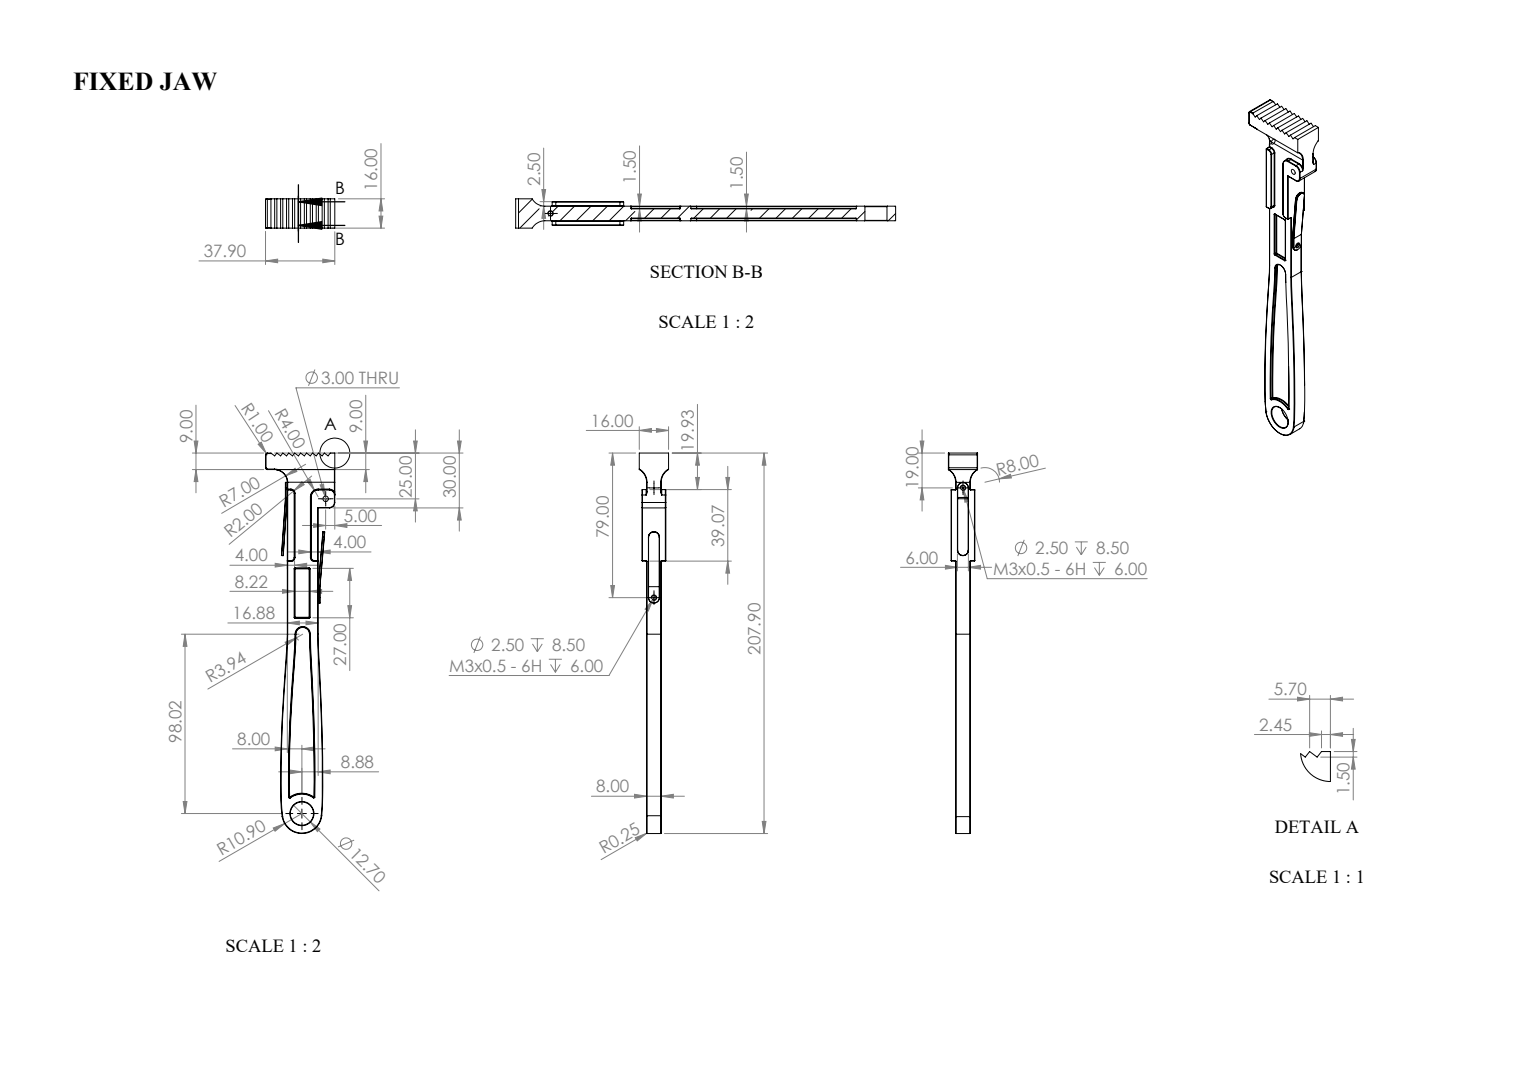
ISO-10303-21;
HEADER;
FILE_DESCRIPTION (('STEP AP214'),
    '1' );
FILE_NAME ('1.0 Fixed Jaw.step',
    '2026-10-07T05:30:18',
    ( '' ),
    ( '' ),
    'SwSTEP 2.0',
    'SolidWorks 2021',
    '' );
FILE_SCHEMA (( 'AUTOMOTIVE_DESIGN' ));
ENDSEC;

DATA;
#30=AXIS2_PLACEMENT_3D ( 'NONE', #64343, #43811, #52312 ) ;
#52=LINE ( 'NONE', #39009, #8257 ) ;
#64=EDGE_CURVE ( 'NONE', #6847, #38896, #39743, .T. ) ;
#74=SURFACE_SIDE_STYLE ('',( #68542 ) ) ;
#87=CARTESIAN_POINT ( 'NONE',  ( -6.000000000000014211, 80.32179676972448590, -4.250000000000000000 ) ) ;
#88=( GEOMETRIC_REPRESENTATION_CONTEXT ( 3 ) GLOBAL_UNCERTAINTY_ASSIGNED_CONTEXT ( ( #83266 ) ) GLOBAL_UNIT_ASSIGNED_CONTEXT ( ( #85236, #77227, #46251 ) ) REPRESENTATION_CONTEXT ( 'NONE', 'WORKASPACE' ) );
#90=EDGE_LOOP ( 'NONE', ( #14273, #19404, #8393, #55652 ) ) ;
#99=DIRECTION ( 'NONE',  ( -0.000000000000000000, -0.000000000000000000, -1.000000000000000000 ) ) ;
#104=CARTESIAN_POINT ( 'NONE',  ( 11.15633734009358058, -69.21829398631774666, 4.000000000000000888 ) ) ;
#105=VERTEX_POINT ( 'NONE', #92727 ) ;
#109=FILL_AREA_STYLE_COLOUR ( '', #46180 ) ;
#111=DIRECTION ( 'NONE',  ( 1.000000000000000000, -0.000000000000000000, -0.000000000000000000 ) ) ;
#123=FILL_AREA_STYLE ('',( #74603 ) ) ;
#124=STYLED_ITEM ( 'NONE', ( #39195 ), #78361 ) ;
#133=CARTESIAN_POINT ( 'NONE',  ( -5.812563760649267941, -35.09659463721938977, -3.750000000000000000 ) ) ;
#148=CIRCLE ( 'NONE', #91104, 1.249999999999987121 ) ;
#175=CARTESIAN_POINT ( 'NONE',  ( -11.62817260212919024, -77.84151128241038009, 3.750000000000000000 ) ) ;
#185=ORIENTED_EDGE ( 'NONE', *, *, #34928, .T. ) ;
#195=DIRECTION ( 'NONE',  ( -1.483861936729427615E-16, 1.000000000000000000, -0.000000000000000000 ) ) ;
#196=DIRECTION ( 'NONE',  ( 0.000000000000000000, 0.000000000000000000, 1.000000000000000000 ) ) ;
#199=ORIENTED_EDGE ( 'NONE', *, *, #97123, .F. ) ;
#201=ORIENTED_EDGE ( 'NONE', *, *, #76299, .T. ) ;
#210=CARTESIAN_POINT ( 'NONE',  ( -6.874984555098656358, -78.81798443069058635, 2.499999999999998224 ) ) ;
#225=STYLED_ITEM ( 'NONE', ( #36779 ), #46100 ) ;
#228=ORIENTED_EDGE ( 'NONE', *, *, #21710, .F. ) ;
#250=SURFACE_STYLE_USAGE ( .BOTH. , #76223 ) ;
#258=FACE_OUTER_BOUND ( 'NONE', #51924, .T. ) ;
#268=AXIS2_PLACEMENT_3D ( 'NONE', #55440, #85944, #96401 ) ;
#274=DIRECTION ( 'NONE',  ( -1.000000000000000000, -0.000000000000000000, -0.000000000000000000 ) ) ;
#281=CARTESIAN_POINT ( 'NONE',  ( 11.13643110622481203, -94.02619357113461263, -3.750000000000000000 ) ) ;
#286=LINE ( 'NONE', #30732, #94331 ) ;
#293=UNCERTAINTY_MEASURE_WITH_UNIT (LENGTH_MEASURE( 1.000000000000000082E-05 ), #85346, 'distance_accuracy_value', 'NONE');
#298=DIRECTION ( 'NONE',  ( 0.000000000000000000, 0.000000000000000000, -1.000000000000000000 ) ) ;
#308=VECTOR ( 'NONE', #84981, 1000.000000000000000 ) ;
#309=( NAMED_UNIT ( * ) SI_UNIT ( $, .STERADIAN. ) SOLID_ANGLE_UNIT ( ) );
#313=ORIENTED_EDGE ( 'NONE', *, *, #41696, .F. ) ;
#328=ORIENTED_EDGE ( 'NONE', *, *, #58687, .T. ) ;
#329=DIRECTION ( 'NONE',  ( 0.000000000000000000, 0.000000000000000000, 1.000000000000000000 ) ) ;
#340=VECTOR ( 'NONE', #77735, 1000.000000000000000 ) ;
#351=CARTESIAN_POINT ( 'NONE',  ( 6.574926501674518420, -50.89417846498341902, -3.750000000000001332 ) ) ;
#365=CARTESIAN_POINT ( 'NONE',  ( 4.864310448982641866, -17.52237222630224878, -2.499999999999999112 ) ) ;
#369=CIRCLE ( 'NONE', #57769, 0.2500000000000002220 ) ;
#384=CARTESIAN_POINT ( 'NONE',  ( -8.330963135173325540, -7.272696214946840598, -3.750000000000000000 ) ) ;
#391=CARTESIAN_POINT ( 'NONE',  ( 9.050000000000002487, 99.99999999999998579, 8.000000000000000000 ) ) ;
#398=EDGE_LOOP ( 'NONE', ( #49399, #35064, #25132, #40932 ) ) ;
#400=CARTESIAN_POINT ( 'NONE',  ( -8.081452932468565109, -7.288464344191233124, -3.999999999999999112 ) ) ;
#406=CARTESIAN_POINT ( 'NONE',  ( -18.89999999999999147, 99.74999999999998579, 7.750000000000000000 ) ) ;
#427=EDGE_CURVE ( 'NONE', #16059, #54251, #3743, .T. ) ;
#445=ORIENTED_EDGE ( 'NONE', *, *, #14494, .F. ) ;
#451=CARTESIAN_POINT ( 'NONE',  ( -6.000000000000014211, 79.82179676972448590, 6.500000000000000888 ) ) ;
#464=ORIENTED_EDGE ( 'NONE', *, *, #87707, .F. ) ;
#475=CARTESIAN_POINT ( 'NONE',  ( -0.6999999999999975131, 99.99999999999998579, -8.000000000000000000 ) ) ;
#477=EDGE_LOOP ( 'NONE', ( #2774, #88083, #69231, #10665 ) ) ;
#493=CARTESIAN_POINT ( 'NONE',  ( 6.033511671501928575, -36.04540650299031768, 2.750000000000000444 ) ) ;
#528=ORIENTED_EDGE ( 'NONE', *, *, #21195, .F. ) ;
#538=VERTEX_POINT ( 'NONE', #32791 ) ;
#539=LINE ( 'NONE', #73152, #10187 ) ;
#540=LINE ( 'NONE', #46011, #12696 ) ;
#548=PLANE ( 'NONE',  #17195 ) ;
#554=CARTESIAN_POINT ( 'NONE',  ( -5.580560104534955101, -28.67655754327235584, -4.000000000000000000 ) ) ;
#556=ORIENTED_EDGE ( 'NONE', *, *, #48860, .F. ) ;
#581=AXIS2_PLACEMENT_3D ( 'NONE', #82369, #74368, #90856 ) ;
#595=( GEOMETRIC_REPRESENTATION_CONTEXT ( 3 ) GLOBAL_UNCERTAINTY_ASSIGNED_CONTEXT ( ( #30226 ) ) GLOBAL_UNIT_ASSIGNED_CONTEXT ( ( #63751, #69807, #85295 ) ) REPRESENTATION_CONTEXT ( 'NONE', 'WORKASPACE' ) );
#598=LINE ( 'NONE', #86029, #77826 ) ;
#599=EDGE_CURVE ( 'NONE', #79717, #54884, #31804, .T. ) ;
#601=CARTESIAN_POINT ( 'NONE',  ( 11.08989791451569396, -87.81815274841501662, 4.000000000000000888 ) ) ;
#620=EDGE_CURVE ( 'NONE', #27580, #78252, #34744, .T. ) ;
#654=CYLINDRICAL_SURFACE ( 'NONE', #4662, 2.999999999999999112 ) ;
#655=EDGE_CURVE ( 'NONE', #6373, #42611, #90428, .T. ) ;
#661=FACE_OUTER_BOUND ( 'NONE', #43555, .T. ) ;
#664=ORIENTED_EDGE ( 'NONE', *, *, #80208, .F. ) ;
#669=CARTESIAN_POINT ( 'NONE',  ( -11.60563658634833040, -81.99692803277896758, 4.000000000000001776 ) ) ;
#679=ORIENTED_EDGE ( 'NONE', *, *, #13478, .F. ) ;
#688=CARTESIAN_POINT ( 'NONE',  ( -3.999999999999994671, 43.00000000000000711, 6.500000000000000888 ) ) ;
#692=ORIENTED_EDGE ( 'NONE', *, *, #60606, .T. ) ;
#694=ORIENTED_EDGE ( 'NONE', *, *, #84783, .T. ) ;
#707=AXIS2_PLACEMENT_3D ( 'NONE', #2561, #55539, #79512 ) ;
#710=DIRECTION ( 'NONE',  ( 0.000000000000000000, -0.000000000000000000, -1.000000000000000000 ) ) ;
#715=DIRECTION ( 'NONE',  ( -0.000000000000000000, -0.000000000000000000, 1.000000000000000000 ) ) ;
#717=VERTEX_POINT ( 'NONE', #42770 ) ;
#730=CARTESIAN_POINT ( 'NONE',  ( 6.034042420210333546, -36.05779855178114701, -2.750000000000001332 ) ) ;
#734=EDGE_CURVE ( 'NONE', #717, #9323, #56198, .T. ) ;
#739=DIRECTION ( 'NONE',  ( 0.000000000000000000, 0.000000000000000000, -1.000000000000000000 ) ) ;
#750=CIRCLE ( 'NONE', #66369, 0.1000000000000001166 ) ;
#761=DIRECTION ( 'NONE',  ( 0.000000000000000000, 0.000000000000000000, -1.000000000000000000 ) ) ;
#767=CARTESIAN_POINT ( 'NONE',  ( 10.68823582872827060, -97.11172657260387098, -4.000000000000000000 ) ) ;
#774=PRESENTATION_STYLE_ASSIGNMENT (( #85725 ) ) ;
#776=ADVANCED_FACE ( 'NONE', ( #13253 ), #4285, .T. ) ;
#780=ORIENTED_EDGE ( 'NONE', *, *, #20104, .T. ) ;
#782=DIRECTION ( 'NONE',  ( -0.000000000000000000, 1.000000000000000000, 0.000000000000000000 ) ) ;
#794=CARTESIAN_POINT ( 'NONE',  ( -3.772059543480554389, -0.8421633283343330501, 3.999999999999999112 ) ) ;
#809=ORIENTED_EDGE ( 'NONE', *, *, #74543, .T. ) ;
#814=( LENGTH_UNIT ( ) NAMED_UNIT ( * ) SI_UNIT ( .MILLI., .METRE. ) );
#818=ADVANCED_FACE ( 'NONE', ( #258 ), #67246, .F. ) ;
#823=CARTESIAN_POINT ( 'NONE',  ( -8.000000000000000000, 80.99999999999994316, -1.249999999999987121 ) ) ;
#826=DIRECTION ( 'NONE',  ( 0.6246950475544238435, 0.7808688094430307203, 0.000000000000000000 ) ) ;
#832=CARTESIAN_POINT ( 'NONE',  ( -7.116236337400218659, -80.68324593764592123, -2.750000000000000000 ) ) ;
#835=( NAMED_UNIT ( * ) SI_UNIT ( $, .STERADIAN. ) SOLID_ANGLE_UNIT ( ) );
#843=CARTESIAN_POINT ( 'NONE',  ( 6.685134130357478277, -80.57704203013921074, -2.500000000000000888 ) ) ;
#846=COLOUR_RGB ( '', 0.40784314, 0.44705882, 0.49803922) ;
#847=CARTESIAN_POINT ( 'NONE',  ( 4.471352795670365587, -3.620003340340034015, 2.750000000000000000 ) ) ;
#861=FILL_AREA_STYLE ('',( #14877 ) ) ;
#868=CYLINDRICAL_SURFACE ( 'NONE', #65920, 0.2500000000000002220 ) ;
#869=DIRECTION ( 'NONE',  ( 0.000000000000000000, 0.000000000000000000, -1.000000000000000000 ) ) ;
#875=VERTEX_POINT ( 'NONE', #9203 ) ;
#876=SURFACE_STYLE_FILL_AREA ( #39838 ) ;
#894=AXIS2_PLACEMENT_3D ( 'NONE', #5161, #50153, #35647 ) ;
#896=CARTESIAN_POINT ( 'NONE',  ( -3.750000000000000000, 37.00000000000000000, 2.500000000000000000 ) ) ;
#905=ORIENTED_EDGE ( 'NONE', *, *, #91110, .F. ) ;
#910=VECTOR ( 'NONE', #54975, 1000.000000000000000 ) ;
#913=CARTESIAN_POINT ( 'NONE',  ( 7.155633850256548634, -69.45312897839663435, 4.000000000000000000 ) ) ;
#917=DIRECTION ( 'NONE',  ( -1.000000000000000000, 0.000000000000000000, 0.000000000000000000 ) ) ;
#918=CARTESIAN_POINT ( 'NONE',  ( -6.060849023604187202, -36.09672517615241816, -3.999999999999998224 ) ) ;
#942=EDGE_CURVE ( 'NONE', #49230, #87437, #86679, .T. ) ;
#944=SURFACE_STYLE_USAGE ( .BOTH. , #70415 ) ;
#946=AXIS2_PLACEMENT_3D ( 'NONE', #32170, #55169, #47682 ) ;
#947=DIRECTION ( 'NONE',  ( 0.000000000000000000, 0.000000000000000000, -1.000000000000000000 ) ) ;
#950=CARTESIAN_POINT ( 'NONE',  ( 4.691427381388422191, -2.693150427207434028, -4.000000000000000000 ) ) ;
#955=AXIS2_PLACEMENT_3D ( 'NONE', #88798, #94817, #26320 ) ;
#965=CARTESIAN_POINT ( 'NONE',  ( -13.22845221182699404, 91.00000000000001421, -8.000000000000001776 ) ) ;
#967=CARTESIAN_POINT ( 'NONE',  ( 4.572805492043258369, -6.390838093377243290, 2.750000000000000000 ) ) ;
#970=DIRECTION ( 'NONE',  ( 0.000000000000000000, 0.000000000000000000, -1.000000000000000000 ) ) ;
#976=AXIS2_PLACEMENT_3D ( 'NONE', #83405, #29399, #14927 ) ;
#981=VERTEX_POINT ( 'NONE', #79166 ) ;
#989=CARTESIAN_POINT ( 'NONE',  ( 18.00000000000000711, 77.36170532436575797, 4.193342410628620343 ) ) ;
#991=SURFACE_STYLE_FILL_AREA ( #92941 ) ;
#1003=EDGE_CURVE ( 'NONE', #3599, #65307, #65631, .T. ) ;
#1019=DIRECTION ( 'NONE',  ( 0.000000000000000000, 0.000000000000000000, 1.000000000000000000 ) ) ;
#1028=ORIENTED_EDGE ( 'NONE', *, *, #35765, .F. ) ;
#1050=STYLED_ITEM ( 'NONE', ( #3795 ), #35208 ) ;
#1051=EDGE_CURVE ( 'NONE', #67870, #46091, #81134, .T. ) ;
#1054=AXIS2_PLACEMENT_3D ( 'NONE', #1684, #85651, #92650 ) ;
#1056=EDGE_CURVE ( 'NONE', #28374, #28519, #71675, .T. ) ;
#1060=ORIENTED_EDGE ( 'NONE', *, *, #71039, .T. ) ;
#1066=CARTESIAN_POINT ( 'NONE',  ( 8.629999999999995453, 40.74999999999999289, -3.750000000000000000 ) ) ;
#1069=CARTESIAN_POINT ( 'NONE',  ( 4.879999999999991900, 76.07179676972444327, 6.250000000000000000 ) ) ;
#1080=DIRECTION ( 'NONE',  ( 1.000000000000000000, 0.000000000000000000, 0.000000000000000000 ) ) ;
#1088=( NAMED_UNIT ( * ) PLANE_ANGLE_UNIT ( ) SI_UNIT ( $, .RADIAN. ) );
#1096=DIRECTION ( 'NONE',  ( 0.000000000000000000, 0.000000000000000000, 1.000000000000000000 ) ) ;
#1107=CARTESIAN_POINT ( 'NONE',  ( -0.000000000000000000, 99.99999999999998579, -8.000000000000000000 ) ) ;
#1113=( BOUNDED_SURFACE ( )  B_SPLINE_SURFACE ( 3, 2, ( 
 ( #32802, #48792, #77812 ),
 ( #94787, #11290, #63297 ),
 ( #64765, #79787, #93807 ),
 ( #79300, #24835, #25337 ),
 ( #95277, #55821, #86315 ),
 ( #87283, #17819, #26287 ),
 ( #39830, #48301, #56788 ),
 ( #26780, #57278, #41327 ),
 ( #70336, #1852, #32310 ),
 ( #62815, #93313, #49774 ),
 ( #35263, #97782, #89746 ),
 ( #50260, #96285, #20276 ),
 ( #5774, #66252, #73265 ),
 ( #87772, #58247, #13760 ),
 ( #27764, #20772, #43262 ),
 ( #35763, #67258, #80281 ),
 ( #28755, #65760, #88766 ),
 ( #44247, #58757, #50773 ) ),
 .UNSPECIFIED., .F., .F., .T. ) 
 B_SPLINE_SURFACE_WITH_KNOTS ( ( 4, 2, 2, 2, 2, 2, 2, 2, 4 ),
 ( 3, 3 ),
 ( 0.000000000000000000, 0.001371970262341175176, 0.002743940524682350352, 0.004115910787023525745, 0.005487881049364700704, 0.006859851311705876531, 0.008231821574047051490, 0.009603791836388226449, 0.01097576209872940141 ),
 ( 0.000000000000000000, 1.000000000000000000 ),
 .UNSPECIFIED. ) 
 GEOMETRIC_REPRESENTATION_ITEM ( )  RATIONAL_B_SPLINE_SURFACE ( (
 ( 1.000000000000000000, 0.7071067811865475727, 1.000000000000000000),
 ( 1.000000000000000000, 0.7072982590433614103, 1.000000000000000000),
 ( 1.000000000000000000, 0.7113498972295660971, 1.000000000000000000),
 ( 1.000000000000000000, 0.7257703676791772418, 1.000000000000000000),
 ( 1.000000000000000000, 0.7362840324263598690, 1.000000000000000000),
 ( 1.000000000000000000, 0.7606319170830569965, 1.000000000000000000),
 ( 1.000000000000000000, 0.7745485803766045674, 1.000000000000000000),
 ( 1.000000000000000000, 0.8036690257212466548, 1.000000000000000000),
 ( 1.000000000000000000, 0.8185245023543151754, 1.000000000000000000),
 ( 1.000000000000000000, 0.8475516512717119477, 1.000000000000000000),
 ( 1.000000000000000000, 0.8617420886046736062, 1.000000000000000000),
 ( 1.000000000000000000, 0.8886174597629885596, 1.000000000000000000),
 ( 1.000000000000000000, 0.9010211234293969973, 1.000000000000000000),
 ( 1.000000000000000000, 0.9233336449993967410, 1.000000000000000000),
 ( 1.000000000000000000, 0.9332564696565026630, 1.000000000000000000),
 ( 1.000000000000000000, 0.9500370447730048795, 1.000000000000000000),
 ( 1.000000000000000000, 0.9567390024731449172, 1.000000000000000000),
 ( 1.000000000000000000, 0.9611621933234241189, 1.000000000000000000) ) ) 
 REPRESENTATION_ITEM ( '' )  SURFACE ( )  );
#1117=DIRECTION ( 'NONE',  ( 0.000000000000000000, 0.000000000000000000, -1.000000000000000000 ) ) ;
#1118=SURFACE_SIDE_STYLE ('',( #69107 ) ) ;
#1119=( BOUNDED_SURFACE ( )  B_SPLINE_SURFACE ( 3, 2, ( 
 ( #95548, #95038, #27036 ),
 ( #4558, #57535, #35527 ),
 ( #64531, #96046, #35022 ),
 ( #88032, #19544, #50040 ),
 ( #80543, #49535, #58021 ),
 ( #20031, #57043, #65523 ),
 ( #50533, #81028, #56562 ),
 ( #73515, #19057, #66021 ) ),
 .UNSPECIFIED., .F., .F., .F. ) 
 B_SPLINE_SURFACE_WITH_KNOTS ( ( 4, 2, 2, 4 ),
 ( 3, 3 ),
 ( 0.000000000000000000, 0.0004516266542298884193, 0.0009032533084597768385, 0.001806506616919553677 ),
 ( 0.000000000000000000, 1.000000000000000000 ),
 .UNSPECIFIED. ) 
 GEOMETRIC_REPRESENTATION_ITEM ( )  RATIONAL_B_SPLINE_SURFACE ( (
 ( 1.000000000000000000, 0.7071067811865523467, 1.000000000000000000),
 ( 1.000000000000000000, 0.7557133596825000854, 1.000000000000000000),
 ( 1.000000000000000000, 0.7976722695486582193, 1.000000000000000000),
 ( 1.000000000000000000, 0.8702934545465945693, 1.000000000000000000),
 ( 1.000000000000000000, 0.9009816261290091166, 1.000000000000000000),
 ( 1.000000000000000000, 0.9749059260395099846, 1.000000000000000000),
 ( 1.000000000000000000, 1.000014990204702858, 1.000000000000000000),
 ( 1.000000000000000000, 1.000000000000000000, 1.000000000000000000) ) ) 
 REPRESENTATION_ITEM ( '' )  SURFACE ( )  );
#1129=ORIENTED_EDGE ( 'NONE', *, *, #54416, .T. ) ;
#1142=VECTOR ( 'NONE', #53062, 1000.000000000000000 ) ;
#1153=CARTESIAN_POINT ( 'NONE',  ( -8.218805110796523650, -9.361916056598095892, 4.000000000000000000 ) ) ;
#1168=VERTEX_POINT ( 'NONE', #82619 ) ;
#1173=CYLINDRICAL_SURFACE ( 'NONE', #94987, 0.2500000000000002220 ) ;
#1190=DIRECTION ( 'NONE',  ( -1.257402221000611116E-16, 1.000000000000000000, 0.000000000000000000 ) ) ;
#1201=CARTESIAN_POINT ( 'NONE',  ( 8.955817848695199146, -3.107653060320455296, 3.750000000000000000 ) ) ;
#1209=FACE_BOUND ( 'NONE', #56829, .T. ) ;
#1222=CARTESIAN_POINT ( 'NONE',  ( 4.441302488725088260, -2.692589364072287772, -2.750000000000000444 ) ) ;
#1256=ORIENTED_EDGE ( 'NONE', *, *, #69290, .F. ) ;
#1271=CARTESIAN_POINT ( 'NONE',  ( -7.750000000000000000, 40.99999999999999289, 4.000000000000000000 ) ) ;
#1272=UNCERTAINTY_MEASURE_WITH_UNIT (LENGTH_MEASURE( 1.000000000000000082E-05 ), #83156, 'distance_accuracy_value', 'NONE');
#1273=VECTOR ( 'NONE', #52048, 1000.000000000000114 ) ;
#1283=DIRECTION ( 'NONE',  ( 0.000000000000000000, 0.000000000000000000, -1.000000000000000000 ) ) ;
#1287=CARTESIAN_POINT ( 'NONE',  ( 17.87804611792045151, 78.26090218833458323, 4.039389165979513585 ) ) ;
#1290=( GEOMETRIC_REPRESENTATION_CONTEXT ( 3 ) GLOBAL_UNCERTAINTY_ASSIGNED_CONTEXT ( ( #20152 ) ) GLOBAL_UNIT_ASSIGNED_CONTEXT ( ( #19702, #95707, #27190 ) ) REPRESENTATION_CONTEXT ( 'NONE', 'WORKASPACE' ) );
#1291=CARTESIAN_POINT ( 'NONE',  ( -5.811454672306898495, -36.11427488548738296, 3.750000000000806022 ) ) ;
#1295=AXIS2_PLACEMENT_3D ( 'NONE', #58868, #65872, #97386 ) ;
#1311=ORIENTED_EDGE ( 'NONE', *, *, #12166, .F. ) ;
#1320=CARTESIAN_POINT ( 'NONE',  ( 3.969999999999999751, 10.25000000000000000, 3.750000000000000000 ) ) ;
#1327=CARTESIAN_POINT ( 'NONE',  ( 5.114684334861586024, -17.52319251364448505, -3.750000000000001332 ) ) ;
#1331=CARTESIAN_POINT ( 'NONE',  ( -3.888850692990851954, -8.270209051930519806, -2.750000000000000000 ) ) ;
#1339=CIRCLE ( 'NONE', #14092, 2.000000000000000000 ) ;
#1341=CARTESIAN_POINT ( 'NONE',  ( -7.982674952684395642, 85.82256618331770426, 4.181766378585055399 ) ) ;
#1343=DIRECTION ( 'NONE',  ( 0.9975640502598257520, -0.06975647374410356982, 0.000000000000000000 ) ) ;
#1348=CIRCLE ( 'NONE', #65182, 0.09999999999999982514 ) ;
#1350=( NAMED_UNIT ( * ) PLANE_ANGLE_UNIT ( ) SI_UNIT ( $, .RADIAN. ) );
#1358=CARTESIAN_POINT ( 'NONE',  ( -11.30180206635943030, -57.06075279892166208, -3.750000000000000000 ) ) ;
#1365=( LENGTH_UNIT ( ) NAMED_UNIT ( * ) SI_UNIT ( .MILLI., .METRE. ) );
#1374=CYLINDRICAL_SURFACE ( 'NONE', #18936, 0.09999999999999939493 ) ;
#1381=CYLINDRICAL_SURFACE ( 'NONE', #44974, 0.2500000000000002220 ) ;
#1384=( LENGTH_UNIT ( ) NAMED_UNIT ( * ) SI_UNIT ( .MILLI., .METRE. ) );
#1406=VECTOR ( 'NONE', #82915, 999.9999999999998863 ) ;
#1409=CARTESIAN_POINT ( 'NONE',  ( 7.160361147697994255, -84.29732993326337009, 4.000000000000000000 ) ) ;
#1420=VECTOR ( 'NONE', #20421, 1000.000000000000000 ) ;
#1428=( GEOMETRIC_REPRESENTATION_CONTEXT ( 3 ) GLOBAL_UNCERTAINTY_ASSIGNED_CONTEXT ( ( #50285 ) ) GLOBAL_UNIT_ASSIGNED_CONTEXT ( ( #76156, #96339, #37675 ) ) REPRESENTATION_CONTEXT ( 'NONE', 'WORKASPACE' ) );
#1432=ORIENTED_EDGE ( 'NONE', *, *, #18304, .F. ) ;
#1445=ADVANCED_FACE ( 'NONE', ( #74115 ), #5649, .T. ) ;
#1458=EDGE_CURVE ( 'NONE', #17988, #12785, #62566, .T. ) ;
#1463=CARTESIAN_POINT ( 'NONE',  ( 4.722628015970558479, -9.822377395415374579, -2.750000000000000000 ) ) ;
#1464=CARTESIAN_POINT ( 'NONE',  ( 6.574584770547601487, -50.88238473864188194, 2.499999999996780797 ) ) ;
#1479=DIRECTION ( 'NONE',  ( -0.000000000000000000, 0.000000000000000000, 1.000000000000000000 ) ) ;
#1482=DIRECTION ( 'NONE',  ( 1.000000000000000000, 0.000000000000000000, 0.000000000000000000 ) ) ;
#1484=CARTESIAN_POINT ( 'NONE',  ( 4.441537491767904022, -2.700695904837609351, -3.750000000000000000 ) ) ;
#1486=DIRECTION ( 'NONE',  ( -0.000000000000000000, -1.000000000000000000, 0.000000000000000000 ) ) ;
#1488=DIRECTION ( 'NONE',  ( -0.08715574274765139351, -0.9961946980917461003, 0.000000000000000000 ) ) ;
#1495=CARTESIAN_POINT ( 'NONE',  ( -8.924603092375777535, 75.06466731010172566, 2.900000000000000355 ) ) ;
#1496=ORIENTED_EDGE ( 'NONE', *, *, #26313, .F. ) ;
#1499=EDGE_CURVE ( 'NONE', #12193, #16898, #77086, .T. ) ;
#1502=AXIS2_PLACEMENT_3D ( 'NONE', #92176, #32141, #40157 ) ;
#1505=ADVANCED_FACE ( 'NONE', ( #62072 ), #85088, .T. ) ;
#1536=CARTESIAN_POINT ( 'NONE',  ( -16.60833333333331652, 99.75000000000000000, -8.000000000000000000 ) ) ;
#1542=SPHERICAL_SURFACE ( 'NONE', #10897, 0.2500000000000000000 ) ;
#1544=ADVANCED_FACE ( 'NONE', ( #2108 ), #93563, .F. ) ;
#1559=VERTEX_POINT ( 'NONE', #16596 ) ;
#1583=( LENGTH_UNIT ( ) NAMED_UNIT ( * ) SI_UNIT ( .MILLI., .METRE. ) );
#1614=DIRECTION ( 'NONE',  ( -1.000000000000000000, -2.569960705150826877E-16, 0.000000000000000000 ) ) ;
#1637=CARTESIAN_POINT ( 'NONE',  ( -8.399999999999998579, 98.49999999999998579, -8.000000000000000000 ) ) ;
#1639=CARTESIAN_POINT ( 'NONE',  ( -0.5000000000000073275, 80.99999999999994316, 0.000000000000000000 ) ) ;
#1640=ORIENTED_EDGE ( 'NONE', *, *, #78041, .T. ) ;
#1668=PRESENTATION_STYLE_ASSIGNMENT (( #38659 ) ) ;
#1670=VERTEX_POINT ( 'NONE', #53595 ) ;
#1684=CARTESIAN_POINT ( 'NONE',  ( 0.4400000000000020006, 1.019547802438468986, -3.750000000000000000 ) ) ;
#1686=CARTESIAN_POINT ( 'NONE',  ( -3.627483523208183680, -3.617667194774622619, 2.499999999999597655 ) ) ;
#1690=DIRECTION ( 'NONE',  ( -0.000000000000000000, 0.000000000000000000, 1.000000000000000000 ) ) ;
#1691=DIRECTION ( 'NONE',  ( 1.000000000000000000, 0.000000000000000000, -0.000000000000000000 ) ) ;
#1697=ORIENTED_EDGE ( 'NONE', *, *, #73921, .T. ) ;
#1698=DIRECTION ( 'NONE',  ( 1.000000000000000000, 0.000000000000000000, 0.000000000000000000 ) ) ;
#1704=CARTESIAN_POINT ( 'NONE',  ( 4.656459206268571904, -8.255604869814334279, -2.750000000000000444 ) ) ;
#1713=SURFACE_SIDE_STYLE ('',( #70194 ) ) ;
#1717=FACE_OUTER_BOUND ( 'NONE', #48148, .T. ) ;
#1723=VECTOR ( 'NONE', #88199, 1000.000000000000000 ) ;
#1732=EDGE_CURVE ( 'NONE', #49491, #1559, #46589, .T. ) ;
#1739=CARTESIAN_POINT ( 'NONE',  ( -5.149999999999996803, 98.49999999999998579, -8.525133428036873795 ) ) ;
#1753=DIRECTION ( 'NONE',  ( -0.000000000000000000, -0.000000000000000000, 1.000000000000000000 ) ) ;
#1755=MECHANICAL_DESIGN_GEOMETRIC_PRESENTATION_REPRESENTATION('',(#6507),#67247);
#1758=ORIENTED_EDGE ( 'NONE', *, *, #63670, .F. ) ;
#1760=DIRECTION ( 'NONE',  ( 1.000000000000000000, 0.000000000000000000, 0.000000000000000000 ) ) ;
#1771=CARTESIAN_POINT ( 'NONE',  ( 17.99999999999999645, 78.24875198621454331, 3.965855704038781404 ) ) ;
#1773=EDGE_CURVE ( 'NONE', #35739, #94992, #27891, .T. ) ;
#1784=ORIENTED_EDGE ( 'NONE', *, *, #75473, .F. ) ;
#1785=EDGE_CURVE ( 'NONE', #54884, #35492, #44377, .T. ) ;
#1799=CARTESIAN_POINT ( 'NONE',  ( -0.5000000000000073275, 80.99999999999994316, 0.000000000000000000 ) ) ;
#1805=CARTESIAN_POINT ( 'NONE',  ( -4.249999999999994671, 43.00000000000000000, -6.500000000000000888 ) ) ;
#1819=AXIS2_PLACEMENT_3D ( 'NONE', #37872, #98390, #30336 ) ;
#1820=STYLED_ITEM ( 'NONE', ( #65871 ), #39060 ) ;
#1821=CARTESIAN_POINT ( 'NONE',  ( -8.000000000000000000, 41.24999999999999289, 6.250000000000000000 ) ) ;
#1829=CARTESIAN_POINT ( 'NONE',  ( -10.00219152607943407, 88.91691738930971667, 5.623636179944063507 ) ) ;
#1832=CARTESIAN_POINT ( 'NONE',  ( 5.679566525943226196, -28.64346213806842556, 2.750000000000001332 ) ) ;
#1845=( GEOMETRIC_REPRESENTATION_CONTEXT ( 3 ) GLOBAL_UNCERTAINTY_ASSIGNED_CONTEXT ( ( #55344 ) ) GLOBAL_UNIT_ASSIGNED_CONTEXT ( ( #13017, #80038, #42063 ) ) REPRESENTATION_CONTEXT ( 'NONE', 'WORKASPACE' ) );
#1852=CARTESIAN_POINT ( 'NONE',  ( -9.483770294663381506, 88.32858231846628883, -5.216041430090311515 ) ) ;
#1883=EDGE_CURVE ( 'NONE', #35180, #37045, #27056, .T. ) ;
#1894=ORIENTED_EDGE ( 'NONE', *, *, #66949, .F. ) ;
#1905=DIRECTION ( 'NONE',  ( -0.9961946980917462113, 0.08715574274765114371, 0.000000000000000000 ) ) ;
#1927=MECHANICAL_DESIGN_GEOMETRIC_PRESENTATION_REPRESENTATION('',(#37028),#64114);
#1934=CARTESIAN_POINT ( 'NONE',  ( -8.000000000000003553, -0.02173251731167446035, 3.750000000000001776 ) ) ;
#1936=DIRECTION ( 'NONE',  ( -1.195561081071950118E-14, 8.738726411657103070E-15, 1.000000000000000000 ) ) ;
#1945=CARTESIAN_POINT ( 'NONE',  ( 7.850000000000003197, 98.49999999999998579, -8.525133428036873795 ) ) ;
#1956=CARTESIAN_POINT ( 'NONE',  ( 4.221206346830829403, -3.619822760651511651, 2.500000000000000000 ) ) ;
#1966=EDGE_CURVE ( 'NONE', #30537, #86221, #95700, .T. ) ;
#1967=ORIENTED_EDGE ( 'NONE', *, *, #84025, .F. ) ;
#1978=CARTESIAN_POINT ( 'NONE',  ( 8.629999999999995453, 41.24999999999999289, 4.000000000000000000 ) ) ;
#1982=CARTESIAN_POINT ( 'NONE',  ( 9.050000000000002487, 99.99999999999998579, -8.525133428036873795 ) ) ;
#1993=VECTOR ( 'NONE', #29194, 1000.000000000000000 ) ;
#2000=CARTESIAN_POINT ( 'NONE',  ( -19.89999999999999858, 92.00000000000000000, 8.000000000000000000 ) ) ;
#2004=DIRECTION ( 'NONE',  ( 1.000000000000000000, 0.000000000000000000, 0.000000000000000000 ) ) ;
#2013=ORIENTED_EDGE ( 'NONE', *, *, #91431, .T. ) ;
#2014=MECHANICAL_DESIGN_GEOMETRIC_PRESENTATION_REPRESENTATION('',(#72206),#89765);
#2021=VERTEX_POINT ( 'NONE', #29367 ) ;
#2032=DIRECTION ( 'NONE',  ( 1.000000000000000000, 0.000000000000000000, 0.000000000000000000 ) ) ;
#2060=CARTESIAN_POINT ( 'NONE',  ( 10.58840669699852199, -98.14374106289703548, -4.000000000000000000 ) ) ;
#2067=ORIENTED_EDGE ( 'NONE', *, *, #18669, .T. ) ;
#2069=DIRECTION ( 'NONE',  ( -0.02177529129993028070, -0.9997628902338809853, 0.000000000000000000 ) ) ;
#2081=STYLED_ITEM ( 'NONE', ( #69841 ), #76215 ) ;
#2084=CYLINDRICAL_SURFACE ( 'NONE', #21834, 0.2500000000000002220 ) ;
#2086=CARTESIAN_POINT ( 'NONE',  ( -18.89999999999999147, 91.25000000000000000, -7.750000000000000000 ) ) ;
#2097=CARTESIAN_POINT ( 'NONE',  ( -11.12340613366069419, 89.95527085539235657, 6.571742733942877557 ) ) ;
#2108=FACE_OUTER_BOUND ( 'NONE', #53525, .T. ) ;
#2109=CARTESIAN_POINT ( 'NONE',  ( -10.82635109560346898, -96.00292546281778527, 4.000000000000000000 ) ) ;
#2112=VECTOR ( 'NONE', #8669, 1000.000000000000000 ) ;
#2119=CARTESIAN_POINT ( 'NONE',  ( -10.29278075765157041, 44.03034551814236153, 0.000000000000000000 ) ) ;
#2120=PRESENTATION_STYLE_ASSIGNMENT (( #63075 ) ) ;
#2137=VERTEX_POINT ( 'NONE', #75867 ) ;
#2151=AXIS2_PLACEMENT_3D ( 'NONE', #93067, #16594, #33053 ) ;
#2157=CIRCLE ( 'NONE', #43652, 0.2500000000000002220 ) ;
#2172=ORIENTED_EDGE ( 'NONE', *, *, #90944, .T. ) ;
#2182=DIRECTION ( 'NONE',  ( 1.000000000000000000, 0.000000000000000000, 0.000000000000000000 ) ) ;
#2183=VERTEX_POINT ( 'NONE', #61837 ) ;
#2184=PRESENTATION_STYLE_ASSIGNMENT (( #40654 ) ) ;
#2189=DIRECTION ( 'NONE',  ( -0.000000000000000000, 1.000000000000000000, -0.000000000000000000 ) ) ;
#2195=DIRECTION ( 'NONE',  ( -0.000000000000000000, -0.000000000000000000, -1.000000000000000000 ) ) ;
#2202=VECTOR ( 'NONE', #88898, 1000.000000000000000 ) ;
#2203=VERTEX_POINT ( 'NONE', #90356 ) ;
#2208=EDGE_CURVE ( 'NONE', #85540, #47721, #21894, .T. ) ;
#2210=( NAMED_UNIT ( * ) SI_UNIT ( $, .STERADIAN. ) SOLID_ANGLE_UNIT ( ) );
#2219=( NAMED_UNIT ( * ) SI_UNIT ( $, .STERADIAN. ) SOLID_ANGLE_UNIT ( ) );
#2237=ORIENTED_EDGE ( 'NONE', *, *, #87940, .T. ) ;
#2249=DIRECTION ( 'NONE',  ( 0.000000000000000000, 0.000000000000000000, -1.000000000000000000 ) ) ;
#2250=UNCERTAINTY_MEASURE_WITH_UNIT (LENGTH_MEASURE( 1.000000000000000082E-05 ), #55656, 'distance_accuracy_value', 'NONE');
#2256=SURFACE_STYLE_USAGE ( .BOTH. , #71710 ) ;
#2270=CARTESIAN_POINT ( 'NONE',  ( -7.322357042924514836, -84.41015717759208314, 4.000000000000000000 ) ) ;
#2287=TOROIDAL_SURFACE ( 'NONE', #83696, 1.750000000000000888, 0.2500000000000000000 ) ;
#2291=CARTESIAN_POINT ( 'NONE',  ( -7.750000000000000000, 41.24999999999999289, 6.500000000000000888 ) ) ;
#2294=EDGE_CURVE ( 'NONE', #83598, #13947, #39853, .T. ) ;
#2297=ORIENTED_EDGE ( 'NONE', *, *, #87825, .F. ) ;
#2300=CARTESIAN_POINT ( 'NONE',  ( -4.000000000000000000, 9.750000000000000000, 4.000000000000000000 ) ) ;
#2301=EDGE_CURVE ( 'NONE', #15515, #34926, #64283, .T. ) ;
#2313=FACE_OUTER_BOUND ( 'NONE', #27274, .T. ) ;
#2314=CARTESIAN_POINT ( 'NONE',  ( -3.628035103970717934, -3.629433155896151675, -2.750000000000000000 ) ) ;
#2324=CARTESIAN_POINT ( 'NONE',  ( -8.211425130294045971, 85.75922772022539675, 4.168580035010579721 ) ) ;
#2327=( LENGTH_UNIT ( ) NAMED_UNIT ( * ) SI_UNIT ( .MILLI., .METRE. ) );
#2330=DIRECTION ( 'NONE',  ( 0.000000000000000000, 0.000000000000000000, 1.000000000000000000 ) ) ;
#2336=CARTESIAN_POINT ( 'NONE',  ( -16.94999999999999929, 100.0000000000000000, -7.896446609406727823 ) ) ;
#2345=DIRECTION ( 'NONE',  ( -2.107602052970794797E-16, 1.000000000000000000, -0.000000000000000000 ) ) ;
#2347=CARTESIAN_POINT ( 'NONE',  ( -6.000000000000014211, 80.07179676972448590, 4.250000000000000000 ) ) ;
#2348=MECHANICAL_DESIGN_GEOMETRIC_PRESENTATION_REPRESENTATION('',(#80616),#15114);
#2353=EDGE_LOOP ( 'NONE', ( #32746, #47116, #81353, #98167 ) ) ;
#2354=DIRECTION ( 'NONE',  ( -1.000000000000000000, -6.938893903907221278E-15, 6.938893903907221278E-15 ) ) ;
#2360=FACE_OUTER_BOUND ( 'NONE', #47057, .T. ) ;
#2391=VERTEX_POINT ( 'NONE', #62824 ) ;
#2395=ORIENTED_EDGE ( 'NONE', *, *, #42890, .F. ) ;
#2406=EDGE_LOOP ( 'NONE', ( #38789, #68564, #35096, #78633 ) ) ;
#2418=VERTEX_POINT ( 'NONE', #40827 ) ;
#2438=ORIENTED_EDGE ( 'NONE', *, *, #33837, .T. ) ;
#2442=ADVANCED_FACE ( 'NONE', ( #69851 ), #1374, .T. ) ;
#2447=DIRECTION ( 'NONE',  ( -0.000000000000000000, -0.000000000000000000, 1.000000000000000000 ) ) ;
#2455=FACE_OUTER_BOUND ( 'NONE', #69497, .T. ) ;
#2457=ORIENTED_EDGE ( 'NONE', *, *, #89519, .T. ) ;
#2459=CYLINDRICAL_SURFACE ( 'NONE', #92120, 0.2500000000000002220 ) ;
#2467=ORIENTED_EDGE ( 'NONE', *, *, #82546, .F. ) ;
#2471=CARTESIAN_POINT ( 'NONE',  ( -3.250000000000000444, 1.019547802438453887, -2.500000000000000000 ) ) ;
#2478=FACE_OUTER_BOUND ( 'NONE', #29779, .T. ) ;
#2492=LINE ( 'NONE', #40474, #9821 ) ;
#2502=VERTEX_POINT ( 'NONE', #93324 ) ;
#2503=DIRECTION ( 'NONE',  ( -1.000000000000000000, 3.469446951953623261E-15, 0.000000000000000000 ) ) ;
#2504=( LENGTH_UNIT ( ) NAMED_UNIT ( * ) SI_UNIT ( .MILLI., .METRE. ) );
#2523=CARTESIAN_POINT ( 'NONE',  ( -4.000000000000000000, 36.75000000000000000, -3.750000000000000000 ) ) ;
#2542=ADVANCED_FACE ( 'NONE', ( #50268, #80785 ), #49783, .F. ) ;
#2557=COLOUR_RGB ( '', 0.31764706, 0.68627451, 0.89019608) ;
#2559=ORIENTED_EDGE ( 'NONE', *, *, #96342, .T. ) ;
#2561=CARTESIAN_POINT ( 'NONE',  ( 3.969999999999999751, 10.25000000000000000, -2.750000000000000000 ) ) ;
#2563=ORIENTED_EDGE ( 'NONE', *, *, #97772, .T. ) ;
#2566=CIRCLE ( 'NONE', #7408, 0.2500000000000002220 ) ;
#2594=LINE ( 'NONE', #48545, #11887 ) ;
#2604=CARTESIAN_POINT ( 'NONE',  ( -7.778993153962144191, -1.060766117554759580, 4.000000000000000000 ) ) ;
#2609=DIRECTION ( 'NONE',  ( 0.8070303256584299145, -0.5905099943842175847, 0.000000000000000000 ) ) ;
#2613=DIRECTION ( 'NONE',  ( 1.000000000000000000, 0.000000000000000000, 0.000000000000000000 ) ) ;
#2626=PRESENTATION_STYLE_ASSIGNMENT (( #71598 ) ) ;
#2630=SPHERICAL_SURFACE ( 'NONE', #35375, 0.2500000000000000000 ) ;
#2631=CARTESIAN_POINT ( 'NONE',  ( -6.599999999999995204, -97.00000000000000000, -4.000000000000000000 ) ) ;
#2633=TOROIDAL_SURFACE ( 'NONE', #15403, 2.750000000000000888, 0.2500000000000000000 ) ;
#2651=CARTESIAN_POINT ( 'NONE',  ( -8.000000000000000000, 40.99999999999999289, -4.250000000000000000 ) ) ;
#2652=ORIENTED_EDGE ( 'NONE', *, *, #42565, .F. ) ;
#2658=CARTESIAN_POINT ( 'NONE',  ( 17.75000000000001776, 4.561680251642721935E-15, 3.750000000000000000 ) ) ;
#2661=EDGE_CURVE ( 'NONE', #59353, #94118, #44470, .T. ) ;
#2673=CIRCLE ( 'NONE', #64922, 0.2500000000000002220 ) ;
#2674=LINE ( 'NONE', #48620, #45796 ) ;
#2678=EDGE_LOOP ( 'NONE', ( #59455, #84303, #7010, #32845 ) ) ;
#2682=EDGE_CURVE ( 'NONE', #16289, #14317, #96295, .T. ) ;
#2691=FACE_OUTER_BOUND ( 'NONE', #12878, .T. ) ;
#2695=FILL_AREA_STYLE_COLOUR ( '', #96755 ) ;
#2698=AXIS2_PLACEMENT_3D ( 'NONE', #72238, #18272, #9785 ) ;
#2708=DIRECTION ( 'NONE',  ( -0.000000000000000000, -0.000000000000000000, 1.000000000000000000 ) ) ;
#2733=CARTESIAN_POINT ( 'NONE',  ( 8.742108547319491052, -4.148811688989288982, -4.000000000000000000 ) ) ;
#2746=ORIENTED_EDGE ( 'NONE', *, *, #3662, .F. ) ;
#2764=CARTESIAN_POINT ( 'NONE',  ( -5.070949216137130122, -24.98410106516922013, 3.999999999995160316 ) ) ;
#2773=CARTESIAN_POINT ( 'NONE',  ( -15.00000000000000000, 83.99999999999998579, -8.000000000000000000 ) ) ;
#2774=ORIENTED_EDGE ( 'NONE', *, *, #75792, .F. ) ;
#2776=ADVANCED_FACE ( 'NONE', ( #42297 ), #92491, .T. ) ;
#2781=ORIENTED_EDGE ( 'NONE', *, *, #92714, .T. ) ;
#2785=AXIS2_PLACEMENT_3D ( 'NONE', #79007, #94012, #16555 ) ;
#2788=CARTESIAN_POINT ( 'NONE',  ( 0.000000000000000000, -97.00000000000000000, -3.750000000000000000 ) ) ;
#2792=CIRCLE ( 'NONE', #5982, 2.250000000000001332 ) ;
#2794=DIRECTION ( 'NONE',  ( 0.000000000000000000, -0.000000000000000000, -1.000000000000000000 ) ) ;
#2799=DIRECTION ( 'NONE',  ( -0.6038238647436497963, 0.7971177707001910751, 1.214306433183775537E-14 ) ) ;
#2806=PRESENTATION_STYLE_ASSIGNMENT (( #71283 ) ) ;
#2835=CARTESIAN_POINT ( 'NONE',  ( -9.000000000000001776, 80.99999999999994316, 2.900000000000000355 ) ) ;
#2836=( NAMED_UNIT ( * ) PLANE_ANGLE_UNIT ( ) SI_UNIT ( $, .RADIAN. ) );
#2845=ORIENTED_EDGE ( 'NONE', *, *, #14494, .T. ) ;
#2853=DIRECTION ( 'NONE',  ( -0.000000000000000000, -1.000000000000000000, -0.000000000000000000 ) ) ;
#2855=SURFACE_STYLE_USAGE ( .BOTH. , #48318 ) ;
#2859=AXIS2_PLACEMENT_3D ( 'NONE', #20883, #73870, #34882 ) ;
#2879=ORIENTED_EDGE ( 'NONE', *, *, #62271, .F. ) ;
#2891=EDGE_CURVE ( 'NONE', #49181, #13782, #9431, .T. ) ;
#2899=EDGE_LOOP ( 'NONE', ( #31606, #88580, #57841, #77361 ) ) ;
#2913=AXIS2_PLACEMENT_3D ( 'NONE', #54169, #93154, #31664 ) ;
#2918=CARTESIAN_POINT ( 'NONE',  ( -10.57641974390271322, -40.47698476369465936, 3.750000000000000000 ) ) ;
#2921=CARTESIAN_POINT ( 'NONE',  ( 10.58840669699852199, -98.14374106289703548, 3.750000000000000000 ) ) ;
#2948=CARTESIAN_POINT ( 'NONE',  ( 9.210000967481738243, -9.315410972688546565, 3.750000000000001776 ) ) ;
#2956=CARTESIAN_POINT ( 'NONE',  ( -5.780406540405962801, -39.80436905996668884, -2.500000000000000000 ) ) ;
#2960=DIRECTION ( 'NONE',  ( 1.000000000000000000, 0.000000000000000000, 0.000000000000000000 ) ) ;
#2962=CARTESIAN_POINT ( 'NONE',  ( 4.380000000000000782, 1.019547802438464545, -3.750000000000000000 ) ) ;
#2986=EDGE_LOOP ( 'NONE', ( #97343, #61026, #74294, #78162 ) ) ;
#2998=STYLED_ITEM ( 'NONE', ( #39152 ), #60167 ) ;
#3000=LINE ( 'NONE', #17985, #910 ) ;
#3018=MECHANICAL_DESIGN_GEOMETRIC_PRESENTATION_REPRESENTATION('',(#19187),#95778);
#3050=AXIS2_PLACEMENT_3D ( 'NONE', #50301, #35303, #59289 ) ;
#3055=ORIENTED_EDGE ( 'NONE', *, *, #7259, .F. ) ;
#3080=SURFACE_STYLE_FILL_AREA ( #71568 ) ;
#3083=STYLED_ITEM ( 'NONE', ( #24289 ), #26841 ) ;
#3084=CARTESIAN_POINT ( 'NONE',  ( -10.60846762071325067, -98.07569628617517310, 3.999999999999999112 ) ) ;
#3088=CARTESIAN_POINT ( 'NONE',  ( 4.219999999999999751, 10.25000000000000000, -2.500000000000000000 ) ) ;
#3090=DIRECTION ( 'NONE',  ( 0.000000000000000000, 0.000000000000000000, -1.000000000000000000 ) ) ;
#3096=CARTESIAN_POINT ( 'NONE',  ( -5.810050997930829908, -36.09132698039145737, -3.750000000000001332 ) ) ;
#3097=FILL_AREA_STYLE ('',( #78087 ) ) ;
#3118=CARTESIAN_POINT ( 'NONE',  ( -13.77308431840578962, 90.93904485323390929, 7.896207356394697285 ) ) ;
#3119=DIRECTION ( 'NONE',  ( -0.9975640502598243087, 0.06975647374412544122, 0.000000000000000000 ) ) ;
#3128=ORIENTED_EDGE ( 'NONE', *, *, #56101, .T. ) ;
#3135=ORIENTED_EDGE ( 'NONE', *, *, #5338, .T. ) ;
#3137=EDGE_LOOP ( 'NONE', ( #4836, #41624, #56935 ) ) ;
#3149=CARTESIAN_POINT ( 'NONE',  ( 11.08989791444925288, -87.81815274839443930, 4.000000000000000000 ) ) ;
#3154=AXIS2_PLACEMENT_3D ( 'NONE', #28845, #89363, #34874 ) ;
#3155=CARTESIAN_POINT ( 'NONE',  ( -15.00000000000000000, 83.99999999999998579, -7.750000000000000000 ) ) ;
#3161=DIRECTION ( 'NONE',  ( 0.000000000000000000, -0.000000000000000000, 1.000000000000000000 ) ) ;
#3163=( NAMED_UNIT ( * ) PLANE_ANGLE_UNIT ( ) SI_UNIT ( $, .RADIAN. ) );
#3169=EDGE_CURVE ( 'NONE', #15638, #25872, #6220, .T. ) ;
#3183=CARTESIAN_POINT ( 'NONE',  ( -8.159336008804556784, -4.163137246816088322, -4.000000000000000000 ) ) ;
#3185=CARTESIAN_POINT ( 'NONE',  ( -0.000000000000000000, 40.74999999999999289, -4.000000000000000000 ) ) ;
#3199=CARTESIAN_POINT ( 'NONE',  ( -6.000000000000000000, 78.07179676972447169, 4.250000000000000000 ) ) ;
#3201=UNCERTAINTY_MEASURE_WITH_UNIT (LENGTH_MEASURE( 1.000000000000000082E-05 ), #69237, 'distance_accuracy_value', 'NONE');
#3205=ORIENTED_EDGE ( 'NONE', *, *, #62192, .F. ) ;
#3206=CARTESIAN_POINT ( 'NONE',  ( 8.650319761818652253, -1.048872767148395280, -4.000000000000000000 ) ) ;
#3207=CARTESIAN_POINT ( 'NONE',  ( 4.722628015970558479, -9.822377395415374579, 3.750000000000001776 ) ) ;
#3214=CARTESIAN_POINT ( 'NONE',  ( 3.969999999999999751, 10.25000000000000000, -2.750000000000000000 ) ) ;
#3217=SURFACE_STYLE_FILL_AREA ( #10226 ) ;
#3219=ORIENTED_EDGE ( 'NONE', *, *, #36268, .F. ) ;
#3233=CARTESIAN_POINT ( 'NONE',  ( -5.580560104534956878, -28.67655754325946660, 4.000000000000000000 ) ) ;
#3243=EDGE_CURVE ( 'NONE', #13782, #81929, #70748, .T. ) ;
#3250=ORIENTED_EDGE ( 'NONE', *, *, #3662, .T. ) ;
#3258=VECTOR ( 'NONE', #11309, 999.9999999999998863 ) ;
#3267=VECTOR ( 'NONE', #90993, 1000.000000000000000 ) ;
#3293=VECTOR ( 'NONE', #33651, 1000.000000000000000 ) ;
#3294=DIRECTION ( 'NONE',  ( 0.000000000000000000, 1.000000000000000000, 0.000000000000000000 ) ) ;
#3297=DIRECTION ( 'NONE',  ( 0.000000000000000000, -1.000000000000000000, 0.000000000000000000 ) ) ;
#3300=CARTESIAN_POINT ( 'NONE',  ( -0.5000000000000073275, 80.99999999999994316, 0.000000000000000000 ) ) ;
#3301=ORIENTED_EDGE ( 'NONE', *, *, #37855, .F. ) ;
#3320=CARTESIAN_POINT ( 'NONE',  ( 11.10647200087811548, -65.08385396171316017, -3.999999999999999112 ) ) ;
#3325=CARTESIAN_POINT ( 'NONE',  ( 14.35000000000000142, 98.49999999999998579, 8.000000000000000000 ) ) ;
#3331=UNCERTAINTY_MEASURE_WITH_UNIT (LENGTH_MEASURE( 1.000000000000000082E-05 ), #72088, 'distance_accuracy_value', 'NONE');
#3349=ORIENTED_EDGE ( 'NONE', *, *, #80392, .T. ) ;
#3365=ORIENTED_EDGE ( 'NONE', *, *, #44520, .F. ) ;
#3379=VERTEX_POINT ( 'NONE', #90619 ) ;
#3387=CARTESIAN_POINT ( 'NONE',  ( -11.19909113571437764, -94.48345865769024954, 3.750000000000001776 ) ) ;
#3391=DIRECTION ( 'NONE',  ( -1.000000000000000000, 0.000000000000000000, 0.000000000000000000 ) ) ;
#3395=( LENGTH_UNIT ( ) NAMED_UNIT ( * ) SI_UNIT ( .MILLI., .METRE. ) );
#3398=ORIENTED_EDGE ( 'NONE', *, *, #43235, .F. ) ;
#3401=DIRECTION ( 'NONE',  ( 0.000000000000000000, 0.000000000000000000, 1.000000000000000000 ) ) ;
#3409=ORIENTED_EDGE ( 'NONE', *, *, #87810, .F. ) ;
#3410=VECTOR ( 'NONE', #96554, 1000.000000000000000 ) ;
#3411=CARTESIAN_POINT ( 'NONE',  ( 11.34661744925197624, 54.08985607419765529, -3.000000000000000000 ) ) ;
#3419=DIRECTION ( 'NONE',  ( -1.000000000000000000, 0.000000000000000000, 0.000000000000000000 ) ) ;
#3424=CARTESIAN_POINT ( 'NONE',  ( 8.992322367875814848, -4.150253140106991090, 3.750000000000001332 ) ) ;
#3431=ADVANCED_FACE ( 'NONE', ( #15642 ), #28642, .F. ) ;
#3434=CARTESIAN_POINT ( 'NONE',  ( -3.585386599411524156, -2.690194976751732359, -2.500000000000604405 ) ) ;
#3440=EDGE_CURVE ( 'NONE', #94114, #26872, #52627, .T. ) ;
#3441=CARTESIAN_POINT ( 'NONE',  ( 4.906778809679744668, -8.256987753881587011, -4.000000000000000000 ) ) ;
#3443=PLANE ( 'NONE',  #6944 ) ;
#3444=CARTESIAN_POINT ( 'NONE',  ( -4.139423687100486582, -8.271184049145468009, 3.999999999999999112 ) ) ;
#3447=DIRECTION ( 'NONE',  ( 0.000000000000000000, 0.000000000000000000, -1.000000000000000000 ) ) ;
#3458=UNCERTAINTY_MEASURE_WITH_UNIT (LENGTH_MEASURE( 1.000000000000000082E-05 ), #32392, 'distance_accuracy_value', 'NONE');
#3465=DIRECTION ( 'NONE',  ( -0.9961946980917462113, 0.08715574274765114371, 0.000000000000000000 ) ) ;
#3468=FACE_OUTER_BOUND ( 'NONE', #66664, .T. ) ;
#3479=CIRCLE ( 'NONE', #88097, 0.2500000000000002220 ) ;
#3480=EDGE_LOOP ( 'NONE', ( #88404, #88335, #52226, #16128, #25037 ) ) ;
#3491=CARTESIAN_POINT ( 'NONE',  ( -10.79821277343923569, -44.62913131165727521, -3.749999999999999556 ) ) ;
#3496=ORIENTED_EDGE ( 'NONE', *, *, #58377, .T. ) ;
#3497=VECTOR ( 'NONE', #5120, 1000.000000000000000 ) ;
#3523=EDGE_LOOP ( 'NONE', ( #75525, #72701, #98043, #81908 ) ) ;
#3545=EDGE_CURVE ( 'NONE', #2502, #13075, #52604, .T. ) ;
#3567=CARTESIAN_POINT ( 'NONE',  ( -3.250000000000000444, 1.019547802438465656, -2.500000000000000000 ) ) ;
#3574=CARTESIAN_POINT ( 'NONE',  ( -8.218805110708677475, -9.361916056596390590, 4.000000000000000000 ) ) ;
#3576=CIRCLE ( 'NONE', #38757, 0.09999999999999982514 ) ;
#3599=VERTEX_POINT ( 'NONE', #47599 ) ;
#3610=ADVANCED_FACE ( 'NONE', ( #16614 ), #32081, .T. ) ;
#3613=ORIENTED_EDGE ( 'NONE', *, *, #97214, .F. ) ;
#3618=FILL_AREA_STYLE ('',( #18134 ) ) ;
#3619=ADVANCED_FACE ( 'NONE', ( #78588 ), #654, .T. ) ;
#3621=VECTOR ( 'NONE', #34408, 1000.000000000000000 ) ;
#3626=ORIENTED_EDGE ( 'NONE', *, *, #17312, .T. ) ;
#3634=CARTESIAN_POINT ( 'NONE',  ( -4.000000000000000000, 9.750000000000000000, 3.750000000000000000 ) ) ;
#3636=AXIS2_PLACEMENT_3D ( 'NONE', #1639, #80067, #78596 ) ;
#3640=CARTESIAN_POINT ( 'NONE',  ( -7.750355510519348456, 84.07179676972448590, 3.750000000000000000 ) ) ;
#3646=CARTESIAN_POINT ( 'NONE',  ( 0.000000000000000000, 91.00000000000000000, -8.000000000000000000 ) ) ;
#3655=CARTESIAN_POINT ( 'NONE',  ( 10.83696084481538691, -98.17058944465519232, -3.750000000000001776 ) ) ;
#3658=( NAMED_UNIT ( * ) PLANE_ANGLE_UNIT ( ) SI_UNIT ( $, .RADIAN. ) );
#3662=EDGE_CURVE ( 'NONE', #79731, #25163, #48380, .T. ) ;
#3670=DIRECTION ( 'NONE',  ( 0.000000000000000000, -0.000000000000000000, -1.000000000000000000 ) ) ;
#3672=DIRECTION ( 'NONE',  ( -0.08715574274765140739, -0.9961946980917462113, 0.000000000000000000 ) ) ;
#3678=CARTESIAN_POINT ( 'NONE',  ( -11.62646502377548607, -81.99905065409454608, -3.750000000000000000 ) ) ;
#3684=STYLED_ITEM ( 'NONE', ( #40350 ), #65927 ) ;
#3699=( GEOMETRIC_REPRESENTATION_CONTEXT ( 3 ) GLOBAL_UNCERTAINTY_ASSIGNED_CONTEXT ( ( #59462 ) ) GLOBAL_UNIT_ASSIGNED_CONTEXT ( ( #69104, #98138, #6134 ) ) REPRESENTATION_CONTEXT ( 'NONE', 'WORKASPACE' ) );
#3701=CARTESIAN_POINT ( 'NONE',  ( 5.510795456469524289, -25.29786701974074603, 2.750000000000000000 ) ) ;
#3712=PLANE ( 'NONE',  #75430 ) ;
#3713=VERTEX_POINT ( 'NONE', #9103 ) ;
#3721=( NAMED_UNIT ( * ) SI_UNIT ( $, .STERADIAN. ) SOLID_ANGLE_UNIT ( ) );
#3735=ORIENTED_EDGE ( 'NONE', *, *, #87534, .F. ) ;
#3743=( BOUNDED_CURVE ( )  B_SPLINE_CURVE ( 3, ( #84826, #93302, #2336, #93795 ),
 .UNSPECIFIED., .F., .T. ) 
 B_SPLINE_CURVE_WITH_KNOTS ( ( 4, 4 ),
 ( 4.712388980384682569, 6.283185307179586232 ),
 .UNSPECIFIED. ) 
 CURVE ( )  GEOMETRIC_REPRESENTATION_ITEM ( )  RATIONAL_B_SPLINE_CURVE ( ( 1.000000000000000000, 0.8047378541243632721, 0.8047378541243632721, 1.000000000000000000 ) ) 
 REPRESENTATION_ITEM ( '' )  );
#3745=AXIS2_PLACEMENT_3D ( 'NONE', #53930, #8430, #947 ) ;
#3769=SURFACE_STYLE_USAGE ( .BOTH. , #49248 ) ;
#3785=CARTESIAN_POINT ( 'NONE',  ( -11.88867004768947488, 90.28252147127371074, 6.948627224671861669 ) ) ;
#3795=PRESENTATION_STYLE_ASSIGNMENT (( #72749 ) ) ;
#3802=LINE ( 'NONE', #34257, #37806 ) ;
#3806=( NAMED_UNIT ( * ) SI_UNIT ( $, .STERADIAN. ) SOLID_ANGLE_UNIT ( ) );
#3807=FACE_OUTER_BOUND ( 'NONE', #24358, .T. ) ;
#3816=( LENGTH_UNIT ( ) NAMED_UNIT ( * ) SI_UNIT ( .MILLI., .METRE. ) );
#3824=DIRECTION ( 'NONE',  ( 1.000000000000000000, -0.000000000000000000, 0.000000000000000000 ) ) ;
#3825=( NAMED_UNIT ( * ) SI_UNIT ( $, .STERADIAN. ) SOLID_ANGLE_UNIT ( ) );
#3831=AXIS2_PLACEMENT_3D ( 'NONE', #33776, #73273, #4305 ) ;
#3870=DIRECTION ( 'NONE',  ( -1.000000000000000000, -1.927470528863123732E-16, 0.000000000000000000 ) ) ;
#3874=ADVANCED_FACE ( 'NONE', ( #27047 ), #35538, .T. ) ;
#3878=VERTEX_POINT ( 'NONE', #56580 ) ;
#3882=EDGE_LOOP ( 'NONE', ( #36369, #73407, #25454, #32022 ) ) ;
#3887=DIRECTION ( 'NONE',  ( -1.000000000000000000, 0.000000000000000000, 0.000000000000000000 ) ) ;
#3889=FACE_OUTER_BOUND ( 'NONE', #88582, .T. ) ;
#3903=DIRECTION ( 'NONE',  ( 0.08715574274765139351, 0.9961946980917461003, -0.000000000000000000 ) ) ;
#3914=CARTESIAN_POINT ( 'NONE',  ( 11.33945612263218372, -87.84223371190563512, 3.750000000000000000 ) ) ;
#3916=DIRECTION ( 'NONE',  ( 0.6246950475544237324, 0.7808688094430306093, 0.000000000000000000 ) ) ;
#3921=CARTESIAN_POINT ( 'NONE',  ( 17.75000000000000000, 78.32179676972447169, -4.000000000000000000 ) ) ;
#3922=CARTESIAN_POINT ( 'NONE',  ( -3.335599319945496077, -2.700684445898925645, -2.499999999999999112 ) ) ;
#3929=CARTESIAN_POINT ( 'NONE',  ( 7.184035427668765017, -73.16388022040806050, -4.000000000000000000 ) ) ;
#3931=DIRECTION ( 'NONE',  ( -0.000000000000000000, 0.000000000000000000, 1.000000000000000000 ) ) ;
#3932=CARTESIAN_POINT ( 'NONE',  ( -7.374944882893554876, -78.83129233208416053, 4.000000000000000888 ) ) ;
#3939=CARTESIAN_POINT ( 'NONE',  ( -6.000000000000009770, 40.99999999999999289, 6.500000000000000888 ) ) ;
#3941=CARTESIAN_POINT ( 'NONE',  ( -3.750000000000000000, 10.00000000000000000, -2.750000000000000000 ) ) ;
#3966=ORIENTED_EDGE ( 'NONE', *, *, #9045, .F. ) ;
#3970=DIRECTION ( 'NONE',  ( -0.000000000000000000, -0.000000000000000000, 1.000000000000000000 ) ) ;
#3973=TOROIDAL_SURFACE ( 'NONE', #85396, 1.750000000000000888, 0.2500000000000000000 ) ;
#3989=EDGE_CURVE ( 'NONE', #16659, #32093, #30185, .T. ) ;
#4002=DIRECTION ( 'NONE',  ( 0.000000000000000000, 0.000000000000000000, -1.000000000000000000 ) ) ;
#4005=EDGE_CURVE ( 'NONE', #10110, #86010, #76692, .T. ) ;
#4008=CARTESIAN_POINT ( 'NONE',  ( -15.00000000000000000, 83.99999999999998579, -3.750000000000000000 ) ) ;
#4013=AXIS2_PLACEMENT_3D ( 'NONE', #22187, #44675, #76163 ) ;
#4021=EDGE_LOOP ( 'NONE', ( #65373, #62874, #89486, #27328 ) ) ;
#4068=CARTESIAN_POINT ( 'NONE',  ( -3.771300132029604679, -6.411618995301440194, -3.750000000000000888 ) ) ;
#4074=CARTESIAN_POINT ( 'NONE',  ( -18.89999999999999503, 98.99999999999998579, 8.000000000000000000 ) ) ;
#4084=CARTESIAN_POINT ( 'NONE',  ( -3.878348535190609958, -3.630205232350322664, -4.000000000000000000 ) ) ;
#4085=EDGE_CURVE ( 'NONE', #16659, #26486, #41434, .T. ) ;
#4091=CIRCLE ( 'NONE', #55162, 6.349999999999995204 ) ;
#4098=EDGE_CURVE ( 'NONE', #24454, #17231, #14305, .T. ) ;
#4105=ORIENTED_EDGE ( 'NONE', *, *, #89557, .T. ) ;
#4110=DIRECTION ( 'NONE',  ( -1.000000000000000000, 0.000000000000000000, -0.000000000000000000 ) ) ;
#4111=VECTOR ( 'NONE', #3903, 1000.000000000000114 ) ;
#4112=COLOUR_RGB ( '', 0.08235294, 0.09019608, 0.10196078) ;
#4119=EDGE_CURVE ( 'NONE', #86711, #69773, #25442, .T. ) ;
#4125=CARTESIAN_POINT ( 'NONE',  ( 17.97673228209724883, 77.65180420275405027, -4.136168975609629150 ) ) ;
#4128=EDGE_CURVE ( 'NONE', #64978, #53779, #37980, .T. ) ;
#4130=ORIENTED_EDGE ( 'NONE', *, *, #83673, .F. ) ;
#4134=CARTESIAN_POINT ( 'NONE',  ( 10.88666287862788273, -94.01511732728891957, 4.000000000000000000 ) ) ;
#4139=DIRECTION ( 'NONE',  ( 0.6246950475544238435, 0.7808688094430307203, 0.000000000000000000 ) ) ;
#4140=CARTESIAN_POINT ( 'NONE',  ( 11.10000000000000142, 98.49999999999998579, 8.000000000000000000 ) ) ;
#4143=CARTESIAN_POINT ( 'NONE',  ( 0.000000000000000000, -97.00000000000000000, -4.000000000000000000 ) ) ;
#4145=DIRECTION ( 'NONE',  ( -1.049065152435176504E-16, 1.000000000000000000, 0.000000000000000000 ) ) ;
#4181=AXIS2_PLACEMENT_3D ( 'NONE', #14712, #75685, #30172 ) ;
#4182=UNCERTAINTY_MEASURE_WITH_UNIT (LENGTH_MEASURE( 1.000000000000000082E-05 ), #71788, 'distance_accuracy_value', 'NONE');
#4188=CARTESIAN_POINT ( 'NONE',  ( 5.510795456469524289, -25.29786701974074603, 3.750000000000001776 ) ) ;
#4224=ORIENTED_EDGE ( 'NONE', *, *, #3545, .F. ) ;
#4237=ORIENTED_EDGE ( 'NONE', *, *, #53624, .T. ) ;
#4248=CARTESIAN_POINT ( 'NONE',  ( -3.750000000000000000, 9.750000000000000000, -4.000000000000000000 ) ) ;
#4249=B_SPLINE_SURFACE_WITH_KNOTS ( 'NONE', 3, 1, ( 
 ( #17669, #84198 ),
 ( #69192, #48142 ),
 ( #31170, #78656 ),
 ( #40659, #62151 ),
 ( #64115, #11132 ),
 ( #58091, #57115 ),
 ( #19123, #41651 ),
 ( #4632, #18641 ),
 ( #42614, #96121 ),
 ( #48632, #57605 ),
 ( #12601, #5116 ),
 ( #26620, #79135 ),
 ( #49604, #71645 ),
 ( #88106, #11621 ),
 ( #19614, #26141 ),
 ( #50109, #41160 ),
 ( #80619, #12113 ),
 ( #35602, #27604 ) ),
 .UNSPECIFIED., .F., .F., .F.,
 ( 4, 2, 2, 2, 2, 2, 2, 2, 4 ),
 ( 2, 2 ),
 ( 0.000000000000000000, 0.06249999999999988898, 0.1249999999999998890, 0.2499999999999997780, 0.4999999999999994449, 0.5624999999999994449, 0.6249999999999994449, 0.7499999999999995559, 0.8570805329376185444 ),
 ( 0.000000000000000000, 1.000000000000000000 ),
 .UNSPECIFIED. ) ;
#4254=FILL_AREA_STYLE ('',( #96741 ) ) ;
#4270=CARTESIAN_POINT ( 'NONE',  ( -13.83909701985790974, 90.94176541299273708, 7.900788997805663350 ) ) ;
#4272=ORIENTED_EDGE ( 'NONE', *, *, #60871, .F. ) ;
#4274=LINE ( 'NONE', #19264, #7402 ) ;
#4285=CYLINDRICAL_SURFACE ( 'NONE', #66457, 3.000000000000000888 ) ;
#4286=FILL_AREA_STYLE ('',( #36253 ) ) ;
#4292=CARTESIAN_POINT ( 'NONE',  ( -5.329507111614364412, -28.66964109972052199, 2.750000000000000444 ) ) ;
#4305=DIRECTION ( 'NONE',  ( 0.000000000000000000, 0.000000000000000000, 1.000000000000000000 ) ) ;
#4312=CARTESIAN_POINT ( 'NONE',  ( 8.959589291341636397, -9.312544548371912256, -4.000000000000000000 ) ) ;
#4314=( NAMED_UNIT ( * ) PLANE_ANGLE_UNIT ( ) SI_UNIT ( $, .RADIAN. ) );
#4315=FACE_OUTER_BOUND ( 'NONE', #2899, .T. ) ;
#4322=VERTEX_POINT ( 'NONE', #12378 ) ;
#4329=CARTESIAN_POINT ( 'NONE',  ( 0.000000000000000000, -97.00000000000000000, 2.500000000000000000 ) ) ;
#4330=CIRCLE ( 'NONE', #17105, 0.2500000000000002220 ) ;
#4384=FILL_AREA_STYLE_COLOUR ( '', #53679 ) ;
#4387=DIRECTION ( 'NONE',  ( 0.000000000000000000, 0.000000000000000000, 1.000000000000000000 ) ) ;
#4393=SURFACE_SIDE_STYLE ('',( #29327 ) ) ;
#4396=CARTESIAN_POINT ( 'NONE',  ( -8.000000000000000000, 41.24999999999999289, 4.250000000000000000 ) ) ;
#4400=CARTESIAN_POINT ( 'NONE',  ( -6.000000000000014211, 80.32179676972448590, 4.250000000000000000 ) ) ;
#4402=LINE ( 'NONE', #58348, #7220 ) ;
#4405=CIRCLE ( 'NONE', #60277, 2.900000000000001243 ) ;
#4410=CARTESIAN_POINT ( 'NONE',  ( 6.910443788711833513, -84.29081344372315243, 2.750000000004829026 ) ) ;
#4412=ORIENTED_EDGE ( 'NONE', *, *, #10740, .T. ) ;
#4423=PRESENTATION_STYLE_ASSIGNMENT (( #41932 ) ) ;
#4431=CARTESIAN_POINT ( 'NONE',  ( 4.471658927061713307, -3.629165645961075715, -3.750000000000000000 ) ) ;
#4437=FACE_OUTER_BOUND ( 'NONE', #25861, .T. ) ;
#4444=LINE ( 'NONE', #42919, #74822 ) ;
#4470=DIRECTION ( 'NONE',  ( -1.049065152435176504E-16, 1.000000000000000000, -0.000000000000000000 ) ) ;
#4480=AXIS2_PLACEMENT_3D ( 'NONE', #16144, #46630, #9629 ) ;
#4481=ADVANCED_FACE ( 'NONE', ( #95898 ), #81366, .F. ) ;
#4489=VECTOR ( 'NONE', #80525, 1000.000000000000000 ) ;
#4491=TOROIDAL_SURFACE ( 'NONE', #33230, 10.65000000000000036, 0.2500000000000000000 ) ;
#4510=CARTESIAN_POINT ( 'NONE',  ( 6.284496703633148051, -36.06254290988038491, 3.999999999999999112 ) ) ;
#4523=CARTESIAN_POINT ( 'NONE',  ( 6.937721053838227014, -80.66520463107747219, -3.750000000000000888 ) ) ;
#4539=ADVANCED_FACE ( 'NONE', ( #67355 ), #72872, .F. ) ;
#4551=TOROIDAL_SURFACE ( 'NONE', #7775, 6.599999999999995204, 0.2500000000000000000 ) ;
#4554=AXIS2_PLACEMENT_3D ( 'NONE', #69033, #70018, #85508 ) ;
#4558=CARTESIAN_POINT ( 'NONE',  ( 18.00000000000000000, 78.65120189252257887, -3.750000044091261309 ) ) ;
#4565=SURFACE_STYLE_USAGE ( .BOTH. , #20038 ) ;
#4582=CARTESIAN_POINT ( 'NONE',  ( -3.586264863028716388, -2.711807932117549225, -4.000000000000000000 ) ) ;
#4589=FACE_OUTER_BOUND ( 'NONE', #98723, .T. ) ;
#4598=DIRECTION ( 'NONE',  ( -0.000000000000000000, -0.000000000000000000, -1.000000000000000000 ) ) ;
#4601=( NAMED_UNIT ( * ) SI_UNIT ( $, .STERADIAN. ) SOLID_ANGLE_UNIT ( ) );
#4602=ORIENTED_EDGE ( 'NONE', *, *, #50023, .F. ) ;
#4608=( LENGTH_UNIT ( ) NAMED_UNIT ( * ) SI_UNIT ( .MILLI., .METRE. ) );
#4619=( GEOMETRIC_REPRESENTATION_CONTEXT ( 3 ) GLOBAL_UNCERTAINTY_ASSIGNED_CONTEXT ( ( #16234 ) ) GLOBAL_UNIT_ASSIGNED_CONTEXT ( ( #80918, #73400, #81402 ) ) REPRESENTATION_CONTEXT ( 'NONE', 'WORKASPACE' ) );
#4624=STYLED_ITEM ( 'NONE', ( #8786 ), #71604 ) ;
#4632=CARTESIAN_POINT ( 'NONE',  ( -5.112373461513591621, -25.53775085953292390, 2.750000000000000000 ) ) ;
#4634=CARTESIAN_POINT ( 'NONE',  ( 8.880000000000020322, 79.82179676972448590, -6.250000000000000000 ) ) ;
#4645=( GEOMETRIC_REPRESENTATION_CONTEXT ( 3 ) GLOBAL_UNCERTAINTY_ASSIGNED_CONTEXT ( ( #48187 ) ) GLOBAL_UNIT_ASSIGNED_CONTEXT ( ( #24067, #98612, #67594 ) ) REPRESENTATION_CONTEXT ( 'NONE', 'WORKASPACE' ) );
#4647=ADVANCED_FACE ( 'NONE', ( #30824 ), #22856, .T. ) ;
#4652=EDGE_CURVE ( 'NONE', #5883, #49695, #54310, .T. ) ;
#4661=( NAMED_UNIT ( * ) SI_UNIT ( $, .STERADIAN. ) SOLID_ANGLE_UNIT ( ) );
#4662=AXIS2_PLACEMENT_3D ( 'NONE', #16118, #55599, #77587 ) ;
#4668=CARTESIAN_POINT ( 'NONE',  ( -11.63911236827289919, -77.84336773400825393, -3.999999999996396216 ) ) ;
#4669=APPLICATION_CONTEXT ( 'automotive_design' ) ;
#4684=ADVANCED_FACE ( 'NONE', ( #83837 ), #15847, .F. ) ;
#4686=CARTESIAN_POINT ( 'NONE',  ( 6.732888861736110009, -58.30752899003807954, 2.750000000000000000 ) ) ;
#4689=( GEOMETRIC_REPRESENTATION_CONTEXT ( 3 ) GLOBAL_UNCERTAINTY_ASSIGNED_CONTEXT ( ( #64161 ) ) GLOBAL_UNIT_ASSIGNED_CONTEXT ( ( #36300, #4828, #51301 ) ) REPRESENTATION_CONTEXT ( 'NONE', 'WORKASPACE' ) );
#4698=DIRECTION ( 'NONE',  ( 1.000000000000000000, 0.000000000000000000, 0.000000000000000000 ) ) ;
#4709=FILL_AREA_STYLE ('',( #82655 ) ) ;
#4716=CARTESIAN_POINT ( 'NONE',  ( -10.77730536144846596, -98.63085534186639336, 4.000000000000000000 ) ) ;
#4717=ORIENTED_EDGE ( 'NONE', *, *, #92517, .F. ) ;
#4718=CARTESIAN_POINT ( 'NONE',  ( 8.629999999999995453, 41.24999999999999289, 6.250000000000000000 ) ) ;
#4724=AXIS2_PLACEMENT_3D ( 'NONE', #49432, #79936, #85981 ) ;
#4728=ORIENTED_EDGE ( 'NONE', *, *, #92365, .F. ) ;
#4733=AXIS2_PLACEMENT_3D ( 'NONE', #83346, #98378, #92318 ) ;
#4743=DIRECTION ( 'NONE',  ( 0.000000000000000000, 0.000000000000000000, 1.000000000000000000 ) ) ;
#4752=CARTESIAN_POINT ( 'NONE',  ( 8.979999999999991545, 18.00000000000000355, -2.900000000000000799 ) ) ;
#4763=CARTESIAN_POINT ( 'NONE',  ( -13.05265508282193920, 90.73577164613084278, 7.477963345815892282 ) ) ;
#4767=FACE_OUTER_BOUND ( 'NONE', #78218, .T. ) ;
#4777=CIRCLE ( 'NONE', #12751, 2.899999999999999911 ) ;
#4787=LINE ( 'NONE', #20771, #96275 ) ;
#4789=FILL_AREA_STYLE_COLOUR ( '', #93108 ) ;
#4794=SURFACE_SIDE_STYLE ('',( #80784 ) ) ;
#4812=EDGE_CURVE ( 'NONE', #11855, #33481, #21871, .T. ) ;
#4828=( NAMED_UNIT ( * ) PLANE_ANGLE_UNIT ( ) SI_UNIT ( $, .RADIAN. ) );
#4829=ORIENTED_EDGE ( 'NONE', *, *, #58243, .F. ) ;
#4836=ORIENTED_EDGE ( 'NONE', *, *, #97835, .T. ) ;
#4838=DIRECTION ( 'NONE',  ( 0.000000000000000000, 1.000000000000000000, -0.000000000000000000 ) ) ;
#4853=CARTESIAN_POINT ( 'NONE',  ( -10.29975640502598289, 43.93058911311638326, 0.000000000000000000 ) ) ;
#4857=EDGE_CURVE ( 'NONE', #52732, #40706, #19125, .T. ) ;
#4890=CARTESIAN_POINT ( 'NONE',  ( -5.999999999999994671, 43.00000000000000000, -6.500000000000000888 ) ) ;
#4899=CYLINDRICAL_SURFACE ( 'NONE', #2859, 0.09999999999999982514 ) ;
#4911=VECTOR ( 'NONE', #55457, 1000.000000000000000 ) ;
#4914=LINE ( 'NONE', #42416, #2202 ) ;
#4916=CIRCLE ( 'NONE', #65556, 0.2500000000000002220 ) ;
#4925=CARTESIAN_POINT ( 'NONE',  ( -4.000000000000000000, 10.00000000000000000, 2.500000000000000000 ) ) ;
#4928=CIRCLE ( 'NONE', #68806, 7.000000000000002665 ) ;
#4936=CARTESIAN_POINT ( 'NONE',  ( -7.750000000000000000, 40.99999999999999289, -4.000000000000000000 ) ) ;
#4954=CYLINDRICAL_SURFACE ( 'NONE', #20204, 2.000000000000000888 ) ;
#4983=ORIENTED_EDGE ( 'NONE', *, *, #80581, .F. ) ;
#4989=CARTESIAN_POINT ( 'NONE',  ( -7.124975165218884854, -78.82169502743931844, 2.500000000000000000 ) ) ;
#4998=ORIENTED_EDGE ( 'NONE', *, *, #73140, .F. ) ;
#5008=LINE ( 'NONE', #65490, #38808 ) ;
#5012=CIRCLE ( 'NONE', #60887, 0.2500000000000002220 ) ;
#5021=VERTEX_POINT ( 'NONE', #33277 ) ;
#5029=CARTESIAN_POINT ( 'NONE',  ( 1.379999999999981908, 20.99999999999999645, -1.249999999999987121 ) ) ;
#5035=LINE ( 'NONE', #58512, #5690 ) ;
#5036=AXIS2_PLACEMENT_3D ( 'NONE', #65620, #57633, #65125 ) ;
#5038=ADVANCED_FACE ( 'NONE', ( #93299 ), #73441, .F. ) ;
#5062=FACE_OUTER_BOUND ( 'NONE', #6236, .T. ) ;
#5072=CARTESIAN_POINT ( 'NONE',  ( -13.76201028429828277, 90.94474152336147199, 7.905771670467119705 ) ) ;
#5076=CARTESIAN_POINT ( 'NONE',  ( 4.600000000000003197, 98.49999999999998579, 8.000000000000000000 ) ) ;
#5078=CARTESIAN_POINT ( 'NONE',  ( -0.000000000000000000, 40.74999999999999289, -4.000000000000000000 ) ) ;
#5080=ORIENTED_EDGE ( 'NONE', *, *, #38357, .T. ) ;
#5081=ORIENTED_EDGE ( 'NONE', *, *, #31371, .T. ) ;
#5082=FACE_OUTER_BOUND ( 'NONE', #20745, .T. ) ;
#5103=SURFACE_STYLE_USAGE ( .BOTH. , #72109 ) ;
#5109=ORIENTED_EDGE ( 'NONE', *, *, #16488, .T. ) ;
#5116=CARTESIAN_POINT ( 'NONE',  ( -6.560019409699617832, -50.64698701990471363, 3.750000000000000444 ) ) ;
#5120=DIRECTION ( 'NONE',  ( -0.000000000000000000, -1.000000000000000000, 0.000000000000000000 ) ) ;
#5129=LINE ( 'NONE', #35619, #63277 ) ;
#5139=CARTESIAN_POINT ( 'NONE',  ( -3.500000000000000444, 1.019547802438453887, -2.750000000000000444 ) ) ;
#5148=CARTESIAN_POINT ( 'NONE',  ( -11.42353084996827484, -90.30959216425827663, -4.000000000001802114 ) ) ;
#5161=CARTESIAN_POINT ( 'NONE',  ( -7.750000000000000000, 79.82179676972448590, 6.250000000000000000 ) ) ;
#5166=ORIENTED_EDGE ( 'NONE', *, *, #81160, .F. ) ;
#5168=EDGE_CURVE ( 'NONE', #26330, #29532, #19761, .T. ) ;
#5202=VECTOR ( 'NONE', #74933, 1000.000000000000114 ) ;
#5205=DIRECTION ( 'NONE',  ( 1.000000000000000000, 0.000000000000000000, 0.000000000000000000 ) ) ;
#5206=CIRCLE ( 'NONE', #35521, 2.000000000000000888 ) ;
#5207=ORIENTED_EDGE ( 'NONE', *, *, #9128, .T. ) ;
#5214=AXIS2_PLACEMENT_3D ( 'NONE', #77425, #3294, #91949 ) ;
#5220=ORIENTED_EDGE ( 'NONE', *, *, #11409, .F. ) ;
#5234=EDGE_LOOP ( 'NONE', ( #82702, #50428, #14183, #75758 ) ) ;
#5238=SPHERICAL_SURFACE ( 'NONE', #18077, 0.2500000000000000000 ) ;
#5243=CARTESIAN_POINT ( 'NONE',  ( 6.349999999999995204, -97.00000000000000000, 4.000000000000000000 ) ) ;
#5251=( NAMED_UNIT ( * ) SI_UNIT ( $, .STERADIAN. ) SOLID_ANGLE_UNIT ( ) );
#5266=CARTESIAN_POINT ( 'NONE',  ( 8.880000000000020322, 80.32179676972448590, 4.250000000000000000 ) ) ;
#5273=CARTESIAN_POINT ( 'NONE',  ( 14.49999999999999822, 75.00000000000000000, -6.500000000000000888 ) ) ;
#5277=CARTESIAN_POINT ( 'NONE',  ( 6.935112714462088768, -80.58076677624440265, 3.750000000000000888 ) ) ;
#5283=VERTEX_POINT ( 'NONE', #45723 ) ;
#5296=VECTOR ( 'NONE', #50825, 1000.000000000000000 ) ;
#5309=VERTEX_POINT ( 'NONE', #21754 ) ;
#5317=LINE ( 'NONE', #26321, #42278 ) ;
#5326=EDGE_CURVE ( 'NONE', #34926, #46257, #22244, .T. ) ;
#5332=EDGE_LOOP ( 'NONE', ( #20026, #59252, #95572, #77600 ) ) ;
#5333=DIRECTION ( 'NONE',  ( 0.000000000000000000, -0.000000000000000000, 1.000000000000000000 ) ) ;
#5334=EDGE_CURVE ( 'NONE', #16387, #65307, #76658, .T. ) ;
#5338=EDGE_CURVE ( 'NONE', #3713, #15093, #33534, .T. ) ;
#5344=( GEOMETRIC_REPRESENTATION_CONTEXT ( 3 ) GLOBAL_UNCERTAINTY_ASSIGNED_CONTEXT ( ( #7477 ) ) GLOBAL_UNIT_ASSIGNED_CONTEXT ( ( #30333, #16829, #15371 ) ) REPRESENTATION_CONTEXT ( 'NONE', 'WORKASPACE' ) );
#5346=ORIENTED_EDGE ( 'NONE', *, *, #11850, .F. ) ;
#5351=LINE ( 'NONE', #80350, #31879 ) ;
#5361=EDGE_CURVE ( 'NONE', #11450, #7152, #37743, .T. ) ;
#5371=VECTOR ( 'NONE', #90727, 1000.000000000000000 ) ;
#5387=CARTESIAN_POINT ( 'NONE',  ( -9.347645168806021587, 88.42200471242378512, -5.276767730577755167 ) ) ;
#5400=CYLINDRICAL_SURFACE ( 'NONE', #53149, 4.000000000000001776 ) ;
#5423=CARTESIAN_POINT ( 'NONE',  ( 8.879999999999995453, 40.74999999999999289, 4.250000000000000000 ) ) ;
#5430=FACE_OUTER_BOUND ( 'NONE', #68172, .T. ) ;
#5433=UNCERTAINTY_MEASURE_WITH_UNIT (LENGTH_MEASURE( 1.000000000000000082E-05 ), #98904, 'distance_accuracy_value', 'NONE');
#5455=( LENGTH_UNIT ( ) NAMED_UNIT ( * ) SI_UNIT ( .MILLI., .METRE. ) );
#5465=EDGE_LOOP ( 'NONE', ( #41750, #43109, #52802, #25495 ) ) ;
#5486=DIRECTION ( 'NONE',  ( -0.000000000000000000, 0.000000000000000000, 1.000000000000000000 ) ) ;
#5493=CARTESIAN_POINT ( 'NONE',  ( 6.879999999999995453, 43.00000000000000000, -6.500000000000000888 ) ) ;
#5497=DIRECTION ( 'NONE',  ( -0.5905099943842175847, -0.8070303256584298035, 0.000000000000000000 ) ) ;
#5523=CARTESIAN_POINT ( 'NONE',  ( 4.469999999999999751, 10.25000000000000000, -3.750000000000000000 ) ) ;
#5528=CARTESIAN_POINT ( 'NONE',  ( -3.250000000000001776, 0.08822490956012368768, -2.500000000000000888 ) ) ;
#5534=FILL_AREA_STYLE_COLOUR ( '', #4112 ) ;
#5536=EDGE_CURVE ( 'NONE', #62370, #89076, #23235, .T. ) ;
#5539=DIRECTION ( 'NONE',  ( -0.000000000000000000, -0.000000000000000000, 1.000000000000000000 ) ) ;
#5545=VECTOR ( 'NONE', #42897, 1000.000000000000000 ) ;
#5552=AXIS2_PLACEMENT_3D ( 'NONE', #33533, #26059, #46580 ) ;
#5565=CARTESIAN_POINT ( 'NONE',  ( -3.889970118670758037, -8.287734203605921834, -4.000000000000000888 ) ) ;
#5567=ORIENTED_EDGE ( 'NONE', *, *, #85560, .F. ) ;
#5576=CARTESIAN_POINT ( 'NONE',  ( 17.74999999999999645, 78.80384757729336798, 4.000000000000000000 ) ) ;
#5580=EDGE_CURVE ( 'NONE', #36801, #21688, #34438, .T. ) ;
#5587=( NAMED_UNIT ( * ) SI_UNIT ( $, .STERADIAN. ) SOLID_ANGLE_UNIT ( ) );
#5588=EDGE_LOOP ( 'NONE', ( #76678, #1432, #7593, #62145 ) ) ;
#5595=ORIENTED_EDGE ( 'NONE', *, *, #20390, .T. ) ;
#5604=AXIS2_PLACEMENT_3D ( 'NONE', #70959, #55455, #38981 ) ;
#5612=( GEOMETRIC_REPRESENTATION_CONTEXT ( 3 ) GLOBAL_UNCERTAINTY_ASSIGNED_CONTEXT ( ( #79519 ) ) GLOBAL_UNIT_ASSIGNED_CONTEXT ( ( #29817, #24318, #835 ) ) REPRESENTATION_CONTEXT ( 'NONE', 'WORKASPACE' ) );
#5613=DIRECTION ( 'NONE',  ( 0.000000000000000000, 1.000000000000000000, 0.000000000000000000 ) ) ;
#5617=CARTESIAN_POINT ( 'NONE',  ( -4.536330790005646207, -17.54398820868007647, 3.750000000000000000 ) ) ;
#5618=DIRECTION ( 'NONE',  ( 0.000000000000000000, 0.000000000000000000, -1.000000000000000000 ) ) ;
#5640=LINE ( 'NONE', #36117, #86845 ) ;
#5641=( LENGTH_UNIT ( ) NAMED_UNIT ( * ) SI_UNIT ( .MILLI., .METRE. ) );
#5649=CYLINDRICAL_SURFACE ( 'NONE', #86302, 0.2500000000000002220 ) ;
#5663=ORIENTED_EDGE ( 'NONE', *, *, #59717, .T. ) ;
#5673=DIRECTION ( 'NONE',  ( -0.000000000000000000, 0.000000000000000000, 1.000000000000000000 ) ) ;
#5677=ORIENTED_EDGE ( 'NONE', *, *, #22946, .F. ) ;
#5690=VECTOR ( 'NONE', #51015, 1000.000000000000000 ) ;
#5693=DIRECTION ( 'NONE',  ( 1.000000000000000000, 0.000000000000000000, 0.000000000000000000 ) ) ;
#5697=LINE ( 'NONE', #15176, #55510 ) ;
#5705=COLOUR_RGB ( '', 0.08235294, 0.09019608, 0.10196078) ;
#5719=COLOUR_RGB ( '', 0.40784314, 0.44705882, 0.49803922) ;
#5722=EDGE_LOOP ( 'NONE', ( #23565, #73701, #81169, #13580 ) ) ;
#5726=DIRECTION ( 'NONE',  ( 0.000000000000000000, 0.000000000000000000, 1.000000000000000000 ) ) ;
#5754=DIRECTION ( 'NONE',  ( 0.000000000000000000, 0.000000000000000000, 1.000000000000000000 ) ) ;
#5766=EDGE_CURVE ( 'NONE', #28519, #35759, #54679, .T. ) ;
#5774=CARTESIAN_POINT ( 'NONE',  ( -11.26637474388419591, 89.93360374965293147, -6.408881440111466432 ) ) ;
#5775=FACE_OUTER_BOUND ( 'NONE', #45800, .T. ) ;
#5782=CARTESIAN_POINT ( 'NONE',  ( -53.17073170731706711, 42.53658536585359684, -8.000000000000000000 ) ) ;
#5791=EDGE_CURVE ( 'NONE', #16659, #47034, #62178, .T. ) ;
#5796=CARTESIAN_POINT ( 'NONE',  ( -7.750000000000000000, 79.82179676972448590, -6.250000000000000000 ) ) ;
#5804=FILL_AREA_STYLE ('',( #74276 ) ) ;
#5806=ADVANCED_FACE ( 'NONE', ( #1717 ), #32873, .T. ) ;
#5817=ORIENTED_EDGE ( 'NONE', *, *, #32860, .F. ) ;
#5821=EDGE_LOOP ( 'NONE', ( #8582, #74835, #91753, #14856 ) ) ;
#5837=AXIS2_PLACEMENT_3D ( 'NONE', #95124, #50121, #80631 ) ;
#5840=CARTESIAN_POINT ( 'NONE',  ( 3.969999999999999751, 10.25000000000000000, 2.750000000000000000 ) ) ;
#5868=DIRECTION ( 'NONE',  ( 0.000000000000000000, 0.000000000000000000, -1.000000000000000000 ) ) ;
#5877=DIRECTION ( 'NONE',  ( 0.000000000000000000, 0.000000000000000000, 1.000000000000000000 ) ) ;
#5883=VERTEX_POINT ( 'NONE', #96647 ) ;
#5885=ADVANCED_FACE ( 'NONE', ( #35633 ), #8897, .T. ) ;
#5886=AXIS2_PLACEMENT_3D ( 'NONE', #23709, #8679, #62155 ) ;
#5898=( NAMED_UNIT ( * ) PLANE_ANGLE_UNIT ( ) SI_UNIT ( $, .RADIAN. ) );
#5902=FILL_AREA_STYLE ('',( #75873 ) ) ;
#5919=CARTESIAN_POINT ( 'NONE',  ( -8.000000000000000000, 80.99999999999994316, 0.000000000000000000 ) ) ;
#5921=CYLINDRICAL_SURFACE ( 'NONE', #48845, 0.1000000000000000333 ) ;
#5929=VECTOR ( 'NONE', #2249, 1000.000000000000000 ) ;
#5933=DIRECTION ( 'NONE',  ( -0.000000000000000000, -0.000000000000000000, 1.000000000000000000 ) ) ;
#5936=MECHANICAL_DESIGN_GEOMETRIC_PRESENTATION_REPRESENTATION('',(#49032),#61800);
#5939=CARTESIAN_POINT ( 'NONE',  ( -6.599999999999995204, -97.00000000000000000, -3.750000000000000000 ) ) ;
#5940=CARTESIAN_POINT ( 'NONE',  ( -10.53011945866294852, -98.59345040283277228, -4.000000000000000000 ) ) ;
#5947=CARTESIAN_POINT ( 'NONE',  ( -10.91752705534077705, -97.59869434427200474, -3.749999999999999112 ) ) ;
#5974=CARTESIAN_POINT ( 'NONE',  ( -6.617417514236028531, -58.37570470593282579, 2.500000000000000000 ) ) ;
#5979=CARTESIAN_POINT ( 'NONE',  ( 9.261744320155163024, -15.50732398184953276, 4.000000000000000000 ) ) ;
#5982=AXIS2_PLACEMENT_3D ( 'NONE', #7788, #21803, #82782 ) ;
#5995=CARTESIAN_POINT ( 'NONE',  ( 0.4400000000000020006, 1.019547802438468986, -2.500000000000000000 ) ) ;
#5997=ADVANCED_FACE ( 'NONE', ( #49157 ), #57637, .T. ) ;
#6036=LINE ( 'NONE', #44513, #17694 ) ;
#6045=CIRCLE ( 'NONE', #33134, 0.5000000000000000000 ) ;
#6052=CARTESIAN_POINT ( 'NONE',  ( 11.43652560662874507, -81.64049707262192612, -3.749999999999999112 ) ) ;
#6058=CARTESIAN_POINT ( 'NONE',  ( -13.69999999999999751, 99.99999999999998579, -8.525133428036873795 ) ) ;
#6080=EDGE_LOOP ( 'NONE', ( #21462, #10142, #42837, #199 ) ) ;
#6098=DIRECTION ( 'NONE',  ( 0.000000000000000000, -1.000000000000000000, 0.000000000000000000 ) ) ;
#6100=AXIS2_PLACEMENT_3D ( 'NONE', #3155, #41652, #40164 ) ;
#6102=SURFACE_STYLE_USAGE ( .BOTH. , #6588 ) ;
#6103=CARTESIAN_POINT ( 'NONE',  ( -6.030800153576633349, -39.80424705863364920, 3.750000000000001332 ) ) ;
#6107=VERTEX_POINT ( 'NONE', #8466 ) ;
#6108=DIRECTION ( 'NONE',  ( -4.606671024408299627E-17, -2.115048048893883575E-15, -1.000000000000000000 ) ) ;
#6124=SURFACE_STYLE_FILL_AREA ( #51122 ) ;
#6126=DIRECTION ( 'NONE',  ( -1.000000000000000000, -0.000000000000000000, -0.000000000000000000 ) ) ;
#6134=( NAMED_UNIT ( * ) SI_UNIT ( $, .STERADIAN. ) SOLID_ANGLE_UNIT ( ) );
#6157=ORIENTED_EDGE ( 'NONE', *, *, #94629, .T. ) ;
#6158=MECHANICAL_DESIGN_GEOMETRIC_PRESENTATION_REPRESENTATION('',(#54048),#79609);
#6159=CARTESIAN_POINT ( 'NONE',  ( 5.429172911446037197, -28.64165983034504137, 2.499999999999999556 ) ) ;
#6161=ORIENTED_EDGE ( 'NONE', *, *, #86978, .F. ) ;
#6163=CARTESIAN_POINT ( 'NONE',  ( 0.000000000000000000, -97.00000000000000000, -3.750000000000000000 ) ) ;
#6170=CARTESIAN_POINT ( 'NONE',  ( -7.750000000000000000, 40.74999999999999289, -4.250000000000000000 ) ) ;
#6176=CARTESIAN_POINT ( 'NONE',  ( 4.380000000000002558, 1.019547802438462547, -2.500000000000000000 ) ) ;
#6181=VERTEX_POINT ( 'NONE', #60094 ) ;
#6183=ORIENTED_EDGE ( 'NONE', *, *, #71947, .F. ) ;
#6185=ORIENTED_EDGE ( 'NONE', *, *, #74797, .F. ) ;
#6194=TOROIDAL_SURFACE ( 'NONE', #28522, 3.250000000000001332, 0.2500000000000000000 ) ;
#6205=CARTESIAN_POINT ( 'NONE',  ( 11.49999999999999645, 75.00000000000000000, 6.500000000000000888 ) ) ;
#6214=CARTESIAN_POINT ( 'NONE',  ( -4.000000000000000000, 37.00000000000000000, -3.750000000000000000 ) ) ;
#6215=SURFACE_SIDE_STYLE ('',( #38203 ) ) ;
#6220=CIRCLE ( 'NONE', #74881, 1.249999999999987121 ) ;
#6236=EDGE_LOOP ( 'NONE', ( #68174, #77554, #41484, #96842 ) ) ;
#6243=CARTESIAN_POINT ( 'NONE',  ( -8.000000000000000000, 83.99999999999994316, 3.000000000000000000 ) ) ;
#6245=CARTESIAN_POINT ( 'NONE',  ( 8.879999999999991900, 76.07179676972447169, -6.250000000000000000 ) ) ;
#6252=CARTESIAN_POINT ( 'NONE',  ( -3.749999999999988010, -5.564482262735336175E-16, -4.250000000000000000 ) ) ;
#6254=( GEOMETRIC_REPRESENTATION_CONTEXT ( 3 ) GLOBAL_UNCERTAINTY_ASSIGNED_CONTEXT ( ( #78215 ) ) GLOBAL_UNIT_ASSIGNED_CONTEXT ( ( #91181, #20726, #21721 ) ) REPRESENTATION_CONTEXT ( 'NONE', 'WORKASPACE' ) );
#6267=CARTESIAN_POINT ( 'NONE',  ( 9.729335482455997663, -19.62342160288553217, -4.000000000000000000 ) ) ;
#6272=ADVANCED_FACE ( 'NONE', ( #46463 ), #46946, .F. ) ;
#6277=CYLINDRICAL_SURFACE ( 'NONE', #67127, 0.2500000000000002220 ) ;
#6283=EDGE_LOOP ( 'NONE', ( #73638, #58172, #10041, #97104 ) ) ;
#6295=CARTESIAN_POINT ( 'NONE',  ( 5.429172911440337757, -28.64165983023028517, -2.499999999999999556 ) ) ;
#6308=EDGE_LOOP ( 'NONE', ( #89162, #17279, #694, #84296 ) ) ;
#6329=FILL_AREA_STYLE ('',( #46794 ) ) ;
#6341=EDGE_CURVE ( 'NONE', #87452, #91690, #83919, .T. ) ;
#6343=CARTESIAN_POINT ( 'NONE',  ( 6.757497259943707313, -58.30388498733396574, -2.750000000000000000 ) ) ;
#6346=ORIENTED_EDGE ( 'NONE', *, *, #23931, .F. ) ;
#6347=DIRECTION ( 'NONE',  ( -1.000000000000000000, 0.000000000000000000, 0.000000000000000000 ) ) ;
#6350=CARTESIAN_POINT ( 'NONE',  ( -13.77612262535527954, 90.93158326518027934, -7.883772450803742338 ) ) ;
#6359=DIRECTION ( 'NONE',  ( 1.000000000000000000, 0.000000000000000000, -0.000000000000000000 ) ) ;
#6373=VERTEX_POINT ( 'NONE', #59109 ) ;
#6380=DIRECTION ( 'NONE',  ( 0.000000000000000000, 0.000000000000000000, 1.000000000000000000 ) ) ;
#6395=CARTESIAN_POINT ( 'NONE',  ( 2.550000000000003819, 99.99999999999998579, 8.000000000000000000 ) ) ;
#6400=EDGE_CURVE ( 'NONE', #86598, #91147, #58421, .T. ) ;
#6406=CIRCLE ( 'NONE', #52726, 0.2500000000000002220 ) ;
#6416=CARTESIAN_POINT ( 'NONE',  ( 4.721518086276724979, -3.620742741961517019, 4.000000000000000000 ) ) ;
#6441=DIRECTION ( 'NONE',  ( -1.000000000000000000, -6.938893903907221278E-15, -0.000000000000000000 ) ) ;
#6456=CARTESIAN_POINT ( 'NONE',  ( -3.749999999999994671, 43.00000000000000711, 4.250000000000000000 ) ) ;
#6457=CARTESIAN_POINT ( 'NONE',  ( 9.511407825589754950, -15.49433182431968170, 3.750000000000000000 ) ) ;
#6467=UNCERTAINTY_MEASURE_WITH_UNIT (LENGTH_MEASURE( 1.000000000000000082E-05 ), #63702, 'distance_accuracy_value', 'NONE');
#6474=CARTESIAN_POINT ( 'NONE',  ( -13.65756908232610378, 90.97036336906094789, -7.949095025303489770 ) ) ;
#6496=CARTESIAN_POINT ( 'NONE',  ( -4.249999999999999112, 78.07179676972445748, 6.250000000000000000 ) ) ;
#6505=DIRECTION ( 'NONE',  ( 1.000000000000000000, 0.000000000000000000, 0.000000000000000000 ) ) ;
#6507=STYLED_ITEM ( 'NONE', ( #53339 ), #34314 ) ;
#6517=DIRECTION ( 'NONE',  ( 0.000000000000000000, -1.000000000000000000, 0.000000000000000000 ) ) ;
#6526=DIRECTION ( 'NONE',  ( -1.000000000000000000, -0.000000000000000000, -0.000000000000000000 ) ) ;
#6536=EDGE_LOOP ( 'NONE', ( #11013, #6809, #53650, #28064 ) ) ;
#6547=CARTESIAN_POINT ( 'NONE',  ( -7.750000000000000000, 40.74999999999999289, 4.000000000000000000 ) ) ;
#6552=VERTEX_POINT ( 'NONE', #49898 ) ;
#6565=EDGE_CURVE ( 'NONE', #89076, #37577, #24771, .T. ) ;
#6566=ORIENTED_EDGE ( 'NONE', *, *, #79404, .F. ) ;
#6571=EDGE_LOOP ( 'NONE', ( #73157, #22574, #58174, #50847 ) ) ;
#6588=SURFACE_SIDE_STYLE ('',( #75082 ) ) ;
#6589=DIRECTION ( 'NONE',  ( -0.5905099943842175847, -0.8070303256584298035, 0.000000000000000000 ) ) ;
#6620=CARTESIAN_POINT ( 'NONE',  ( -9.024359497401759356, 75.07164295747612925, 3.000000000000000000 ) ) ;
#6639=EDGE_CURVE ( 'NONE', #981, #82789, #88557, .T. ) ;
#6647=CARTESIAN_POINT ( 'NONE',  ( 4.669717816210469330, -13.81568353613706535, 2.499999999999999556 ) ) ;
#6660=CARTESIAN_POINT ( 'NONE',  ( -11.58433430580200607, -69.52997016218412796, 4.000000000003603340 ) ) ;
#6679=DIRECTION ( 'NONE',  ( 0.000000000000000000, 0.000000000000000000, -1.000000000000000000 ) ) ;
#6680=CIRCLE ( 'NONE', #54551, 8.250000000000007105 ) ;
#6685=ORIENTED_EDGE ( 'NONE', *, *, #23632, .F. ) ;
#6694=MECHANICAL_DESIGN_GEOMETRIC_PRESENTATION_REPRESENTATION('',(#22697),#80123);
#6699=DIRECTION ( 'NONE',  ( -0.000000000000000000, -1.000000000000000000, -0.000000000000000000 ) ) ;
#6703=CARTESIAN_POINT ( 'NONE',  ( 14.35000000000000142, 98.50000000000001421, -8.000000000000000000 ) ) ;
#6716=DIRECTION ( 'NONE',  ( -1.000000000000000000, 0.000000000000000000, -0.000000000000000000 ) ) ;
#6734=CARTESIAN_POINT ( 'NONE',  ( 42.87872917473848844, 58.60092987214253668, -8.000000000000000000 ) ) ;
#6744=DIRECTION ( 'NONE',  ( -0.000000000000000000, -0.000000000000000000, -1.000000000000000000 ) ) ;
#6747=CIRCLE ( 'NONE', #67415, 0.2500000000000002220 ) ;
#6756=CIRCLE ( 'NONE', #35510, 0.2499999999999978351 ) ;
#6757=CIRCLE ( 'NONE', #30722, 6.599999999999995204 ) ;
#6761=ORIENTED_EDGE ( 'NONE', *, *, #32079, .F. ) ;
#6763=AXIS2_PLACEMENT_3D ( 'NONE', #6170, #73664, #67162 ) ;
#6764=CARTESIAN_POINT ( 'NONE',  ( 11.08992015845062262, -87.81706477660959820, -4.000000000000000000 ) ) ;
#6774=( LENGTH_UNIT ( ) NAMED_UNIT ( * ) SI_UNIT ( .MILLI., .METRE. ) );
#6778=ORIENTED_EDGE ( 'NONE', *, *, #35765, .T. ) ;
#6792=CIRCLE ( 'NONE', #57867, 0.2500000000000002220 ) ;
#6793=PRESENTATION_STYLE_ASSIGNMENT (( #14808 ) ) ;
#6809=ORIENTED_EDGE ( 'NONE', *, *, #79708, .T. ) ;
#6814=CARTESIAN_POINT ( 'NONE',  ( 11.24699797944280100, 54.09857164847241506, -3.000000000000000000 ) ) ;
#6824=VECTOR ( 'NONE', #27721, 1000.000000000000000 ) ;
#6825=AXIS2_PLACEMENT_3D ( 'NONE', #66981, #50987, #81481 ) ;
#6832=( LENGTH_UNIT ( ) NAMED_UNIT ( * ) SI_UNIT ( .MILLI., .METRE. ) );
#6836=CYLINDRICAL_SURFACE ( 'NONE', #34342, 0.2500000000000002220 ) ;
#6840=ORIENTED_EDGE ( 'NONE', *, *, #33985, .T. ) ;
#6842=( NAMED_UNIT ( * ) SI_UNIT ( $, .STERADIAN. ) SOLID_ANGLE_UNIT ( ) );
#6844=CARTESIAN_POINT ( 'NONE',  ( 4.441081520557000673, -2.684960557620042376, -2.500000000000000888 ) ) ;
#6847=VERTEX_POINT ( 'NONE', #68860 ) ;
#6852=VECTOR ( 'NONE', #20822, 1000.000000000000000 ) ;
#6866=VECTOR ( 'NONE', #78764, 1000.000000000000000 ) ;
#6868=SURFACE_STYLE_FILL_AREA ( #15374 ) ;
#6880=PRESENTATION_STYLE_ASSIGNMENT (( #83861 ) ) ;
#6894=EDGE_CURVE ( 'NONE', #9920, #69773, #55072, .T. ) ;
#6909=STYLED_ITEM ( 'NONE', ( #54805 ), #92469 ) ;
#6922=CARTESIAN_POINT ( 'NONE',  ( 6.825238882348372726, -50.90120388559804354, 4.000000000000000000 ) ) ;
#6923=SURFACE_SIDE_STYLE ('',( #98442 ) ) ;
#6932=EDGE_CURVE ( 'NONE', #96670, #30525, #91347, .T. ) ;
#6944=AXIS2_PLACEMENT_3D ( 'NONE', #55454, #18933, #72405 ) ;
#6946=DIRECTION ( 'NONE',  ( -1.000000000000000000, 0.000000000000000000, -0.000000000000000000 ) ) ;
#6947=ORIENTED_EDGE ( 'NONE', *, *, #35382, .F. ) ;
#6952=EDGE_CURVE ( 'NONE', #49408, #717, #77320, .T. ) ;
#6957=CARTESIAN_POINT ( 'NONE',  ( 8.879999999999991900, 76.07179676972447169, 6.500000000000000888 ) ) ;
#6960=DIRECTION ( 'NONE',  ( 1.000000000000000000, 0.000000000000000000, 0.000000000000000000 ) ) ;
#6961=LINE ( 'NONE', #36966, #60133 ) ;
#6971=CARTESIAN_POINT ( 'NONE',  ( -8.004782461319718934, 84.51756810411845322, 3.750000000000000000 ) ) ;
#7010=ORIENTED_EDGE ( 'NONE', *, *, #19227, .F. ) ;
#7021=CARTESIAN_POINT ( 'NONE',  ( 0.000000000000000000, 80.32179676972448590, 4.000000000000000000 ) ) ;
#7025=CARTESIAN_POINT ( 'NONE',  ( -6.000000000000000000, 78.07179676972447169, -6.250000000000000000 ) ) ;
#7039=CARTESIAN_POINT ( 'NONE',  ( -7.322357042924514836, -84.41015717759208314, -4.000000000000000000 ) ) ;
#7046=CARTESIAN_POINT ( 'NONE',  ( -8.000000000000000000, 41.24999999999999289, -6.250000000000000000 ) ) ;
#7048=CARTESIAN_POINT ( 'NONE',  ( -12.23643000159860250, 90.44368800334666503, -7.046674173440611533 ) ) ;
#7060=EDGE_LOOP ( 'NONE', ( #17501, #96359, #87481, #19133 ) ) ;
#7082=DIRECTION ( 'NONE',  ( -0.000000000000000000, 0.000000000000000000, -1.000000000000000000 ) ) ;
#7085=CARTESIAN_POINT ( 'NONE',  ( 8.630000000000000782, 1.019547802438458550, 4.000000000000000000 ) ) ;
#7091=VERTEX_POINT ( 'NONE', #61340 ) ;
#7106=ORIENTED_EDGE ( 'NONE', *, *, #67725, .T. ) ;
#7115=AXIS2_PLACEMENT_3D ( 'NONE', #90595, #31080, #91600 ) ;
#7121=CARTESIAN_POINT ( 'NONE',  ( -19.64999999999999858, 98.99999999999998579, 7.750000000000000000 ) ) ;
#7132=UNCERTAINTY_MEASURE_WITH_UNIT (LENGTH_MEASURE( 1.000000000000000082E-05 ), #61334, 'distance_accuracy_value', 'NONE');
#7145=CARTESIAN_POINT ( 'NONE',  ( 6.579634127946655475, -87.99828267815715321, -4.000000000000000000 ) ) ;
#7147=VECTOR ( 'NONE', #32620, 1000.000000000000000 ) ;
#7148=ORIENTED_EDGE ( 'NONE', *, *, #18304, .T. ) ;
#7152=VERTEX_POINT ( 'NONE', #17339 ) ;
#7159=CARTESIAN_POINT ( 'NONE',  ( -8.468251460007511611, -9.345277391842092385, 4.000000000000000000 ) ) ;
#7165=CARTESIAN_POINT ( 'NONE',  ( -3.750000000000000000, 10.25000000000000000, -2.750000000000000000 ) ) ;
#7167=ADVANCED_FACE ( 'NONE', ( #3807 ), #56312, .T. ) ;
#7185=VERTEX_POINT ( 'NONE', #18310 ) ;
#7187=ORIENTED_EDGE ( 'NONE', *, *, #63876, .T. ) ;
#7194=FACE_OUTER_BOUND ( 'NONE', #61423, .T. ) ;
#7199=ORIENTED_EDGE ( 'NONE', *, *, #13544, .T. ) ;
#7200=AXIS2_PLACEMENT_3D ( 'NONE', #66375, #51382, #13382 ) ;
#7203=ORIENTED_EDGE ( 'NONE', *, *, #46528, .T. ) ;
#7208=DIRECTION ( 'NONE',  ( 1.000000000000000000, 0.000000000000000000, 0.000000000000000000 ) ) ;
#7209=FACE_OUTER_BOUND ( 'NONE', #93687, .T. ) ;
#7211=PLANE ( 'NONE',  #2913 ) ;
#7220=VECTOR ( 'NONE', #80386, 1000.000000000000000 ) ;
#7221=ADVANCED_FACE ( 'NONE', ( #40329 ), #1113, .T. ) ;
#7227=ORIENTED_EDGE ( 'NONE', *, *, #90627, .T. ) ;
#7238=AXIS2_PLACEMENT_3D ( 'NONE', #81577, #99, #36592 ) ;
#7243=EDGE_CURVE ( 'NONE', #13092, #94718, #71020, .T. ) ;
#7245=SURFACE_STYLE_FILL_AREA ( #45231 ) ;
#7259=EDGE_CURVE ( 'NONE', #91314, #92036, #51761, .T. ) ;
#7260=CARTESIAN_POINT ( 'NONE',  ( 9.779999999999990479, 20.99999999999999645, -2.899999999999999911 ) ) ;
#7266=CARTESIAN_POINT ( 'NONE',  ( 11.01507687156111892, -96.09620168231128901, -3.750000000000000000 ) ) ;
#7278=ORIENTED_EDGE ( 'NONE', *, *, #26619, .F. ) ;
#7279=ORIENTED_EDGE ( 'NONE', *, *, #2661, .F. ) ;
#7292=SURFACE_STYLE_USAGE ( .BOTH. , #59285 ) ;
#7294=EDGE_CURVE ( 'NONE', #19902, #89066, #74751, .T. ) ;
#7296=SURFACE_STYLE_FILL_AREA ( #91267 ) ;
#7297=ORIENTED_EDGE ( 'NONE', *, *, #44366, .T. ) ;
#7302=CIRCLE ( 'NONE', #28044, 0.2500000000000002220 ) ;
#7309=VECTOR ( 'NONE', #78699, 1000.000000000000000 ) ;
#7310=ORIENTED_EDGE ( 'NONE', *, *, #81256, .T. ) ;
#7315=CARTESIAN_POINT ( 'NONE',  ( 9.879999999999990123, 20.99999999999999645, 0.000000000000000000 ) ) ;
#7328=AXIS2_PLACEMENT_3D ( 'NONE', #13014, #29986, #6505 ) ;
#7338=SURFACE_STYLE_FILL_AREA ( #6329 ) ;
#7350=VECTOR ( 'NONE', #70197, 1000.000000000000000 ) ;
#7351=CARTESIAN_POINT ( 'NONE',  ( 5.678900477119734447, -28.62996443916405909, -2.499999999996779909 ) ) ;
#7360=DIRECTION ( 'NONE',  ( 0.000000000000000000, 1.000000000000000000, 0.000000000000000000 ) ) ;
#7370=CARTESIAN_POINT ( 'NONE',  ( -10.07341714983716230, -32.14978703225411039, -4.000000000000000000 ) ) ;
#7374=SURFACE_STYLE_USAGE ( .BOTH. , #36876 ) ;
#7378=SURFACE_STYLE_USAGE ( .BOTH. , #39347 ) ;
#7387=ORIENTED_EDGE ( 'NONE', *, *, #94690, .T. ) ;
#7388=CARTESIAN_POINT ( 'NONE',  ( -9.543993260087553665, -28.01899697271202427, -4.000000000000000000 ) ) ;
#7394=SURFACE_STYLE_FILL_AREA ( #5902 ) ;
#7402=VECTOR ( 'NONE', #88247, 1000.000000000000114 ) ;
#7408=AXIS2_PLACEMENT_3D ( 'NONE', #44692, #6699, #98216 ) ;
#7414=DIRECTION ( 'NONE',  ( -0.000000000000000000, -0.000000000000000000, -1.000000000000000000 ) ) ;
#7429=DIRECTION ( 'NONE',  ( 1.000000000000000000, 6.938893903907221278E-15, -0.000000000000000000 ) ) ;
#7461=( NAMED_UNIT ( * ) SI_UNIT ( $, .STERADIAN. ) SOLID_ANGLE_UNIT ( ) );
#7467=CARTESIAN_POINT ( 'NONE',  ( 7.155629327958947350, -69.45263185074750822, -4.000000000000000000 ) ) ;
#7477=UNCERTAINTY_MEASURE_WITH_UNIT (LENGTH_MEASURE( 1.000000000000000082E-05 ), #30333, 'distance_accuracy_value', 'NONE');
#7478=CARTESIAN_POINT ( 'NONE',  ( -12.79762580178202214, 90.64749249312531276, 7.346077433007431878 ) ) ;
#7485=CARTESIAN_POINT ( 'NONE',  ( 4.380000000000000782, 1.019547802438464545, -2.750000000000000000 ) ) ;
#7505=CARTESIAN_POINT ( 'NONE',  ( 0.000000000000000000, 70.25000000000000000, -6.250000000000000000 ) ) ;
#7523=B_SPLINE_CURVE_WITH_KNOTS ( 'NONE', 3,
 ( #19032, #43976, #51993, #73489, #36989, #97020, #58990, #97511 ),
 .UNSPECIFIED., .F., .F.,
 ( 4, 2, 2, 4 ),
 ( 0.000000000000000000, 0.0004516266542298916719, 0.0009032533084597833438, 0.001806506616919566688 ),
 .UNSPECIFIED. ) ;
#7540=EDGE_CURVE ( 'NONE', #55430, #12785, #82268, .T. ) ;
#7542=DIRECTION ( 'NONE',  ( 0.000000000000000000, 0.000000000000000000, -1.000000000000000000 ) ) ;
#7548=CARTESIAN_POINT ( 'NONE',  ( -7.232415441807423129, -88.12698951299773853, -4.000000000000000000 ) ) ;
#7561=CIRCLE ( 'NONE', #71417, 0.2500000000000002220 ) ;
#7582=ORIENTED_EDGE ( 'NONE', *, *, #84272, .F. ) ;
#7587=DIRECTION ( 'NONE',  ( 0.000000000000000000, 0.000000000000000000, 1.000000000000000000 ) ) ;
#7593=ORIENTED_EDGE ( 'NONE', *, *, #39541, .F. ) ;
#7594=DIRECTION ( 'NONE',  ( -1.000000000000000000, 0.000000000000000000, 0.000000000000000000 ) ) ;
#7595=AXIS2_PLACEMENT_3D ( 'NONE', #4925, #73397, #21404 ) ;
#7597=DIRECTION ( 'NONE',  ( 0.8070303256584298035, -0.5905099943842175847, 0.000000000000000000 ) ) ;
#7609=SURFACE_SIDE_STYLE ('',( #16576 ) ) ;
#7613=DIRECTION ( 'NONE',  ( -0.000000000000000000, -0.000000000000000000, -1.000000000000000000 ) ) ;
#7624=DIRECTION ( 'NONE',  ( 1.000000000000000000, -0.000000000000000000, -0.000000000000000000 ) ) ;
#7628=CIRCLE ( 'NONE', #10821, 4.000000000000001776 ) ;
#7633=PRESENTATION_STYLE_ASSIGNMENT (( #53104 ) ) ;
#7637=CARTESIAN_POINT ( 'NONE',  ( 15.00000000000000000, 77.07179676972447169, 6.500000000000000888 ) ) ;
#7639=TOROIDAL_SURFACE ( 'NONE', #92195, 8.250000000000000000, 0.2500000000000000000 ) ;
#7668=CARTESIAN_POINT ( 'NONE',  ( -8.897278993079112297, -15.56326597358625108, 4.000000000000000000 ) ) ;
#7689=ADVANCED_FACE ( 'NONE', ( #59744 ), #68742, .F. ) ;
#7692=ORIENTED_EDGE ( 'NONE', *, *, #82620, .F. ) ;
#7703=CIRCLE ( 'NONE', #63554, 0.2499999999999980294 ) ;
#7706=( NAMED_UNIT ( * ) SI_UNIT ( $, .STERADIAN. ) SOLID_ANGLE_UNIT ( ) );
#7720=DIRECTION ( 'NONE',  ( 1.000000000000000000, 3.167963975439022915E-12, 0.000000000000000000 ) ) ;
#7729=ORIENTED_EDGE ( 'NONE', *, *, #11977, .T. ) ;
#7742=CYLINDRICAL_SURFACE ( 'NONE', #77668, 0.2500000000000002220 ) ;
#7749=TOROIDAL_SURFACE ( 'NONE', #44410, 2.899999999999999911, 0.1000000000000000056 ) ;
#7757=SURFACE_SIDE_STYLE ('',( #54210 ) ) ;
#7768=DIRECTION ( 'NONE',  ( 1.000000000000000000, 0.000000000000000000, -0.000000000000000000 ) ) ;
#7772=FACE_OUTER_BOUND ( 'NONE', #60279, .T. ) ;
#7775=AXIS2_PLACEMENT_3D ( 'NONE', #8913, #91926, #60436 ) ;
#7788=CARTESIAN_POINT ( 'NONE',  ( -6.000000000000000000, 78.07179676972447169, 4.000000000000000000 ) ) ;
#7795=ORIENTED_EDGE ( 'NONE', *, *, #76361, .T. ) ;
#7799=DIRECTION ( 'NONE',  ( 0.6246950475544238435, 0.7808688094430307203, 0.000000000000000000 ) ) ;
#7800=ORIENTED_EDGE ( 'NONE', *, *, #76887, .T. ) ;
#7808=( NAMED_UNIT ( * ) SI_UNIT ( $, .STERADIAN. ) SOLID_ANGLE_UNIT ( ) );
#7811=PRESENTATION_STYLE_ASSIGNMENT (( #75797 ) ) ;
#7813=FILL_AREA_STYLE_COLOUR ( '', #38330 ) ;
#7817=ORIENTED_EDGE ( 'NONE', *, *, #620, .F. ) ;
#7818=DIRECTION ( 'NONE',  ( -0.000000000000000000, 0.000000000000000000, 1.000000000000000000 ) ) ;
#7831=CYLINDRICAL_SURFACE ( 'NONE', #10129, 0.2500000000000002220 ) ;
#7842=CARTESIAN_POINT ( 'NONE',  ( 4.130000000000000782, 1.019547802438464545, -2.500000000000000000 ) ) ;
#7850=DIRECTION ( 'NONE',  ( 1.000000000000000000, 0.000000000000000000, 0.000000000000000000 ) ) ;
#7854=CARTESIAN_POINT ( 'NONE',  ( -3.750000000000000000, 78.07179676972445748, 4.000000000000000000 ) ) ;
#7859=CARTESIAN_POINT ( 'NONE',  ( -8.330963134902997780, -7.272696214962663497, -4.000000000000000000 ) ) ;
#7863=ORIENTED_EDGE ( 'NONE', *, *, #77918, .F. ) ;
#7866=FACE_OUTER_BOUND ( 'NONE', #93030, .T. ) ;
#7874=ORIENTED_EDGE ( 'NONE', *, *, #63870, .F. ) ;
#7875=DIRECTION ( 'NONE',  ( -0.000000000000000000, -0.000000000000000000, -1.000000000000000000 ) ) ;
#7876=CARTESIAN_POINT ( 'NONE',  ( -7.909660991676054742, -4.175919252839798368, -4.000000000000000000 ) ) ;
#7887=PLANE ( 'NONE',  #68258 ) ;
#7903=ADVANCED_FACE ( 'NONE', ( #10696 ), #45523, .F. ) ;
#7911=ORIENTED_EDGE ( 'NONE', *, *, #31695, .T. ) ;
#7918=CARTESIAN_POINT ( 'NONE',  ( -7.366188783701793419, -80.69039970148938323, -4.000000000000000000 ) ) ;
#7949=CARTESIAN_POINT ( 'NONE',  ( -4.000000000000000000, 78.07179676972445748, -6.500000000000000888 ) ) ;
#7958=EDGE_CURVE ( 'NONE', #85917, #14813, #98301, .T. ) ;
#7967=CARTESIAN_POINT ( 'NONE',  ( -13.34400464406060571, 90.99713512412014893, -7.995014993563001049 ) ) ;
#7970=CARTESIAN_POINT ( 'NONE',  ( 5.678900477127609037, -28.62996443930519774, 2.500000000000000000 ) ) ;
#7982=ORIENTED_EDGE ( 'NONE', *, *, #51956, .T. ) ;
#7991=CARTESIAN_POINT ( 'NONE',  ( -9.990730578767623271, 46.91630561652144138, -2.899999999999999467 ) ) ;
#8000=ORIENTED_EDGE ( 'NONE', *, *, #13212, .F. ) ;
#8028=ORIENTED_EDGE ( 'NONE', *, *, #13420, .T. ) ;
#8033=DIRECTION ( 'NONE',  ( 1.000000000000000000, 0.000000000000000000, 0.000000000000000000 ) ) ;
#8043=ORIENTED_EDGE ( 'NONE', *, *, #9359, .F. ) ;
#8052=VECTOR ( 'NONE', #12171, 1000.000000000000114 ) ;
#8055=VERTEX_POINT ( 'NONE', #92050 ) ;
#8059=ORIENTED_EDGE ( 'NONE', *, *, #98705, .T. ) ;
#8062=ORIENTED_EDGE ( 'NONE', *, *, #48567, .T. ) ;
#8077=VECTOR ( 'NONE', #95656, 1000.000000000000000 ) ;
#8082=FACE_OUTER_BOUND ( 'NONE', #22544, .T. ) ;
#8084=ORIENTED_EDGE ( 'NONE', *, *, #87293, .F. ) ;
#8090=SURFACE_STYLE_USAGE ( .BOTH. , #7609 ) ;
#8092=CARTESIAN_POINT ( 'NONE',  ( 8.921421356237301481, 27.04185244743870697, -3.000000000000000888 ) ) ;
#8095=ORIENTED_EDGE ( 'NONE', *, *, #82686, .T. ) ;
#8102=CARTESIAN_POINT ( 'NONE',  ( -6.982525766139714207, -88.11956320875633253, -3.750000000000000000 ) ) ;
#8116=STYLED_ITEM ( 'NONE', ( #20534 ), #62435 ) ;
#8123=STYLED_ITEM ( 'NONE', ( #60741 ), #46435 ) ;
#8130=VECTOR ( 'NONE', #76000, 1000.000000000000000 ) ;
#8138=UNCERTAINTY_MEASURE_WITH_UNIT (LENGTH_MEASURE( 1.000000000000000082E-05 ), #18710, 'distance_accuracy_value', 'NONE');
#8141=VERTEX_POINT ( 'NONE', #93521 ) ;
#8147=CARTESIAN_POINT ( 'NONE',  ( -11.58433430577145273, -69.52997016218431270, 3.750000000000000000 ) ) ;
#8160=DIRECTION ( 'NONE',  ( 0.000000000000000000, 0.000000000000000000, 1.000000000000000000 ) ) ;
#8170=ADVANCED_FACE ( 'NONE', ( #63511 ), #56728, .T. ) ;
#8181=CARTESIAN_POINT ( 'NONE',  ( -6.822555938877846948, -84.39442183841865130, 2.500000000000000444 ) ) ;
#8190=VERTEX_POINT ( 'NONE', #2060 ) ;
#8191=CARTESIAN_POINT ( 'NONE',  ( 8.880000000000000782, 1.019547802438459216, 3.750000000000000000 ) ) ;
#8196=( NAMED_UNIT ( * ) SI_UNIT ( $, .STERADIAN. ) SOLID_ANGLE_UNIT ( ) );
#8216=CARTESIAN_POINT ( 'NONE',  ( -6.732636091893173358, -88.11213685669363826, 2.500000000000000000 ) ) ;
#8221=DIRECTION ( 'NONE',  ( -1.000000000000000000, 0.000000000000000000, 0.000000000000000000 ) ) ;
#8226=DIRECTION ( 'NONE',  ( 1.000000000000000000, 0.000000000000000000, 0.000000000000000000 ) ) ;
#8230=CARTESIAN_POINT ( 'NONE',  ( -10.44999999999999751, 99.99999999999998579, -8.525133428036873795 ) ) ;
#8231=( GEOMETRIC_REPRESENTATION_CONTEXT ( 3 ) GLOBAL_UNCERTAINTY_ASSIGNED_CONTEXT ( ( #57422 ) ) GLOBAL_UNIT_ASSIGNED_CONTEXT ( ( #29839, #52842, #68359 ) ) REPRESENTATION_CONTEXT ( 'NONE', 'WORKASPACE' ) );
#8250=CARTESIAN_POINT ( 'NONE',  ( -19.89999999999999858, 92.00000000000000000, -7.750000000000000000 ) ) ;
#8257=VECTOR ( 'NONE', #15038, 1000.000000000000000 ) ;
#8258=ORIENTED_EDGE ( 'NONE', *, *, #60120, .T. ) ;
#8259=VECTOR ( 'NONE', #47279, 1000.000000000000000 ) ;
#8262=CARTESIAN_POINT ( 'NONE',  ( 4.629999999999995453, 43.00000000000000711, 4.250000000000000000 ) ) ;
#8267=CARTESIAN_POINT ( 'NONE',  ( -4.249999999999994671, 43.00000000000000711, 6.500000000000000888 ) ) ;
#8275=CARTESIAN_POINT ( 'NONE',  ( -3.836050625226996580, -2.701282487337019145, 3.999999999999999112 ) ) ;
#8279=VERTEX_POINT ( 'NONE', #40037 ) ;
#8288=ORIENTED_EDGE ( 'NONE', *, *, #1056, .T. ) ;
#8291=EDGE_CURVE ( 'NONE', #8190, #31523, #34366, .T. ) ;
#8292=FILL_AREA_STYLE ('',( #92280 ) ) ;
#8300=CIRCLE ( 'NONE', #68973, 2.250000000000000444 ) ;
#8304=DIRECTION ( 'NONE',  ( 0.8070303256584299145, -0.5905099943842175847, 0.000000000000000000 ) ) ;
#8305=SURFACE_STYLE_USAGE ( .BOTH. , #93762 ) ;
#8314=CARTESIAN_POINT ( 'NONE',  ( 8.630000000000000782, 1.085138116723527427E-15, -3.750000000000000000 ) ) ;
#8325=CARTESIAN_POINT ( 'NONE',  ( 6.905507196108331414, -69.44000359822085500, -2.750000000000000000 ) ) ;
#8331=AXIS2_PLACEMENT_3D ( 'NONE', #40117, #17136, #87574 ) ;
#8339=CARTESIAN_POINT ( 'NONE',  ( -8.922167142635602843, 75.09950301435408448, 2.900000000000000355 ) ) ;
#8340=CARTESIAN_POINT ( 'NONE',  ( -9.543993260040148030, -28.01899697272886769, -4.000000000000000000 ) ) ;
#8344=EDGE_LOOP ( 'NONE', ( #17428, #66577, #67027, #73596 ) ) ;
#8362=CARTESIAN_POINT ( 'NONE',  ( 8.879999999999995453, 40.74999999999999289, -4.250000000000000000 ) ) ;
#8363=CARTESIAN_POINT ( 'NONE',  ( -0.5000000000000073275, 80.99999999999994316, 0.000000000000000000 ) ) ;
#8375=DIRECTION ( 'NONE',  ( 0.9975640502598243087, -0.06975647374412535795, 0.000000000000000000 ) ) ;
#8377=ADVANCED_FACE ( 'NONE', ( #19979 ), #50971, .T. ) ;
#8393=ORIENTED_EDGE ( 'NONE', *, *, #26467, .F. ) ;
#8395=CARTESIAN_POINT ( 'NONE',  ( 6.905642986249669768, -69.45547628558871622, 3.999999999999999556 ) ) ;
#8399=CYLINDRICAL_SURFACE ( 'NONE', #76977, 0.2500000000000002220 ) ;
#8405=AXIS2_PLACEMENT_3D ( 'NONE', #50883, #21375, #29843 ) ;
#8427=CARTESIAN_POINT ( 'NONE',  ( 8.879999999999995453, 41.24999999999999289, 4.000000000000000000 ) ) ;
#8430=DIRECTION ( 'NONE',  ( 1.000000000000000000, 0.000000000000000000, -0.000000000000000000 ) ) ;
#8433=CARTESIAN_POINT ( 'NONE',  ( 8.880000000000000782, 1.019547802438458550, 3.750000000000000000 ) ) ;
#8436=AXIS2_PLACEMENT_3D ( 'NONE', #34839, #28334, #20842 ) ;
#8441=CARTESIAN_POINT ( 'NONE',  ( 17.75000000000000711, 43.00000000000000000, -6.500000000000000888 ) ) ;
#8448=LINE ( 'NONE', #16450, #83630 ) ;
#8450=ORIENTED_EDGE ( 'NONE', *, *, #84364, .F. ) ;
#8459=MECHANICAL_DESIGN_GEOMETRIC_PRESENTATION_REPRESENTATION('',(#85112),#49989);
#8466=CARTESIAN_POINT ( 'NONE',  ( -3.999999999999994671, 43.00000000000000711, 6.250000000000000000 ) ) ;
#8473=( NAMED_UNIT ( * ) SI_UNIT ( $, .STERADIAN. ) SOLID_ANGLE_UNIT ( ) );
#8480=MECHANICAL_DESIGN_GEOMETRIC_PRESENTATION_REPRESENTATION('',(#77132),#34003);
#8490=EDGE_CURVE ( 'NONE', #83825, #875, #97483, .T. ) ;
#8498=CARTESIAN_POINT ( 'NONE',  ( -4.000000000000000000, 10.25000000000000000, -4.000000000000000000 ) ) ;
#8501=CARTESIAN_POINT ( 'NONE',  ( -3.949999999999997069, 99.99999999999998579, -8.525133428036873795 ) ) ;
#8508=DIRECTION ( 'NONE',  ( -0.000000000000000000, -1.000000000000000000, -0.000000000000000000 ) ) ;
#8520=DIRECTION ( 'NONE',  ( 1.000000000000000000, 0.000000000000000000, 0.000000000000000000 ) ) ;
#8528=CARTESIAN_POINT ( 'NONE',  ( -7.750000000000000000, 41.24999999999999289, 6.250000000000000000 ) ) ;
#8549=ORIENTED_EDGE ( 'NONE', *, *, #51059, .F. ) ;
#8565=SURFACE_STYLE_FILL_AREA ( #29696 ) ;
#8570=( NAMED_UNIT ( * ) SI_UNIT ( $, .STERADIAN. ) SOLID_ANGLE_UNIT ( ) );
#8576=EDGE_CURVE ( 'NONE', #63305, #37093, #6792, .T. ) ;
#8577=( NAMED_UNIT ( * ) PLANE_ANGLE_UNIT ( ) SI_UNIT ( $, .RADIAN. ) );
#8579=CARTESIAN_POINT ( 'NONE',  ( -18.89999999999999147, 99.99999999999998579, 7.750000000000000000 ) ) ;
#8581=ORIENTED_EDGE ( 'NONE', *, *, #97118, .T. ) ;
#8582=ORIENTED_EDGE ( 'NONE', *, *, #39884, .T. ) ;
#8595=CARTESIAN_POINT ( 'NONE',  ( 3.969999999999999751, 37.00000000000000000, 2.500000000000000000 ) ) ;
#8597=CARTESIAN_POINT ( 'NONE',  ( -7.750000000000000000, 41.24999999999999289, 6.500000000000000888 ) ) ;
#8601=CARTESIAN_POINT ( 'NONE',  ( 18.00000000000000355, 73.00000000000001421, 4.000000000000000000 ) ) ;
#8602=EDGE_CURVE ( 'NONE', #33481, #44632, #56323, .T. ) ;
#8604=AXIS2_PLACEMENT_3D ( 'NONE', #38760, #85732, #92247 ) ;
#8625=EDGE_LOOP ( 'NONE', ( #4829, #18530, #46835, #15543 ) ) ;
#8630=CARTESIAN_POINT ( 'NONE',  ( -9.206628575885845933, -19.70849028575491246, 4.000000000000000000 ) ) ;
#8640=CYLINDRICAL_SURFACE ( 'NONE', #18817, 0.2500000000000002220 ) ;
#8642=LINE ( 'NONE', #78121, #89188 ) ;
#8649=DIRECTION ( 'NONE',  ( 1.049065152435176504E-16, -1.000000000000000000, 0.000000000000000000 ) ) ;
#8651=ORIENTED_EDGE ( 'NONE', *, *, #23068, .T. ) ;
#8660=CARTESIAN_POINT ( 'NONE',  ( -6.829866546992951370, -69.52413922185967010, 2.500000000000000444 ) ) ;
#8662=CYLINDRICAL_SURFACE ( 'NONE', #17075, 0.2500000000000002220 ) ;
#8669=DIRECTION ( 'NONE',  ( -1.000000000000000000, 0.000000000000000000, 0.000000000000000000 ) ) ;
#8670=ORIENTED_EDGE ( 'NONE', *, *, #95368, .T. ) ;
#8671=CARTESIAN_POINT ( 'NONE',  ( 8.900267494636356247, -1.043573704943436598, 3.750000000000000000 ) ) ;
#8673=CARTESIAN_POINT ( 'NONE',  ( -7.199999999999996625, 99.99999999999998579, 8.000000000000000000 ) ) ;
#8677=EDGE_LOOP ( 'NONE', ( #2652, #83075, #58683 ) ) ;
#8679=DIRECTION ( 'NONE',  ( -0.000000000000000000, -0.000000000000000000, -1.000000000000000000 ) ) ;
#8707=CIRCLE ( 'NONE', #23081, 0.2500000000000002220 ) ;
#8712=ORIENTED_EDGE ( 'NONE', *, *, #655, .T. ) ;
#8719=DIRECTION ( 'NONE',  ( 1.000000000000000000, 0.000000000000000000, 0.000000000000000000 ) ) ;
#8736=EDGE_LOOP ( 'NONE', ( #90155, #44793, #34896, #92702 ) ) ;
#8738=PLANE ( 'NONE',  #53282 ) ;
#8739=CARTESIAN_POINT ( 'NONE',  ( -8.000000000000000000, 1.019547802438466100, -3.750000000000000000 ) ) ;
#8748=VECTOR ( 'NONE', #24961, 1000.000000000000000 ) ;
#8753=AXIS2_PLACEMENT_3D ( 'NONE', #11298, #41819, #27771 ) ;
#8755=CARTESIAN_POINT ( 'NONE',  ( -6.868018881922843377, -58.39307134327827953, 3.999999999996775024 ) ) ;
#8757=ORIENTED_EDGE ( 'NONE', *, *, #54271, .F. ) ;
#8767=DIRECTION ( 'NONE',  ( 0.000000000000000000, -1.000000000000000000, 0.000000000000000000 ) ) ;
#8778=FACE_OUTER_BOUND ( 'NONE', #85630, .T. ) ;
#8781=STYLED_ITEM ( 'NONE', ( #20078 ), #52424 ) ;
#8786=PRESENTATION_STYLE_ASSIGNMENT (( #8305 ) ) ;
#8798=CARTESIAN_POINT ( 'NONE',  ( -9.000000000000003553, 80.99999999999994316, 0.000000000000000000 ) ) ;
#8799=CARTESIAN_POINT ( 'NONE',  ( -10.53011945866295029, -98.59345040283277228, 3.750000000000000000 ) ) ;
#8814=PRESENTATION_STYLE_ASSIGNMENT (( #24817 ) ) ;
#8825=CARTESIAN_POINT ( 'NONE',  ( -10.79676793865326268, -44.60032227172077768, -3.750000000001800782 ) ) ;
#8829=ORIENTED_EDGE ( 'NONE', *, *, #24698, .T. ) ;
#8840=EDGE_CURVE ( 'NONE', #2418, #27580, #21205, .T. ) ;
#8842=DIRECTION ( 'NONE',  ( 6.938893903907222067E-15, 0.000000000000000000, 1.000000000000000000 ) ) ;
#8859=AXIS2_PLACEMENT_3D ( 'NONE', #75245, #8719, #76723 ) ;
#8869=ORIENTED_EDGE ( 'NONE', *, *, #12536, .F. ) ;
#8871=ORIENTED_EDGE ( 'NONE', *, *, #59734, .T. ) ;
#8894=CARTESIAN_POINT ( 'NONE',  ( -10.88853822400146676, 46.97908644289115898, 0.000000000000000000 ) ) ;
#8897=TOROIDAL_SURFACE ( 'NONE', #31234, 9.900000000000002132, 0.1000000000000000056 ) ;
#8905=CARTESIAN_POINT ( 'NONE',  ( -18.89999999999999503, 92.00000000000000000, -8.000000000000000000 ) ) ;
#8913=CARTESIAN_POINT ( 'NONE',  ( 0.000000000000000000, -97.00000000000000000, 3.750000000000000000 ) ) ;
#8915=DIRECTION ( 'NONE',  ( -0.06975647374412544122, -0.9975640502598243087, 0.000000000000000000 ) ) ;
#8917=DIRECTION ( 'NONE',  ( -1.000000000000000000, 0.000000000000000000, 0.000000000000000000 ) ) ;
#8929=CARTESIAN_POINT ( 'NONE',  ( -10.88853822400146676, 46.97908644289115898, 0.000000000000000000 ) ) ;
#8935=CARTESIAN_POINT ( 'NONE',  ( 4.655929185078333532, -8.243906417220228988, 2.750000000000000000 ) ) ;
#8937=VERTEX_POINT ( 'NONE', #64366 ) ;
#8949=ORIENTED_EDGE ( 'NONE', *, *, #6565, .T. ) ;
#8956=LINE ( 'NONE', #47930, #56057 ) ;
#8969=DIRECTION ( 'NONE',  ( -0.9975640502598257520, 0.06975647374410356982, 0.000000000000000000 ) ) ;
#8994=LINE ( 'NONE', #54485, #76168 ) ;
#9022=AXIS2_PLACEMENT_3D ( 'NONE', #57762, #72757, #11777 ) ;
#9027=VERTEX_POINT ( 'NONE', #47401 ) ;
#9044=STYLED_ITEM ( 'NONE', ( #2184 ), #72298 ) ;
#9045=EDGE_CURVE ( 'NONE', #37066, #82533, #22792, .T. ) ;
#9048=EDGE_LOOP ( 'NONE', ( #74803, #17346, #36868, #88710 ) ) ;
#9055=( LENGTH_UNIT ( ) NAMED_UNIT ( * ) SI_UNIT ( .MILLI., .METRE. ) );
#9056=DIRECTION ( 'NONE',  ( -0.000000000000000000, -0.000000000000000000, 1.000000000000000000 ) ) ;
#9066=FACE_OUTER_BOUND ( 'NONE', #94299, .T. ) ;
#9068=LINE ( 'NONE', #94041, #16017 ) ;
#9079=ADVANCED_FACE ( 'NONE', ( #7194 ), #91674, .T. ) ;
#9080=DIRECTION ( 'NONE',  ( 0.000000000000000000, 0.000000000000000000, -1.000000000000000000 ) ) ;
#9087=DIRECTION ( 'NONE',  ( -0.06975647374412544122, -0.9975640502598241977, 0.000000000000000000 ) ) ;
#9089=CARTESIAN_POINT ( 'NONE',  ( 4.629999999999994564, 43.00000000000000711, -4.000000000000000000 ) ) ;
#9103=CARTESIAN_POINT ( 'NONE',  ( 8.880000000000020322, 80.07179676972448590, -6.250000000000000000 ) ) ;
#9114=EDGE_LOOP ( 'NONE', ( #44094, #24276, #13831, #44125 ) ) ;
#9115=ORIENTED_EDGE ( 'NONE', *, *, #59622, .T. ) ;
#9120=CARTESIAN_POINT ( 'NONE',  ( -18.89999999999999503, 98.99999999999998579, -7.750000000000000000 ) ) ;
#9128=EDGE_CURVE ( 'NONE', #37577, #2183, #21709, .T. ) ;
#9132=DIRECTION ( 'NONE',  ( -1.000000000000000000, -0.000000000000000000, -0.000000000000000000 ) ) ;
#9139=SURFACE_STYLE_FILL_AREA ( #94110 ) ;
#9141=CYLINDRICAL_SURFACE ( 'NONE', #30298, 2.000000000000000888 ) ;
#9146=VERTEX_POINT ( 'NONE', #6205 ) ;
#9154=DIRECTION ( 'NONE',  ( 6.325067799096631348E-17, -2.128331934758712753E-15, 1.000000000000000000 ) ) ;
#9158=ORIENTED_EDGE ( 'NONE', *, *, #61400, .F. ) ;
#9165=CARTESIAN_POINT ( 'NONE',  ( 6.349999999999995204, -97.00000000000000000, -3.750000000000000000 ) ) ;
#9167=LINE ( 'NONE', #24185, #16468 ) ;
#9169=MECHANICAL_DESIGN_GEOMETRIC_PRESENTATION_REPRESENTATION('',(#28301),#29862);
#9171=LINE ( 'NONE', #93155, #61759 ) ;
#9182=AXIS2_PLACEMENT_3D ( 'NONE', #48387, #1936, #94379 ) ;
#9185=CARTESIAN_POINT ( 'NONE',  ( 6.935117329331200509, -80.58074665965396832, -2.750000000000000888 ) ) ;
#9203=CARTESIAN_POINT ( 'NONE',  ( 15.55000000000000071, 99.99999999999998579, -8.000000000000000000 ) ) ;
#9215=UNCERTAINTY_MEASURE_WITH_UNIT (LENGTH_MEASURE( 1.000000000000000082E-05 ), #31377, 'distance_accuracy_value', 'NONE');
#9221=CARTESIAN_POINT ( 'NONE',  ( 8.630000001796595654, -0.01508430609074851159, -4.000000000000000000 ) ) ;
#9222=CARTESIAN_POINT ( 'NONE',  ( 8.879999999999999005, 20.99999999999999645, 0.000000000000000000 ) ) ;
#9226=AXIS2_PLACEMENT_3D ( 'NONE', #28726, #67228, #37725 ) ;
#9233=UNCERTAINTY_MEASURE_WITH_UNIT (LENGTH_MEASURE( 1.000000000000000082E-05 ), #25621, 'distance_accuracy_value', 'NONE');
#9234=STYLED_ITEM ( 'NONE', ( #89550 ), #15837 ) ;
#9247=CARTESIAN_POINT ( 'NONE',  ( 18.00000000000000000, 77.07179676972447169, 4.250000000000000000 ) ) ;
#9252=ORIENTED_EDGE ( 'NONE', *, *, #92831, .F. ) ;
#9269=EDGE_LOOP ( 'NONE', ( #16063, #4130, #22269, #42755 ) ) ;
#9296=SURFACE_STYLE_FILL_AREA ( #23829 ) ;
#9301=CARTESIAN_POINT ( 'NONE',  ( -8.224651678658434051, 85.81254401277075772, 3.937446577531860559 ) ) ;
#9319=CARTESIAN_POINT ( 'NONE',  ( -8.028888469548853379, -1.053269085617737799, -4.000000000000000000 ) ) ;
#9323=VERTEX_POINT ( 'NONE', #64932 ) ;
#9326=DIRECTION ( 'NONE',  ( 0.8073289077885641429, -0.5901017155109146151, 0.000000000000000000 ) ) ;
#9336=FILL_AREA_STYLE_COLOUR ( '', #80403 ) ;
#9345=DIRECTION ( 'NONE',  ( -1.000000000000000000, 0.000000000000000000, 0.000000000000000000 ) ) ;
#9346=FILL_AREA_STYLE_COLOUR ( '', #46777 ) ;
#9350=UNCERTAINTY_MEASURE_WITH_UNIT (LENGTH_MEASURE( 1.000000000000000082E-05 ), #41081, 'distance_accuracy_value', 'NONE');
#9355=DIRECTION ( 'NONE',  ( -0.000000000000000000, -0.000000000000000000, -1.000000000000000000 ) ) ;
#9359=EDGE_CURVE ( 'NONE', #20156, #26894, #50438, .T. ) ;
#9364=MANIFOLD_SOLID_BREP ( 'Fillet10', #77781 ) ;
#9383=ORIENTED_EDGE ( 'NONE', *, *, #26758, .T. ) ;
#9394=CIRCLE ( 'NONE', #50926, 0.2500000000000002220 ) ;
#9410=SURFACE_STYLE_FILL_AREA ( #69423 ) ;
#9413=DIRECTION ( 'NONE',  ( -1.483861936729427615E-16, 1.000000000000000000, 0.000000000000000000 ) ) ;
#9414=AXIS2_PLACEMENT_3D ( 'NONE', #34830, #93373, #24901 ) ;
#9418=VERTEX_POINT ( 'NONE', #93857 ) ;
#9419=CARTESIAN_POINT ( 'NONE',  ( 6.432108699068926683, -88.20011490510430008, -2.500000000000000000 ) ) ;
#9431=CIRCLE ( 'NONE', #11005, 8.250000000000007105 ) ;
#9437=CARTESIAN_POINT ( 'NONE',  ( 11.18060183609497571, -93.00793896048890019, 3.750000000000000888 ) ) ;
#9438=EDGE_CURVE ( 'NONE', #77456, #63872, #80292, .T. ) ;
#9444=ORIENTED_EDGE ( 'NONE', *, *, #90779, .F. ) ;
#9451=CARTESIAN_POINT ( 'NONE',  ( 17.74999999999999645, 78.80384757729336798, 4.000000000000000000 ) ) ;
#9453=CARTESIAN_POINT ( 'NONE',  ( -8.900000000000002132, 80.99999999999994316, 0.000000000000000000 ) ) ;
#9454=STYLED_ITEM ( 'NONE', ( #11330 ), #14380 ) ;
#9465=ORIENTED_EDGE ( 'NONE', *, *, #1003, .F. ) ;
#9466=AXIS2_PLACEMENT_3D ( 'NONE', #14569, #91539, #75046 ) ;
#9478=ORIENTED_EDGE ( 'NONE', *, *, #60792, .F. ) ;
#9479=( LENGTH_UNIT ( ) NAMED_UNIT ( * ) SI_UNIT ( .MILLI., .METRE. ) );
#9480=FILL_AREA_STYLE_COLOUR ( '', #44676 ) ;
#9524=ADVANCED_FACE ( 'NONE', ( #39397 ), #86855, .F. ) ;
#9552=MECHANICAL_DESIGN_GEOMETRIC_PRESENTATION_REPRESENTATION('',(#70236),#35084);
#9563=ORIENTED_EDGE ( 'NONE', *, *, #50053, .T. ) ;
#9572=COLOUR_RGB ( '', 0.40784314, 0.44705882, 0.49803922) ;
#9581=CARTESIAN_POINT ( 'NONE',  ( -11.26387636255947733, -65.37812658113172404, 3.999999999999999112 ) ) ;
#9590=FACE_OUTER_BOUND ( 'NONE', #64282, .T. ) ;
#9596=DIRECTION ( 'NONE',  ( 1.000000000000000000, 0.000000000000000000, -0.000000000000000000 ) ) ;
#9605=LINE ( 'NONE', #30614, #49712 ) ;
#9608=EDGE_CURVE ( 'NONE', #981, #15638, #26831, .T. ) ;
#9625=AXIS2_PLACEMENT_3D ( 'NONE', #2119, #24610, #15636 ) ;
#9629=DIRECTION ( 'NONE',  ( 1.000000000000000000, 0.000000000000000000, 0.000000000000000000 ) ) ;
#9631=( NAMED_UNIT ( * ) SI_UNIT ( $, .STERADIAN. ) SOLID_ANGLE_UNIT ( ) );
#9632=CIRCLE ( 'NONE', #31947, 0.2499999999999997780 ) ;
#9657=CARTESIAN_POINT ( 'NONE',  ( -8.099999999999999645, 80.99999999999994316, -2.900000000000000799 ) ) ;
#9661=ORIENTED_EDGE ( 'NONE', *, *, #69352, .F. ) ;
#9662=SURFACE_SIDE_STYLE ('',( #39681 ) ) ;
#9665=SURFACE_STYLE_USAGE ( .BOTH. , #16680 ) ;
#9666=FACE_OUTER_BOUND ( 'NONE', #6308, .T. ) ;
#9668=CARTESIAN_POINT ( 'NONE',  ( 8.880000000000020322, 79.82179676972448590, 6.500000000000000888 ) ) ;
#9673=DIRECTION ( 'NONE',  ( 6.938893903907222067E-15, 0.000000000000000000, 1.000000000000000000 ) ) ;
#9678=CARTESIAN_POINT ( 'NONE',  ( 4.380000000000002558, 1.019547802438462547, -2.750000000000000000 ) ) ;
#9679=VECTOR ( 'NONE', #57666, 1000.000000000000000 ) ;
#9680=ORIENTED_EDGE ( 'NONE', *, *, #49895, .T. ) ;
#9684=AXIS2_PLACEMENT_3D ( 'NONE', #11424, #95420, #65399 ) ;
#9688=CARTESIAN_POINT ( 'NONE',  ( 4.219999999999999751, 37.00000000000000000, 2.750000000000000000 ) ) ;
#9727=EDGE_CURVE ( 'NONE', #21688, #71973, #35816, .T. ) ;
#9730=AXIS2_PLACEMENT_3D ( 'NONE', #15976, #46949, #63431 ) ;
#9736=DIRECTION ( 'NONE',  ( 1.000000000000000000, -6.938893903907221278E-15, -6.938893903907221278E-15 ) ) ;
#9742=DIRECTION ( 'NONE',  ( -0.000000000000000000, -1.000000000000000000, -0.000000000000000000 ) ) ;
#9743=CARTESIAN_POINT ( 'NONE',  ( 17.99999999999999645, 78.09931407715556873, 3.985200473436547597 ) ) ;
#9746=CARTESIAN_POINT ( 'NONE',  ( -5.331138373813207210, -28.69357394137744421, 3.749999999999193534 ) ) ;
#9756=CARTESIAN_POINT ( 'NONE',  ( 15.00000000000000000, 77.07179676972447169, -6.250000000000000000 ) ) ;
#9762=B_SPLINE_CURVE_WITH_KNOTS ( 'NONE', 3,
 ( #65596, #43596, #28097, #97128, #57609, #57118, #28598, #74084, #5617, #59087, #51604, #34605, #6103, #89595, #87615, #64605, #21105, #82088, #13599, #44079, #74588, #19617 ),
 .UNSPECIFIED., .F., .F.,
 ( 4, 2, 2, 2, 2, 2, 2, 2, 2, 2, 4 ),
 ( -6.000000000051943759E-08, 0.002788756707268867478, 0.005577573414537735468, 0.01115520682907547058, 0.02231047365815094080, 0.03346574048722640582, 0.04462100731630187084, 0.06693154097445282169, 0.07808680780352829365, 0.08366444121806604350, 0.08924207463260379336 ),
 .UNSPECIFIED. ) ;
#9766=VECTOR ( 'NONE', #2853, 1000.000000000000000 ) ;
#9770=ORIENTED_EDGE ( 'NONE', *, *, #23064, .T. ) ;
#9774=DIRECTION ( 'NONE',  ( 1.000000000000000000, 0.000000000000000000, 0.000000000000000000 ) ) ;
#9777=CARTESIAN_POINT ( 'NONE',  ( -9.024359497401759356, 75.07164295747612925, -2.900000000000000799 ) ) ;
#9785=DIRECTION ( 'NONE',  ( -2.107602052970795044E-16, 1.000000000000000000, 0.000000000000000000 ) ) ;
#9790=LINE ( 'NONE', #40289, #8259 ) ;
#9794=CIRCLE ( 'NONE', #72016, 0.2500000000000002220 ) ;
#9808=( NAMED_UNIT ( * ) PLANE_ANGLE_UNIT ( ) SI_UNIT ( $, .RADIAN. ) );
#9814=STYLED_ITEM ( 'NONE', ( #58621 ), #33558 ) ;
#9815=CARTESIAN_POINT ( 'NONE',  ( 18.00000000000000711, 77.35013740655264769, -4.131316298316595415 ) ) ;
#9816=DIRECTION ( 'NONE',  ( 0.000000000000000000, 0.000000000000000000, -1.000000000000000000 ) ) ;
#9821=VECTOR ( 'NONE', #17961, 1000.000000000000000 ) ;
#9823=CARTESIAN_POINT ( 'NONE',  ( 7.079515573063597245, -88.00917032380692717, -3.749999999999998668 ) ) ;
#9828=CARTESIAN_POINT ( 'NONE',  ( 8.629999999999995453, 41.24999999999999289, -6.500000000000000888 ) ) ;
#9837=SURFACE_STYLE_USAGE ( .BOTH. , #62823 ) ;
#9861=PLANE ( 'NONE',  #95068 ) ;
#9912=CARTESIAN_POINT ( 'NONE',  ( -11.42264910390652233, -90.33240963618720798, 3.750000000000000888 ) ) ;
#9920=VERTEX_POINT ( 'NONE', #39286 ) ;
#9923=CARTESIAN_POINT ( 'NONE',  ( -9.000000000000001776, 80.99999999999994316, -2.900000000000000799 ) ) ;
#9934=CARTESIAN_POINT ( 'NONE',  ( 6.507545146407271552, -58.30914921483925895, 2.500000000000000000 ) ) ;
#9949=CARTESIAN_POINT ( 'NONE',  ( -6.030006457173053391, -39.79017371240020395, -2.499999999999193534 ) ) ;
#9953=CARTESIAN_POINT ( 'NONE',  ( 4.380000000000001670, 1.019547802438464768, -4.000000000000000000 ) ) ;
#9954=CARTESIAN_POINT ( 'NONE',  ( 3.969999999999999751, 36.75000000000000000, -4.000000000000000000 ) ) ;
#9957=CARTESIAN_POINT ( 'NONE',  ( 17.75000000000000355, 73.00000000000001421, -6.250000000000000000 ) ) ;
#9981=CARTESIAN_POINT ( 'NONE',  ( -9.000000000000001776, 80.99999999999994316, 0.000000000000000000 ) ) ;
#9986=CIRCLE ( 'NONE', #91406, 1.000000000000000888 ) ;
#9992=( GEOMETRIC_REPRESENTATION_CONTEXT ( 3 ) GLOBAL_UNCERTAINTY_ASSIGNED_CONTEXT ( ( #70115 ) ) GLOBAL_UNIT_ASSIGNED_CONTEXT ( ( #15972, #69959, #46462 ) ) REPRESENTATION_CONTEXT ( 'NONE', 'WORKASPACE' ) );
#9996=MECHANICAL_DESIGN_GEOMETRIC_PRESENTATION_REPRESENTATION('',(#64270),#62636);
#10001=CARTESIAN_POINT ( 'NONE',  ( 9.779999999999990479, 20.99999999999999645, 0.000000000000000000 ) ) ;
#10007=CARTESIAN_POINT ( 'NONE',  ( -8.899065713163235358, -15.58770999055384365, -3.750000000000000888 ) ) ;
#10013=ORIENTED_EDGE ( 'NONE', *, *, #12166, .T. ) ;
#10022=CIRCLE ( 'NONE', #56337, 0.2500000000000002220 ) ;
#10040=VERTEX_POINT ( 'NONE', #39957 ) ;
#10041=ORIENTED_EDGE ( 'NONE', *, *, #10407, .T. ) ;
#10053=CIRCLE ( 'NONE', #22832, 6.599999999999995204 ) ;
#10072=LINE ( 'NONE', #64029, #75773 ) ;
#10081=DIRECTION ( 'NONE',  ( 0.000000000000000000, -0.000000000000000000, 1.000000000000000000 ) ) ;
#10082=DIRECTION ( 'NONE',  ( -0.000000000000000000, -0.000000000000000000, -1.000000000000000000 ) ) ;
#10084=AXIS2_PLACEMENT_3D ( 'NONE', #52202, #15701, #45687 ) ;
#10088=ADVANCED_FACE ( 'NONE', ( #2478 ), #32445, .T. ) ;
#10092=CARTESIAN_POINT ( 'NONE',  ( -6.030735108402915934, -39.80307983730808274, -3.749999999999999556 ) ) ;
#10093=FILL_AREA_STYLE_COLOUR ( '', #28866 ) ;
#10100=CARTESIAN_POINT ( 'NONE',  ( 8.879999999999991900, 27.04366094290857347, 2.900000000000000355 ) ) ;
#10109=CARTESIAN_POINT ( 'NONE',  ( 8.630000000000000782, 1.019547802438458550, -4.000000000000000000 ) ) ;
#10110=VERTEX_POINT ( 'NONE', #48434 ) ;
#10124=COLOUR_RGB ( '', 0.09019608, 0.27058824, 0.51372549) ;
#10127=ORIENTED_EDGE ( 'NONE', *, *, #79404, .T. ) ;
#10129=AXIS2_PLACEMENT_3D ( 'NONE', #8314, #67329, #98355 ) ;
#10131=DIRECTION ( 'NONE',  ( -0.000000000000000000, -0.000000000000000000, 1.000000000000000000 ) ) ;
#10139=DIRECTION ( 'NONE',  ( 1.000000000000000000, 0.000000000000000000, 0.000000000000000000 ) ) ;
#10142=ORIENTED_EDGE ( 'NONE', *, *, #76054, .F. ) ;
#10152=( GEOMETRIC_REPRESENTATION_CONTEXT ( 3 ) GLOBAL_UNCERTAINTY_ASSIGNED_CONTEXT ( ( #53115 ) ) GLOBAL_UNIT_ASSIGNED_CONTEXT ( ( #82735, #62186, #2219 ) ) REPRESENTATION_CONTEXT ( 'NONE', 'WORKASPACE' ) );
#10154=ORIENTED_EDGE ( 'NONE', *, *, #54141, .T. ) ;
#10156=CARTESIAN_POINT ( 'NONE',  ( -3.887834249412648546, -8.254296980873792933, 2.750000000000000888 ) ) ;
#10178=EDGE_CURVE ( 'NONE', #59059, #43266, #39477, .T. ) ;
#10187=VECTOR ( 'NONE', #76500, 1000.000000000000114 ) ;
#10196=DIRECTION ( 'NONE',  ( -1.000000000000000000, 0.000000000000000000, 0.000000000000000000 ) ) ;
#10203=ORIENTED_EDGE ( 'NONE', *, *, #22207, .F. ) ;
#10210=UNCERTAINTY_MEASURE_WITH_UNIT (LENGTH_MEASURE( 1.000000000000000082E-05 ), #67804, 'distance_accuracy_value', 'NONE');
#10214=VERTEX_POINT ( 'NONE', #35890 ) ;
#10226=FILL_AREA_STYLE ('',( #79697 ) ) ;
#10228=ORIENTED_EDGE ( 'NONE', *, *, #15758, .F. ) ;
#10241=CARTESIAN_POINT ( 'NONE',  ( 6.284583270191198778, -88.40194713205143273, 3.750000000000000000 ) ) ;
#10244=DIRECTION ( 'NONE',  ( 0.9961946980917453232, -0.08715574274766037244, 0.000000000000000000 ) ) ;
#10253=( NAMED_UNIT ( * ) PLANE_ANGLE_UNIT ( ) SI_UNIT ( $, .RADIAN. ) );
#10272=CARTESIAN_POINT ( 'NONE',  ( 8.629999999999995453, 43.00000000000000000, -6.500000000000000888 ) ) ;
#10279=DIRECTION ( 'NONE',  ( 1.000000000000000000, 0.000000000000000000, 0.000000000000000000 ) ) ;
#10294=CARTESIAN_POINT ( 'NONE',  ( -9.247107438774047949, 88.00886336720424197, 5.024692236534948009 ) ) ;
#10298=ORIENTED_EDGE ( 'NONE', *, *, #48882, .T. ) ;
#10303=FACE_OUTER_BOUND ( 'NONE', #8736, .T. ) ;
#10325=AXIS2_PLACEMENT_3D ( 'NONE', #98524, #29977, #21019 ) ;
#10327=EDGE_CURVE ( 'NONE', #17231, #47751, #16601, .T. ) ;
#10334=CARTESIAN_POINT ( 'NONE',  ( 11.08992015851877078, -87.81706477658710241, -4.000000000000000888 ) ) ;
#10343=STYLED_ITEM ( 'NONE', ( #41809 ), #7167 ) ;
#10348=DIRECTION ( 'NONE',  ( 0.06975647374410356982, 0.9975640502598257520, -0.000000000000000000 ) ) ;
#10358=ORIENTED_EDGE ( 'NONE', *, *, #12845, .F. ) ;
#10366=B_SPLINE_CURVE_WITH_KNOTS ( 'NONE', 3,
 ( #35875, #72035, #34022, #95025, #57030, #2097, #18064, #25573, #66367, #96903, #94052, #49521, #81378, #63057, #93554, #40569, #43372, #55570 ),
 .UNSPECIFIED., .F., .F.,
 ( 4, 2, 2, 2, 2, 2, 2, 2, 4 ),
 ( 0.0005459035990385047079, 0.001906373199480198037, 0.003266842799921891582, 0.004627312400363584911, 0.005987782000805278240, 0.007348251601246971569, 0.008708721201688664898, 0.01006919080213035909, 0.01142966040257205156 ),
 .UNSPECIFIED. ) ;
#10370=CARTESIAN_POINT ( 'NONE',  ( 7.850000000000003197, 98.49999999999998579, 8.000000000000000000 ) ) ;
#10385=( GEOMETRIC_REPRESENTATION_CONTEXT ( 3 ) GLOBAL_UNCERTAINTY_ASSIGNED_CONTEXT ( ( #50490 ) ) GLOBAL_UNIT_ASSIGNED_CONTEXT ( ( #65354, #91821, #6842 ) ) REPRESENTATION_CONTEXT ( 'NONE', 'WORKASPACE' ) );
#10388=ORIENTED_EDGE ( 'NONE', *, *, #89192, .F. ) ;
#10389=STYLED_ITEM ( 'NONE', ( #91815 ), #85238 ) ;
#10399=CARTESIAN_POINT ( 'NONE',  ( -10.88853822400146676, 46.97908644289115898, 3.000000000000000000 ) ) ;
#10400=DIRECTION ( 'NONE',  ( -0.000000000000000000, -0.000000000000000000, -1.000000000000000000 ) ) ;
#10403=LINE ( 'NONE', #63392, #29797 ) ;
#10407=EDGE_CURVE ( 'NONE', #15068, #83910, #5317, .T. ) ;
#10410=PLANE ( 'NONE',  #39299 ) ;
#10428=CARTESIAN_POINT ( 'NONE',  ( 10.72261300086672797, -40.29758884457105239, 3.750000000000000444 ) ) ;
#10434=CIRCLE ( 'NONE', #96663, 0.2500000000000002220 ) ;
#10441=DIRECTION ( 'NONE',  ( -1.000000000000000000, 0.000000000000000000, -1.734723475976805517E-15 ) ) ;
#10444=DIRECTION ( 'NONE',  ( 1.000000000000000000, 0.000000000000000000, 0.000000000000000000 ) ) ;
#10482=STYLED_ITEM ( 'NONE', ( #51125 ), #5997 ) ;
#10484=CARTESIAN_POINT ( 'NONE',  ( 4.219999999999999751, 36.75000000000000000, -4.000000000000000000 ) ) ;
#10489=CARTESIAN_POINT ( 'NONE',  ( -10.57647196447611648, -40.47791205351722965, -3.749999999999999556 ) ) ;
#10537=ORIENTED_EDGE ( 'NONE', *, *, #42020, .F. ) ;
#10558=ADVANCED_FACE ( 'NONE', ( #73297 ), #34296, .T. ) ;
#10564=CARTESIAN_POINT ( 'NONE',  ( -11.01424773205765817, -93.41215259629041157, -4.000000000000000888 ) ) ;
#10565=VECTOR ( 'NONE', #17594, 1000.000000000000000 ) ;
#10566=CIRCLE ( 'NONE', #66444, 3.940000000000000835 ) ;
#10568=FACE_OUTER_BOUND ( 'NONE', #83860, .T. ) ;
#10572=LINE ( 'NONE', #3088, #10565 ) ;
#10573=CARTESIAN_POINT ( 'NONE',  ( 11.24699797944280100, 54.09857164847241506, 0.000000000000000000 ) ) ;
#10595=AXIS2_PLACEMENT_3D ( 'NONE', #92312, #70812, #17315 ) ;
#10602=CARTESIAN_POINT ( 'NONE',  ( -13.34397673082797020, 90.99712473415623037, 7.994997298710761591 ) ) ;
#10608=FILL_AREA_STYLE_COLOUR ( '', #22051 ) ;
#10613=DIRECTION ( 'NONE',  ( 0.000000000000000000, 0.000000000000000000, -1.000000000000000000 ) ) ;
#10616=ORIENTED_EDGE ( 'NONE', *, *, #50019, .T. ) ;
#10623=EDGE_CURVE ( 'NONE', #22589, #16383, #13792, .T. ) ;
#10624=CIRCLE ( 'NONE', #23411, 4.250000000000001776 ) ;
#10625=TOROIDAL_SURFACE ( 'NONE', #12244, 7.250000000000002665, 0.2500000000000000000 ) ;
#10626=TOROIDAL_SURFACE ( 'NONE', #5837, 1.750000000000000888, 0.2500000000000000000 ) ;
#10640=FACE_OUTER_BOUND ( 'NONE', #9048, .T. ) ;
#10642=CARTESIAN_POINT ( 'NONE',  ( 10.93736952808811047, -97.13260119838979278, 3.750000000000000000 ) ) ;
#10664=VECTOR ( 'NONE', #83581, 999.9999999999998863 ) ;
#10665=ORIENTED_EDGE ( 'NONE', *, *, #20667, .F. ) ;
#10667=DIRECTION ( 'NONE',  ( -0.000000000000000000, 0.000000000000000000, 1.000000000000000000 ) ) ;
#10671=LINE ( 'NONE', #41185, #16923 ) ;
#10679=CARTESIAN_POINT ( 'NONE',  ( -3.750000000000000000, 0.000000000000000000, -2.500000000000000000 ) ) ;
#10690=ORIENTED_EDGE ( 'NONE', *, *, #90022, .T. ) ;
#10692=STYLED_ITEM ( 'NONE', ( #65994 ), #38400 ) ;
#10696=FACE_OUTER_BOUND ( 'NONE', #83160, .T. ) ;
#10702=CARTESIAN_POINT ( 'NONE',  ( 8.880000000000000782, -0.01161165531298087583, -3.750000000000000000 ) ) ;
#10712=ORIENTED_EDGE ( 'NONE', *, *, #32274, .T. ) ;
#10727=DIRECTION ( 'NONE',  ( 0.000000000000000000, 0.000000000000000000, -1.000000000000000000 ) ) ;
#10730=CARTESIAN_POINT ( 'NONE',  ( -6.581680125707231710, -88.31141629936868753, 2.750000000000000000 ) ) ;
#10740=EDGE_CURVE ( 'NONE', #30525, #70565, #16802, .T. ) ;
#10742=B_SPLINE_CURVE_WITH_KNOTS ( 'NONE', 3,
 ( #43523, #67024, #21532, #67523, #60004, #90498 ),
 .UNSPECIFIED., .F., .F.,
 ( 4, 2, 4 ),
 ( 0.000000000000000000, 0.0002100574294231419411, 0.0004201148588462838823 ),
 .UNSPECIFIED. ) ;
#10746=VERTEX_POINT ( 'NONE', #68317 ) ;
#10756=DIRECTION ( 'NONE',  ( -1.000000000000000000, -0.000000000000000000, -0.000000000000000000 ) ) ;
#10768=LINE ( 'NONE', #69304, #56290 ) ;
#10774=FILL_AREA_STYLE ('',( #80242 ) ) ;
#10801=EDGE_CURVE ( 'NONE', #11027, #105, #24802, .T. ) ;
#10808=CARTESIAN_POINT ( 'NONE',  ( 8.979999999999991545, 27.03929484861771826, -3.000000000000000000 ) ) ;
#10821=AXIS2_PLACEMENT_3D ( 'NONE', #81189, #72685, #12194 ) ;
#10826=( NAMED_UNIT ( * ) SI_UNIT ( $, .STERADIAN. ) SOLID_ANGLE_UNIT ( ) );
#10828=PRESENTATION_STYLE_ASSIGNMENT (( #56808 ) ) ;
#10832=CIRCLE ( 'NONE', #49140, 0.2500000000000002220 ) ;
#10845=CARTESIAN_POINT ( 'NONE',  ( 8.879999999999991900, 76.07179676972447169, 6.500000000000000888 ) ) ;
#10849=EDGE_LOOP ( 'NONE', ( #19368, #11104, #75249, #13473 ) ) ;
#10850=EDGE_CURVE ( 'NONE', #18240, #32841, #31277, .T. ) ;
#10852=ORIENTED_EDGE ( 'NONE', *, *, #72663, .F. ) ;
#10855=EDGE_LOOP ( 'NONE', ( #84912, #81070, #76426, #78136 ) ) ;
#10869=CARTESIAN_POINT ( 'NONE',  ( -15.00000000000004974, 91.25000000000000000, 8.000000000000000000 ) ) ;
#10882=ORIENTED_EDGE ( 'NONE', *, *, #35785, .F. ) ;
#10892=STYLED_ITEM ( 'NONE', ( #95813 ), #59069 ) ;
#10897=AXIS2_PLACEMENT_3D ( 'NONE', #8528, #23049, #2032 ) ;
#10898=B_SPLINE_CURVE_WITH_KNOTS ( 'NONE', 3,
 ( #16171, #18504, #48994, #61644, #77151, #69662, #79504, #11003, #64476, #23690, #26488, #56983, #23194, #87488, #49479, #8660, #68682, #210, #53668, #8181, #38678, #69178 ),
 .UNSPECIFIED., .F., .F.,
 ( 4, 2, 2, 2, 2, 2, 2, 2, 2, 2, 4 ),
 ( 0.000000000000000000, 0.002788651922846089107, 0.005577303845692178214, 0.01115460769138435643, 0.02230921538276871285, 0.03346382307415306928, 0.04461843076553742571, 0.06692764614830616632, 0.07808225383969051581, 0.08365955768538271831, 0.08923686153107489305 ),
 .UNSPECIFIED. ) ;
#10899=SURFACE_SIDE_STYLE ('',( #17911 ) ) ;
#10911=CARTESIAN_POINT ( 'NONE',  ( 4.600000000000003197, 98.49999999999998579, -8.525133428036873795 ) ) ;
#10923=LINE ( 'NONE', #63904, #8748 ) ;
#10924=CARTESIAN_POINT ( 'NONE',  ( -3.770608837557338333, -6.399801140514261633, -2.750000000000403233 ) ) ;
#10944=CIRCLE ( 'NONE', #49263, 1.249999999999987121 ) ;
#10950=ORIENTED_EDGE ( 'NONE', *, *, #34284, .F. ) ;
#10960=EDGE_LOOP ( 'NONE', ( #92524, #38406, #4272, #9478 ) ) ;
#10964=DIRECTION ( 'NONE',  ( 0.000000000000000000, 0.000000000000000000, -1.000000000000000000 ) ) ;
#10965=AXIS2_PLACEMENT_3D ( 'NONE', #49244, #43211, #4743 ) ;
#10969=EDGE_CURVE ( 'NONE', #52027, #91180, #50600, .T. ) ;
#11003=CARTESIAN_POINT ( 'NONE',  ( -4.010384638568478266, -13.83464189901984120, 2.500000000000000444 ) ) ;
#11005=AXIS2_PLACEMENT_3D ( 'NONE', #25233, #17720, #23757 ) ;
#11013=ORIENTED_EDGE ( 'NONE', *, *, #94952, .F. ) ;
#11017=EDGE_LOOP ( 'NONE', ( #57674, #44219, #55817 ) ) ;
#11018=DIRECTION ( 'NONE',  ( 0.000000000000000000, -7.806255641895625614E-15, -1.000000000000000000 ) ) ;
#11023=COLOUR_RGB ( '', 0.08235294, 0.09019608, 0.10196078) ;
#11027=VERTEX_POINT ( 'NONE', #66082 ) ;
#11056=CARTESIAN_POINT ( 'NONE',  ( -10.67057496978640252, -97.55820424041962724, -4.000000000000000000 ) ) ;
#11063=DIRECTION ( 'NONE',  ( -0.000000000000000000, -1.000000000000000000, -0.000000000000000000 ) ) ;
#11069=FILL_AREA_STYLE_COLOUR ( '', #32145 ) ;
#11081=CARTESIAN_POINT ( 'NONE',  ( -3.750000000000000000, 36.75000000000000000, -2.750000000000000000 ) ) ;
#11087=ORIENTED_EDGE ( 'NONE', *, *, #12326, .F. ) ;
#11093=CARTESIAN_POINT ( 'NONE',  ( -13.51588146042584171, 90.98610341008148339, 7.976019732132908935 ) ) ;
#11099=DIRECTION ( 'NONE',  ( 0.000000000000000000, 0.000000000000000000, -1.000000000000000000 ) ) ;
#11101=VERTEX_POINT ( 'NONE', #9777 ) ;
#11104=ORIENTED_EDGE ( 'NONE', *, *, #42890, .T. ) ;
#11125=CIRCLE ( 'NONE', #84577, 2.000000000000000000 ) ;
#11126=CARTESIAN_POINT ( 'NONE',  ( 9.779999999999990479, 20.99999999999999645, -3.000000000000000000 ) ) ;
#11129=CARTESIAN_POINT ( 'NONE',  ( 10.58840669699852199, -98.14374106289703548, 4.000000000000000000 ) ) ;
#11132=CARTESIAN_POINT ( 'NONE',  ( -3.711005778769052021, -5.293034685380286319, 3.750000000000000444 ) ) ;
#11148=ORIENTED_EDGE ( 'NONE', *, *, #65570, .T. ) ;
#11156=SURFACE_STYLE_USAGE ( .BOTH. , #58625 ) ;
#11163=CARTESIAN_POINT ( 'NONE',  ( 0.000000000000000000, 91.00000000000000000, 7.750000000000000000 ) ) ;
#11175=LINE ( 'NONE', #18693, #7309 ) ;
#11176=UNCERTAINTY_MEASURE_WITH_UNIT (LENGTH_MEASURE( 1.000000000000000082E-05 ), #16772, 'distance_accuracy_value', 'NONE');
#11191=VECTOR ( 'NONE', #66315, 1000.000000000000000 ) ;
#11216=SURFACE_SIDE_STYLE ('',( #26703 ) ) ;
#11217=ORIENTED_EDGE ( 'NONE', *, *, #55858, .F. ) ;
#11219=ORIENTED_EDGE ( 'NONE', *, *, #72465, .T. ) ;
#11230=ORIENTED_EDGE ( 'NONE', *, *, #74466, .F. ) ;
#11240=COLOUR_RGB ( '', 0.72549020, 0.75294118, 0.79215686) ;
#11245=CIRCLE ( 'NONE', #70371, 0.2500000000000002220 ) ;
#11246=EDGE_CURVE ( 'NONE', #77672, #49491, #4405, .T. ) ;
#11253=CYLINDRICAL_SURFACE ( 'NONE', #89973, 0.09999999999999982514 ) ;
#11256=TOROIDAL_SURFACE ( 'NONE', #94259, 0.7500000000000008882, 0.2500000000000000000 ) ;
#11258=CARTESIAN_POINT ( 'NONE',  ( -13.80105244023572197, 90.89655890636302615, 7.750000000000543565 ) ) ;
#11263=LINE ( 'NONE', #49744, #90179 ) ;
#11278=VECTOR ( 'NONE', #44100, 1000.000000000000000 ) ;
#11281=EDGE_CURVE ( 'NONE', #11943, #1670, #83072, .T. ) ;
#11283=AXIS2_PLACEMENT_3D ( 'NONE', #61068, #6108, #51610 ) ;
#11287=EDGE_CURVE ( 'NONE', #25163, #7091, #68077, .T. ) ;
#11290=CARTESIAN_POINT ( 'NONE',  ( -8.004649405379840488, 84.50413264541204228, -3.999860480131919527 ) ) ;
#11298=CARTESIAN_POINT ( 'NONE',  ( 3.969999999999999751, 36.75000000000000000, -3.750000000000000000 ) ) ;
#11299=SURFACE_STYLE_USAGE ( .BOTH. , #28762 ) ;
#11309=DIRECTION ( 'NONE',  ( 0.6246950475544238435, 0.7808688094430307203, 0.000000000000000000 ) ) ;
#11315=SURFACE_STYLE_USAGE ( .BOTH. , #35788 ) ;
#11330=PRESENTATION_STYLE_ASSIGNMENT (( #12800 ) ) ;
#11335=DIRECTION ( 'NONE',  ( 0.000000000000000000, -1.000000000000000000, 0.000000000000000000 ) ) ;
#11347=EDGE_LOOP ( 'NONE', ( #84778, #23603, #43347, #38791 ) ) ;
#11357=VECTOR ( 'NONE', #67869, 1000.000000000000000 ) ;
#11363=VERTEX_POINT ( 'NONE', #21594 ) ;
#11375=DIRECTION ( 'NONE',  ( -6.938893903907222067E-15, 0.000000000000000000, -1.000000000000000000 ) ) ;
#11389=STYLED_ITEM ( 'NONE', ( #58029 ), #46610 ) ;
#11396=DIRECTION ( 'NONE',  ( -0.000000000000000000, -1.000000000000000000, -0.000000000000000000 ) ) ;
#11397=AXIS2_PLACEMENT_3D ( 'NONE', #93589, #40606, #34056 ) ;
#11402=CARTESIAN_POINT ( 'NONE',  ( 11.10714268220738354, -52.69759663682445705, 3.750000000000000000 ) ) ;
#11408=EDGE_CURVE ( 'NONE', #33129, #96487, #598, .T. ) ;
#11409=EDGE_CURVE ( 'NONE', #79587, #8141, #42644, .T. ) ;
#11411=CARTESIAN_POINT ( 'NONE',  ( -3.500000001558553286, 0.09224605988788428523, -2.499999999999595879 ) ) ;
#11418=CARTESIAN_POINT ( 'NONE',  ( 6.575338752097509065, -50.90849809615561838, -3.999999999999999556 ) ) ;
#11424=CARTESIAN_POINT ( 'NONE',  ( -19.00000000000000000, 75.76920769491739804, -2.900000000000000799 ) ) ;
#11442=LINE ( 'NONE', #87438, #78845 ) ;
#11450=VERTEX_POINT ( 'NONE', #1069 ) ;
#11461=FACE_OUTER_BOUND ( 'NONE', #34534, .T. ) ;
#11466=CARTESIAN_POINT ( 'NONE',  ( -11.07344383391687259, -96.04710479529198608, -3.750000000000000888 ) ) ;
#11484=CARTESIAN_POINT ( 'NONE',  ( -3.750000000000000000, 36.75000000000000000, 2.500000000000000000 ) ) ;
#11487=ORIENTED_EDGE ( 'NONE', *, *, #35113, .T. ) ;
#11495=CARTESIAN_POINT ( 'NONE',  ( 8.879999999999991900, 76.07179676972447169, 6.250000000000000000 ) ) ;
#11513=ADVANCED_FACE ( 'NONE', ( #55018 ), #33011, .T. ) ;
#11525=ORIENTED_EDGE ( 'NONE', *, *, #18796, .F. ) ;
#11537=DIRECTION ( 'NONE',  ( 0.000000000000000000, 0.000000000000000000, 1.000000000000000000 ) ) ;
#11540=CARTESIAN_POINT ( 'NONE',  ( 0.000000000000000000, -97.00000000000000000, -3.750000000000000000 ) ) ;
#11570=DIRECTION ( 'NONE',  ( -1.000000000000000000, 0.000000000000000000, 0.000000000000000000 ) ) ;
#11571=DIRECTION ( 'NONE',  ( -0.9975640502598243087, 0.06975647374412544122, 0.000000000000000000 ) ) ;
#11573=ORIENTED_EDGE ( 'NONE', *, *, #51593, .T. ) ;
#11588=LINE ( 'NONE', #50080, #31643 ) ;
#11590=SURFACE_SIDE_STYLE ('',( #35569 ) ) ;
#11598=ORIENTED_EDGE ( 'NONE', *, *, #17411, .T. ) ;
#11599=MECHANICAL_DESIGN_GEOMETRIC_PRESENTATION_REPRESENTATION('',(#57913),#61135);
#11612=VECTOR ( 'NONE', #33566, 1000.000000000000000 ) ;
#11613=ORIENTED_EDGE ( 'NONE', *, *, #4119, .F. ) ;
#11615=ORIENTED_EDGE ( 'NONE', *, *, #9438, .T. ) ;
#11616=CARTESIAN_POINT ( 'NONE',  ( 10.47195283036333180, -40.28639508448244300, 4.000000000000000000 ) ) ;
#11618=DIRECTION ( 'NONE',  ( 1.000000000000000000, 1.049065152435176504E-16, -0.000000000000000000 ) ) ;
#11621=CARTESIAN_POINT ( 'NONE',  ( -7.045329894599615450, -66.66420243593404393, 3.750000000000000444 ) ) ;
#11623=CARTESIAN_POINT ( 'NONE',  ( -14.89999999999999680, 98.49999999999998579, -8.525133428036873795 ) ) ;
#11625=DIRECTION ( 'NONE',  ( 0.000000000000000000, 1.000000000000000000, -0.000000000000000000 ) ) ;
#11639=AXIS2_PLACEMENT_3D ( 'NONE', #74193, #5726, #34720 ) ;
#11659=DIRECTION ( 'NONE',  ( 0.000000000000000000, 0.000000000000000000, 1.000000000000000000 ) ) ;
#11672=AXIS2_PLACEMENT_3D ( 'NONE', #42613, #35600, #12600 ) ;
#11678=AXIS2_PLACEMENT_3D ( 'NONE', #65133, #27138, #88137 ) ;
#11680=CARTESIAN_POINT ( 'NONE',  ( 6.878063601867475008, -66.29791949882819324, 3.750000000000001776 ) ) ;
#11686=AXIS2_PLACEMENT_3D ( 'NONE', #62277, #32271, #40288 ) ;
#11715=LINE ( 'NONE', #43192, #1723 ) ;
#11719=EDGE_LOOP ( 'NONE', ( #32422, #4105, #20334, #75297 ) ) ;
#11742=CARTESIAN_POINT ( 'NONE',  ( 3.969999999999999751, 37.00000000000000000, -3.750000000000000000 ) ) ;
#11748=DIRECTION ( 'NONE',  ( -1.000000000000000000, 0.000000000000000000, -0.000000000000000000 ) ) ;
#11762=CARTESIAN_POINT ( 'NONE',  ( 6.934003561272409577, -73.15726776819576571, 2.750000000000000888 ) ) ;
#11765=DIRECTION ( 'NONE',  ( 1.000000000000000000, 0.000000000000000000, 6.938893903907221278E-15 ) ) ;
#11772=( NAMED_UNIT ( * ) PLANE_ANGLE_UNIT ( ) SI_UNIT ( $, .RADIAN. ) );
#11777=DIRECTION ( 'NONE',  ( 0.6246950475544237324, 0.7808688094430306093, 0.000000000000000000 ) ) ;
#11796=CARTESIAN_POINT ( 'NONE',  ( 9.479665769771463246, -19.63627307881997908, -4.000000000000000000 ) ) ;
#11798=FACE_OUTER_BOUND ( 'NONE', #90761, .T. ) ;
#11799=( LENGTH_UNIT ( ) NAMED_UNIT ( * ) SI_UNIT ( .MILLI., .METRE. ) );
#11805=( NAMED_UNIT ( * ) SI_UNIT ( $, .STERADIAN. ) SOLID_ANGLE_UNIT ( ) );
#11818=COLOUR_RGB ( '', 0.08235294, 0.09019608, 0.10196078) ;
#11821=ORIENTED_EDGE ( 'NONE', *, *, #94239, .T. ) ;
#11839=ORIENTED_EDGE ( 'NONE', *, *, #89519, .F. ) ;
#11850=EDGE_CURVE ( 'NONE', #12076, #31523, #46754, .T. ) ;
#11855=VERTEX_POINT ( 'NONE', #62734 ) ;
#11860=ORIENTED_EDGE ( 'NONE', *, *, #9608, .F. ) ;
#11870=DIRECTION ( 'NONE',  ( -1.000000000000000000, 0.000000000000000000, 0.000000000000000000 ) ) ;
#11881=( LENGTH_UNIT ( ) NAMED_UNIT ( * ) SI_UNIT ( .MILLI., .METRE. ) );
#11885=DIRECTION ( 'NONE',  ( -0.000000000000000000, 1.000000000000000000, -0.000000000000000000 ) ) ;
#11887=VECTOR ( 'NONE', #40073, 1000.000000000000000 ) ;
#11899=FILL_AREA_STYLE ('',( #49885 ) ) ;
#11901=PLANE ( 'NONE',  #41104 ) ;
#11915=CARTESIAN_POINT ( 'NONE',  ( 6.905642986249669768, -69.45547628558871622, -3.999999999999999556 ) ) ;
#11927=CIRCLE ( 'NONE', #63019, 2.899999999999999911 ) ;
#11943=VERTEX_POINT ( 'NONE', #92264 ) ;
#11944=VECTOR ( 'NONE', #45272, 1000.000000000000000 ) ;
#11961=EDGE_CURVE ( 'NONE', #25626, #70343, #23788, .T. ) ;
#11973=ADVANCED_FACE ( 'NONE', ( #79716 ), #88191, .F. ) ;
#11977=EDGE_CURVE ( 'NONE', #11450, #37577, #7628, .T. ) ;
#11982=DIRECTION ( 'NONE',  ( -0.000000000000000000, -0.000000000000000000, 1.000000000000000000 ) ) ;
#11983=EDGE_LOOP ( 'NONE', ( #69157, #33967, #8670, #67433 ) ) ;
#11995=CARTESIAN_POINT ( 'NONE',  ( 8.630000000000000782, 1.085138116723527427E-15, 4.000000000000000000 ) ) ;
#11997=EDGE_LOOP ( 'NONE', ( #97474, #92263, #43689, #21668 ) ) ;
#12006=CARTESIAN_POINT ( 'NONE',  ( -13.77306509549858760, 90.93909206156975245, -7.896286030156202784 ) ) ;
#12022=EDGE_LOOP ( 'NONE', ( #18923, #95095, #8757, #7874 ) ) ;
#12031=CARTESIAN_POINT ( 'NONE',  ( -3.638307330400850415, -8.269691488429794290, -2.500000000000000000 ) ) ;
#12046=CARTESIAN_POINT ( 'NONE',  ( -3.500000000000000888, 0.08935878030161711894, -3.750000000000001776 ) ) ;
#12058=DIRECTION ( 'NONE',  ( 3.035766082959409260E-14, 1.000000000000000000, 0.000000000000000000 ) ) ;
#12061=DIRECTION ( 'NONE',  ( 0.000000000000000000, 0.000000000000000000, 1.000000000000000000 ) ) ;
#12062=CARTESIAN_POINT ( 'NONE',  ( -3.772059543480756005, -0.8421633283344439613, -4.000000000000000000 ) ) ;
#12076=VERTEX_POINT ( 'NONE', #96206 ) ;
#12077=CARTESIAN_POINT ( 'NONE',  ( 8.979999999999991545, 21.00000000000000000, 0.000000000000000000 ) ) ;
#12081=ORIENTED_EDGE ( 'NONE', *, *, #50492, .T. ) ;
#12087=CARTESIAN_POINT ( 'NONE',  ( 9.779999999999988702, 27.00436609429084811, -3.000000000000000000 ) ) ;
#12088=AXIS2_PLACEMENT_3D ( 'NONE', #39627, #70609, #17127 ) ;
#12106=CARTESIAN_POINT ( 'NONE',  ( -7.750000000000000000, 40.99999999999999289, -6.500000000000000888 ) ) ;
#12107=AXIS2_PLACEMENT_3D ( 'NONE', #78178, #48166, #62676 ) ;
#12112=EDGE_CURVE ( 'NONE', #89066, #75564, #79484, .T. ) ;
#12113=CARTESIAN_POINT ( 'NONE',  ( -7.081429851441987999, -84.79152421822195151, 3.750000000000000444 ) ) ;
#12114=( LENGTH_UNIT ( ) NAMED_UNIT ( * ) SI_UNIT ( .MILLI., .METRE. ) );
#12124=CIRCLE ( 'NONE', #34520, 0.2500000000000002220 ) ;
#12150=DIRECTION ( 'NONE',  ( 0.9975640502598257520, -0.06975647374410356982, 0.000000000000000000 ) ) ;
#12153=COLOUR_RGB ( '', 0.09019608, 0.27058824, 0.51372549) ;
#12166=EDGE_CURVE ( 'NONE', #29547, #3599, #92261, .T. ) ;
#12171=DIRECTION ( 'NONE',  ( 0.8070303256584299145, -0.5905099943842175847, 0.000000000000000000 ) ) ;
#12177=EDGE_LOOP ( 'NONE', ( #30416, #67614, #8549, #63250 ) ) ;
#12191=CARTESIAN_POINT ( 'NONE',  ( -6.732636091893172470, -88.11213685669366669, -3.750000000000000000 ) ) ;
#12193=VERTEX_POINT ( 'NONE', #51187 ) ;
#12194=DIRECTION ( 'NONE',  ( 1.000000000000000000, 0.000000000000000000, 0.000000000000000000 ) ) ;
#12212=ORIENTED_EDGE ( 'NONE', *, *, #59192, .T. ) ;
#12230=DIRECTION ( 'NONE',  ( -0.9887436111420608853, -0.1496197561345335991, 0.000000000000000000 ) ) ;
#12234=FACE_OUTER_BOUND ( 'NONE', #14359, .T. ) ;
#12244=AXIS2_PLACEMENT_3D ( 'NONE', #71880, #18893, #77905 ) ;
#12258=LINE ( 'NONE', #74226, #21814 ) ;
#12261=FILL_AREA_STYLE_COLOUR ( '', #25031 ) ;
#12273=DIRECTION ( 'NONE',  ( 1.000000000000000000, 0.000000000000000000, 0.000000000000000000 ) ) ;
#12275=UNCERTAINTY_MEASURE_WITH_UNIT (LENGTH_MEASURE( 1.000000000000000082E-05 ), #83322, 'distance_accuracy_value', 'NONE');
#12280=ORIENTED_EDGE ( 'NONE', *, *, #46018, .F. ) ;
#12290=CARTESIAN_POINT ( 'NONE',  ( 6.284583270191197002, -88.40194713205143273, -4.000000000000000000 ) ) ;
#12292=DIRECTION ( 'NONE',  ( 0.000000000000000000, -1.000000000000000000, 0.000000000000000000 ) ) ;
#12296=UNCERTAINTY_MEASURE_WITH_UNIT (LENGTH_MEASURE( 1.000000000000000082E-05 ), #72569, 'distance_accuracy_value', 'NONE');
#12299=LINE ( 'NONE', #66785, #92326 ) ;
#12304=CARTESIAN_POINT ( 'NONE',  ( 5.129999999999995453, 43.00000000000000711, -6.250000000000000000 ) ) ;
#12309=DIRECTION ( 'NONE',  ( 0.000000000000000000, 0.000000000000000000, 1.000000000000000000 ) ) ;
#12320=CIRCLE ( 'NONE', #17125, 2.250000000000001332 ) ;
#12324=CARTESIAN_POINT ( 'NONE',  ( -3.749999999999999112, 78.07179676972445748, 4.250000000000000000 ) ) ;
#12326=EDGE_CURVE ( 'NONE', #54753, #75561, #6045, .T. ) ;
#12330=EDGE_CURVE ( 'NONE', #71973, #36998, #50715, .T. ) ;
#12339=DIRECTION ( 'NONE',  ( -0.000000000000000000, -0.000000000000000000, -1.000000000000000000 ) ) ;
#12344=CARTESIAN_POINT ( 'NONE',  ( -14.89999999999999680, 98.49999999999998579, 8.000000000000000000 ) ) ;
#12347=VECTOR ( 'NONE', #48811, 1000.000000000000114 ) ;
#12349=ORIENTED_EDGE ( 'NONE', *, *, #69083, .T. ) ;
#12378=CARTESIAN_POINT ( 'NONE',  ( 7.850000000000003197, 98.50000000000000000, -8.000000000000000000 ) ) ;
#12393=CARTESIAN_POINT ( 'NONE',  ( -7.072497013479695838, -84.40007040885043921, -2.500000000001209255 ) ) ;
#12402=CARTESIAN_POINT ( 'NONE',  ( -6.060849023604186314, -36.09672517615243237, 3.999999999999999112 ) ) ;
#12413=EDGE_CURVE ( 'NONE', #37066, #85540, #5697, .T. ) ;
#12421=CARTESIAN_POINT ( 'NONE',  ( 2.550000000000003819, 99.99999999999998579, -8.000000000000000000 ) ) ;
#12477=CARTESIAN_POINT ( 'NONE',  ( -7.124975165242272368, -78.82169502743931844, 2.750000000000000000 ) ) ;
#12484=CARTESIAN_POINT ( 'NONE',  ( 5.800000000000003375, 99.99999999999998579, -8.525133428036873795 ) ) ;
#12489=UNCERTAINTY_MEASURE_WITH_UNIT (LENGTH_MEASURE( 1.000000000000000082E-05 ), #17357, 'distance_accuracy_value', 'NONE');
#12498=DIRECTION ( 'NONE',  ( 0.000000000000000000, 1.000000000000000000, 0.000000000000000000 ) ) ;
#12506=SURFACE_STYLE_USAGE ( .BOTH. , #29462 ) ;
#12512=DIRECTION ( 'NONE',  ( 0.000000000000000000, 1.000000000000000000, 0.000000000000000000 ) ) ;
#12519=CARTESIAN_POINT ( 'NONE',  ( -3.335590168189931592, -2.700456006050038216, -2.500000000000000000 ) ) ;
#12520=COLOUR_RGB ( '', 0.40784314, 0.44705882, 0.49803922) ;
#12530=FACE_OUTER_BOUND ( 'NONE', #97549, .T. ) ;
#12536=EDGE_CURVE ( 'NONE', #27652, #69653, #87468, .T. ) ;
#12541=( LENGTH_UNIT ( ) NAMED_UNIT ( * ) SI_UNIT ( .MILLI., .METRE. ) );
#12556=ADVANCED_FACE ( 'NONE', ( #62606 ), #8640, .F. ) ;
#12557=CARTESIAN_POINT ( 'NONE',  ( -3.522141228720374162, -0.8488377518990324333, -4.000000000000000000 ) ) ;
#12558=ORIENTED_EDGE ( 'NONE', *, *, #93514, .T. ) ;
#12563=CARTESIAN_POINT ( 'NONE',  ( -13.65777738219310677, 90.97033672325892439, 7.949049539904468276 ) ) ;
#12574=DIRECTION ( 'NONE',  ( 0.000000000000000000, 1.000000000000000000, 0.000000000000000000 ) ) ;
#12583=EDGE_LOOP ( 'NONE', ( #75788, #95954, #72667, #77169 ) ) ;
#12591=DIRECTION ( 'NONE',  ( 1.000000000000000000, 0.000000000000000000, 0.000000000000000000 ) ) ;
#12594=VECTOR ( 'NONE', #9132, 1000.000000000000000 ) ;
#12596=CARTESIAN_POINT ( 'NONE',  ( -7.750000000000000000, 80.32179676972448590, 3.750000000000000000 ) ) ;
#12600=DIRECTION ( 'NONE',  ( -1.000000000000000000, 0.000000000000000000, -0.000000000000000000 ) ) ;
#12601=CARTESIAN_POINT ( 'NONE',  ( -6.560019409699617832, -50.64698701990471363, 2.750000000000000000 ) ) ;
#12603=CYLINDRICAL_SURFACE ( 'NONE', #76409, 0.2500000000000002220 ) ;
#12615=DIRECTION ( 'NONE',  ( 0.000000000000000000, -0.000000000000000000, -1.000000000000000000 ) ) ;
#12619=ORIENTED_EDGE ( 'NONE', *, *, #49798, .T. ) ;
#12625=( NAMED_UNIT ( * ) PLANE_ANGLE_UNIT ( ) SI_UNIT ( $, .RADIAN. ) );
#12629=VECTOR ( 'NONE', #67649, 1000.000000000000114 ) ;
#12634=CARTESIAN_POINT ( 'NONE',  ( -10.67057496914079096, -97.55820424040057048, -4.000000000000000000 ) ) ;
#12637=DIRECTION ( 'NONE',  ( -1.000000000000000000, 0.000000000000000000, 0.000000000000000000 ) ) ;
#12647=ADVANCED_FACE ( 'NONE', ( #24147 ), #85901, .F. ) ;
#12658=VECTOR ( 'NONE', #88805, 1000.000000000000000 ) ;
#12665=EDGE_LOOP ( 'NONE', ( #34127, #89926, #27157, #30111 ) ) ;
#12666=DIRECTION ( 'NONE',  ( 1.000000000000000000, -0.000000000000000000, 0.000000000000000000 ) ) ;
#12668=ORIENTED_EDGE ( 'NONE', *, *, #43116, .T. ) ;
#12677=DIRECTION ( 'NONE',  ( 0.8070303256584298035, -0.5905099943842175847, 0.000000000000000000 ) ) ;
#12696=VECTOR ( 'NONE', #24003, 1000.000000000000000 ) ;
#12717=DIRECTION ( 'NONE',  ( -0.000000000000000000, -0.000000000000000000, -1.000000000000000000 ) ) ;
#12718=DIRECTION ( 'NONE',  ( -0.000000000000000000, 0.000000000000000000, 1.000000000000000000 ) ) ;
#12719=CARTESIAN_POINT ( 'NONE',  ( 0.000000000000000000, 0.000000000000000000, -2.500000000000000000 ) ) ;
#12751=AXIS2_PLACEMENT_3D ( 'NONE', #91289, #98336, #29794 ) ;
#12754=DIRECTION ( 'NONE',  ( -1.483861936729427615E-16, 1.000000000000000000, -0.000000000000000000 ) ) ;
#12764=DIRECTION ( 'NONE',  ( 1.257402221000611116E-16, -1.000000000000000000, -0.000000000000000000 ) ) ;
#12765=DIRECTION ( 'NONE',  ( -1.000000000000000000, 0.000000000000000000, 0.000000000000000000 ) ) ;
#12770=ORIENTED_EDGE ( 'NONE', *, *, #23931, .T. ) ;
#12780=DIRECTION ( 'NONE',  ( 0.000000000000000000, 0.000000000000000000, -1.000000000000000000 ) ) ;
#12785=VERTEX_POINT ( 'NONE', #57086 ) ;
#12800=SURFACE_STYLE_USAGE ( .BOTH. , #58287 ) ;
#12810=TOROIDAL_SURFACE ( 'NONE', #27216, 0.5000000000000000000, 0.2500000000000000000 ) ;
#12811=PRESENTATION_STYLE_ASSIGNMENT (( #75661 ) ) ;
#12816=( GEOMETRIC_REPRESENTATION_CONTEXT ( 3 ) GLOBAL_UNCERTAINTY_ASSIGNED_CONTEXT ( ( #5433 ) ) GLOBAL_UNIT_ASSIGNED_CONTEXT ( ( #98904, #59874, #53361 ) ) REPRESENTATION_CONTEXT ( 'NONE', 'WORKASPACE' ) );
#12845=EDGE_CURVE ( 'NONE', #30525, #21081, #11588, .T. ) ;
#12852=VECTOR ( 'NONE', #2195, 1000.000000000000000 ) ;
#12861=CARTESIAN_POINT ( 'NONE',  ( -8.646548597236176192, 87.41340560412832872, -4.720830526302458807 ) ) ;
#12870=( LENGTH_UNIT ( ) NAMED_UNIT ( * ) SI_UNIT ( .MILLI., .METRE. ) );
#12876=ADVANCED_FACE ( 'NONE', ( #34076 ), #30063, .T. ) ;
#12878=EDGE_LOOP ( 'NONE', ( #24627, #86208, #50770, #28905 ) ) ;
#12880=CARTESIAN_POINT ( 'NONE',  ( -7.079903288604985079, -69.52484394646408816, -2.500000000000000000 ) ) ;
#12886=AXIS2_PLACEMENT_3D ( 'NONE', #8363, #24851, #55333 ) ;
#12890=CARTESIAN_POINT ( 'NONE',  ( 6.935087012957517949, -80.58470470491535309, -3.750000000000000000 ) ) ;
#12894=CARTESIAN_POINT ( 'NONE',  ( -3.750000000000000888, 1.019547802438465212, 4.000000000000000000 ) ) ;
#12904=VECTOR ( 'NONE', #23179, 1000.000000000000000 ) ;
#12905=CARTESIAN_POINT ( 'NONE',  ( -7.750000000000000000, 41.24999999999999289, 6.250000000000000000 ) ) ;
#12912=VERTEX_POINT ( 'NONE', #42583 ) ;
#12931=DIRECTION ( 'NONE',  ( 1.224646799147353207E-16, 1.000000000000000000, 0.000000000000000000 ) ) ;
#12935=CARTESIAN_POINT ( 'NONE',  ( 8.979999999999991545, 21.00000000000000000, -3.000000000000000000 ) ) ;
#12938=CARTESIAN_POINT ( 'NONE',  ( 18.00000000000000355, 77.07179676972445748, 4.250000000000000000 ) ) ;
#12941=EDGE_LOOP ( 'NONE', ( #73568, #50893, #81148 ) ) ;
#12966=CARTESIAN_POINT ( 'NONE',  ( -6.356892395138682872, -50.94284410517786910, 2.500000000000000000 ) ) ;
#12984=FACE_OUTER_BOUND ( 'NONE', #76552, .T. ) ;
#12992=CYLINDRICAL_SURFACE ( 'NONE', #13910, 0.2500000000000002220 ) ;
#12997=CIRCLE ( 'NONE', #48117, 0.2500000000000002220 ) ;
#12999=EDGE_CURVE ( 'NONE', #32841, #15068, #1348, .T. ) ;
#13014=CARTESIAN_POINT ( 'NONE',  ( -3.750000000000000000, 36.75000000000000000, -2.500000000000000000 ) ) ;
#13017=( LENGTH_UNIT ( ) NAMED_UNIT ( * ) SI_UNIT ( .MILLI., .METRE. ) );
#13027=DIRECTION ( 'NONE',  ( 0.000000000000000000, -1.000000000000000000, -2.602085213965208275E-15 ) ) ;
#13028=CARTESIAN_POINT ( 'NONE',  ( -8.000000000000000000, 79.82179676972448590, -6.250000000000000000 ) ) ;
#13041=DIRECTION ( 'NONE',  ( -1.000000000000000000, 0.000000000000000000, 0.000000000000000000 ) ) ;
#13046=PRESENTATION_STYLE_ASSIGNMENT (( #35044 ) ) ;
#13052=SURFACE_SIDE_STYLE ('',( #51554 ) ) ;
#13062=VERTEX_POINT ( 'NONE', #59914 ) ;
#13075=VERTEX_POINT ( 'NONE', #68421 ) ;
#13086=EDGE_CURVE ( 'NONE', #42611, #56730, #20457, .T. ) ;
#13087=( LENGTH_UNIT ( ) NAMED_UNIT ( * ) SI_UNIT ( .MILLI., .METRE. ) );
#13089=ORIENTED_EDGE ( 'NONE', *, *, #48770, .F. ) ;
#13092=VERTEX_POINT ( 'NONE', #30398 ) ;
#13111=CARTESIAN_POINT ( 'NONE',  ( 8.880000000000020322, 80.07179676972448590, 6.250000000000000000 ) ) ;
#13122=CARTESIAN_POINT ( 'NONE',  ( -3.500000000000000444, 1.019547802438453887, -3.750000000000000000 ) ) ;
#13123=EDGE_CURVE ( 'NONE', #37045, #83910, #16190, .T. ) ;
#13124=CYLINDRICAL_SURFACE ( 'NONE', #46921, 0.1000000000000000333 ) ;
#13130=CARTESIAN_POINT ( 'NONE',  ( -10.77730536144846596, -98.63085534186639336, -3.749999999999994671 ) ) ;
#13132=DIRECTION ( 'NONE',  ( -0.000000000000000000, 1.000000000000000000, -0.000000000000000000 ) ) ;
#13140=UNCERTAINTY_MEASURE_WITH_UNIT (LENGTH_MEASURE( 1.000000000000000082E-05 ), #47808, 'distance_accuracy_value', 'NONE');
#13169=CARTESIAN_POINT ( 'NONE',  ( -10.77984007350130469, -96.52126437880588128, 4.000000000000000000 ) ) ;
#13174=COLOUR_RGB ( '', 0.08235294, 0.09019608, 0.10196078) ;
#13178=SURFACE_STYLE_FILL_AREA ( #37184 ) ;
#13180=VECTOR ( 'NONE', #36872, 1000.000000000000000 ) ;
#13195=ORIENTED_EDGE ( 'NONE', *, *, #21354, .T. ) ;
#13207=CARTESIAN_POINT ( 'NONE',  ( -8.000000000000000000, 83.99999999999994316, 3.750000000000000000 ) ) ;
#13208=VECTOR ( 'NONE', #21836, 1000.000000000000000 ) ;
#13212=EDGE_CURVE ( 'NONE', #4322, #17079, #39190, .T. ) ;
#13229=AXIS2_PLACEMENT_3D ( 'NONE', #87305, #12292, #72779 ) ;
#13232=ADVANCED_FACE ( 'NONE', ( #47663, #1209 ), #7211, .T. ) ;
#13235=EDGE_LOOP ( 'NONE', ( #75658, #56590, #97259, #94384 ) ) ;
#13236=AXIS2_PLACEMENT_3D ( 'NONE', #34378, #11396, #63410 ) ;
#13242=EDGE_CURVE ( 'NONE', #96688, #52732, #14098, .T. ) ;
#13253=FACE_OUTER_BOUND ( 'NONE', #11347, .T. ) ;
#13276=FILL_AREA_STYLE ('',( #97295 ) ) ;
#13281=CIRCLE ( 'NONE', #42062, 0.2500000000000002220 ) ;
#13284=VECTOR ( 'NONE', #11870, 1000.000000000000000 ) ;
#13287=LINE ( 'NONE', #43775, #31651 ) ;
#13317=EDGE_LOOP ( 'NONE', ( #80166, #53526, #64662, #79863 ) ) ;
#13324=EDGE_CURVE ( 'NONE', #30576, #38057, #82757, .T. ) ;
#13334=DIRECTION ( 'NONE',  ( 0.000000000000000000, -1.000000000000000000, -0.000000000000000000 ) ) ;
#13342=CARTESIAN_POINT ( 'NONE',  ( -13.80050776813097002, 90.89648773604355370, -7.753931633032691728 ) ) ;
#13354=FILL_AREA_STYLE ('',( #81840 ) ) ;
#13357=ORIENTED_EDGE ( 'NONE', *, *, #57021, .T. ) ;
#13381=CARTESIAN_POINT ( 'NONE',  ( -7.072497013529895682, -84.40007040885102185, -2.750000000000805578 ) ) ;
#13382=DIRECTION ( 'NONE',  ( 0.000000000000000000, 0.000000000000000000, 1.000000000000000000 ) ) ;
#13388=AXIS2_PLACEMENT_3D ( 'NONE', #64139, #41676, #70692 ) ;
#13389=CARTESIAN_POINT ( 'NONE',  ( 17.75000000000000711, 43.00000000000000000, 6.250000000000000000 ) ) ;
#13390=CARTESIAN_POINT ( 'NONE',  ( -11.23890517442507075, -88.22482801187260293, -4.000000000000000888 ) ) ;
#13395=CARTESIAN_POINT ( 'NONE',  ( -4.000000000000000000, 10.25000000000000000, -2.750000000000000000 ) ) ;
#13409=ORIENTED_EDGE ( 'NONE', *, *, #24949, .T. ) ;
#13420=EDGE_CURVE ( 'NONE', #33129, #22102, #49133, .T. ) ;
#13428=FILL_AREA_STYLE ('',( #51929 ) ) ;
#13449=VECTOR ( 'NONE', #91442, 999.9999999999998863 ) ;
#13450=DIRECTION ( 'NONE',  ( 0.000000000000000000, 0.000000000000000000, -1.000000000000000000 ) ) ;
#13470=CARTESIAN_POINT ( 'NONE',  ( 10.58840669699852199, -98.14374106289703548, -3.750000000000000000 ) ) ;
#13471=CARTESIAN_POINT ( 'NONE',  ( 11.10646695662408767, -65.08356741887227770, 4.000000000000000000 ) ) ;
#13473=ORIENTED_EDGE ( 'NONE', *, *, #734, .T. ) ;
#13478=EDGE_CURVE ( 'NONE', #11027, #66682, #86650, .T. ) ;
#13480=B_SPLINE_CURVE_WITH_KNOTS ( 'NONE', 3,
 ( #53551, #37585, #52085, #22585, #83573, #45566, #601, #45063, #29071, #104, #75572, #82578, #68572, #84066, #97612, #74577, #67590, #76061, #30550, #15092, #60567, #38083, #44576, #7085 ),
 .UNSPECIFIED., .F., .F.,
 ( 4, 2, 2, 2, 2, 2, 2, 2, 2, 2, 2, 4 ),
 ( 0.000000000000000000, 0.003099737161558395546, 0.006199474323116791093, 0.01239894864623362208, 0.02479789729246732743, 0.03719684593870102585, 0.04959579458493475201, 0.07439369187740220435, 0.08679264052363593052, 0.09299211484675279360, 0.09609185200831121820, 0.09919158916986964281 ),
 .UNSPECIFIED. ) ;
#13544=EDGE_CURVE ( 'NONE', #57586, #93536, #72604, .T. ) ;
#13545=CARTESIAN_POINT ( 'NONE',  ( 9.512243806915856581, -15.51051116580330635, -3.750000000000000888 ) ) ;
#13546=CARTESIAN_POINT ( 'NONE',  ( -3.500000000000000444, 1.019547802438453887, -3.750000000000000000 ) ) ;
#13552=DIRECTION ( 'NONE',  ( 1.000000000000000000, 0.000000000000000000, 0.000000000000000000 ) ) ;
#13562=ORIENTED_EDGE ( 'NONE', *, *, #15724, .T. ) ;
#13563=ORIENTED_EDGE ( 'NONE', *, *, #77125, .F. ) ;
#13571=DIRECTION ( 'NONE',  ( -1.000000000000000000, 0.000000000000000000, 0.000000000000000000 ) ) ;
#13576=EDGE_CURVE ( 'NONE', #68711, #11943, #81100, .T. ) ;
#13580=ORIENTED_EDGE ( 'NONE', *, *, #942, .T. ) ;
#13593=MECHANICAL_DESIGN_GEOMETRIC_PRESENTATION_REPRESENTATION('',(#63121),#48710);
#13594=DIRECTION ( 'NONE',  ( 0.000000000000000000, 0.000000000000000000, -1.000000000000000000 ) ) ;
#13598=FILL_AREA_STYLE ('',( #66091 ) ) ;
#13599=CARTESIAN_POINT ( 'NONE',  ( -7.116236362341394006, -80.68324313941631942, 3.750000000000001332 ) ) ;
#13600=DIRECTION ( 'NONE',  ( 1.000000000000000000, 0.000000000000000000, 0.000000000000000000 ) ) ;
#13619=CARTESIAN_POINT ( 'NONE',  ( 0.000000000000000000, 91.00000000000000000, 8.000000000000000000 ) ) ;
#13621=CARTESIAN_POINT ( 'NONE',  ( 15.00000000000000000, 77.07179676972447169, 4.250000000000000000 ) ) ;
#13630=CIRCLE ( 'NONE', #58293, 10.09999999999999787 ) ;
#13650=DIRECTION ( 'NONE',  ( -0.000000000000000000, 0.000000000000000000, 1.000000000000000000 ) ) ;
#13654=CIRCLE ( 'NONE', #47188, 0.2500000000000002220 ) ;
#13659=ORIENTED_EDGE ( 'NONE', *, *, #86431, .F. ) ;
#13660=VECTOR ( 'NONE', #36857, 1000.000000000000000 ) ;
#13667=CARTESIAN_POINT ( 'NONE',  ( -11.17376097873395047, -90.29818107661104420, 4.000000000000000000 ) ) ;
#13672=MECHANICAL_DESIGN_GEOMETRIC_PRESENTATION_REPRESENTATION('',(#16894),#95089);
#13688=VECTOR ( 'NONE', #38718, 1000.000000000000000 ) ;
#13692=ORIENTED_EDGE ( 'NONE', *, *, #83031, .T. ) ;
#13704=AXIS2_PLACEMENT_3D ( 'NONE', #38714, #69213, #739 ) ;
#13712=CARTESIAN_POINT ( 'NONE',  ( -9.000000000000001776, 80.99999999999994316, 2.900000000000001243 ) ) ;
#13716=ORIENTED_EDGE ( 'NONE', *, *, #38119, .T. ) ;
#13723=PRESENTATION_STYLE_ASSIGNMENT (( #97745 ) ) ;
#13728=ADVANCED_FACE ( 'NONE', ( #59086 ), #12603, .F. ) ;
#13735=AXIS2_PLACEMENT_3D ( 'NONE', #91284, #22317, #22806 ) ;
#13760=CARTESIAN_POINT ( 'NONE',  ( -11.82883858055346415, 90.33605471726345115, -7.015824399821311452 ) ) ;
#13768=CARTESIAN_POINT ( 'NONE',  ( 11.35644985441411059, -65.08036738588863557, -4.000000000000000000 ) ) ;
#13782=VERTEX_POINT ( 'NONE', #21104 ) ;
#13784=CYLINDRICAL_SURFACE ( 'NONE', #76339, 0.2500000000000002220 ) ;
#13790=ADVANCED_FACE ( 'NONE', ( #51603 ), #44583, .T. ) ;
#13792=LINE ( 'NONE', #14298, #11944 ) ;
#13796=CARTESIAN_POINT ( 'NONE',  ( 8.880000000000000782, 1.116573172248542834E-15, 3.750000000000000000 ) ) ;
#13799=CARTESIAN_POINT ( 'NONE',  ( -3.500000000000000444, 0.08393865084445589764, 3.750000000000000000 ) ) ;
#13809=LINE ( 'NONE', #19819, #96837 ) ;
#13810=( GEOMETRIC_REPRESENTATION_CONTEXT ( 3 ) GLOBAL_UNCERTAINTY_ASSIGNED_CONTEXT ( ( #60114 ) ) GLOBAL_UNIT_ASSIGNED_CONTEXT ( ( #66745, #88752, #35750 ) ) REPRESENTATION_CONTEXT ( 'NONE', 'WORKASPACE' ) );
#13812=AXIS2_PLACEMENT_3D ( 'NONE', #30275, #8767, #31754 ) ;
#13831=ORIENTED_EDGE ( 'NONE', *, *, #45198, .F. ) ;
#13832=STYLED_ITEM ( 'NONE', ( #92071 ), #38078 ) ;
#13842=CARTESIAN_POINT ( 'NONE',  ( -13.79358826900837265, 90.89928960263274860, -7.799418555803335984 ) ) ;
#13846=TOROIDAL_SURFACE ( 'NONE', #69742, 2.250000000000001332, 0.2500000000000000000 ) ;
#13847=( NAMED_UNIT ( * ) SI_UNIT ( $, .STERADIAN. ) SOLID_ANGLE_UNIT ( ) );
#13852=ORIENTED_EDGE ( 'NONE', *, *, #48083, .T. ) ;
#13861=ORIENTED_EDGE ( 'NONE', *, *, #90819, .T. ) ;
#13873=DIRECTION ( 'NONE',  ( -0.000000000000000000, 0.000000000000000000, 1.000000000000000000 ) ) ;
#13879=FACE_OUTER_BOUND ( 'NONE', #94221, .T. ) ;
#13882=CIRCLE ( 'NONE', #31417, 3.000000000000000888 ) ;
#13884=CARTESIAN_POINT ( 'NONE',  ( -7.232415441807423129, -88.12698951299773853, -3.750000000000000000 ) ) ;
#13893=DIRECTION ( 'NONE',  ( 0.000000000000000000, 0.000000000000000000, 1.000000000000000000 ) ) ;
#13898=SURFACE_STYLE_USAGE ( .BOTH. , #51894 ) ;
#13905=EDGE_CURVE ( 'NONE', #41505, #21427, #73244, .T. ) ;
#13910=AXIS2_PLACEMENT_3D ( 'NONE', #51491, #74979, #27994 ) ;
#13947=VERTEX_POINT ( 'NONE', #50433 ) ;
#13973=CARTESIAN_POINT ( 'NONE',  ( -7.121341127240343738, -73.24353698637879972, 2.500000000000000000 ) ) ;
#13978=CARTESIAN_POINT ( 'NONE',  ( 11.29389914936710859, -89.89072489378423825, 3.750000000000000000 ) ) ;
#13981=CIRCLE ( 'NONE', #28313, 3.690000000000000391 ) ;
#13983=CARTESIAN_POINT ( 'NONE',  ( 4.645843784090632589, -0.8374430341443435122, 3.999999999999999112 ) ) ;
#13992=CARTESIAN_POINT ( 'NONE',  ( -13.73837289480035651, 90.95369347093435408, -7.920836650016501501 ) ) ;
#14001=EDGE_CURVE ( 'NONE', #72372, #80582, #4444, .T. ) ;
#14015=AXIS2_PLACEMENT_3D ( 'NONE', #89720, #46206, #30198 ) ;
#14022=SURFACE_SIDE_STYLE ('',( #37013 ) ) ;
#14029=EDGE_CURVE ( 'NONE', #92036, #16571, #65899, .T. ) ;
#14032=EDGE_CURVE ( 'NONE', #76760, #1168, #87599, .T. ) ;
#14048=CARTESIAN_POINT ( 'NONE',  ( 11.35674113183028311, -65.10122143319173915, -3.750000000000000000 ) ) ;
#14049=CARTESIAN_POINT ( 'NONE',  ( -7.072388532688812290, -84.40601219567531643, -4.000000000001612932 ) ) ;
#14050=COLOUR_RGB ( '', 0.40784314, 0.44705882, 0.49803922) ;
#14052=VERTEX_POINT ( 'NONE', #95932 ) ;
#14065=ADVANCED_FACE ( 'NONE', ( #5430 ), #72414, .F. ) ;
#14081=ORIENTED_EDGE ( 'NONE', *, *, #33950, .T. ) ;
#14092=AXIS2_PLACEMENT_3D ( 'NONE', #73429, #90900, #21433 ) ;
#14094=VERTEX_POINT ( 'NONE', #88910 ) ;
#14098=CIRCLE ( 'NONE', #92316, 2.900000000000002576 ) ;
#14100=DIRECTION ( 'NONE',  ( 1.000000000000000000, 0.000000000000000000, 0.000000000000000000 ) ) ;
#14102=CARTESIAN_POINT ( 'NONE',  ( -3.750000000000000000, 36.75000000000000000, -2.750000000000000000 ) ) ;
#14113=PLANE ( 'NONE',  #87260 ) ;
#14115=AXIS2_PLACEMENT_3D ( 'NONE', #66558, #97086, #59052 ) ;
#14116=CARTESIAN_POINT ( 'NONE',  ( 6.879999999999995453, 43.00000000000000000, 6.500000000000000888 ) ) ;
#14119=ORIENTED_EDGE ( 'NONE', *, *, #96580, .F. ) ;
#14138=( NAMED_UNIT ( * ) PLANE_ANGLE_UNIT ( ) SI_UNIT ( $, .RADIAN. ) );
#14142=EDGE_CURVE ( 'NONE', #26894, #85540, #42933, .T. ) ;
#14161=CARTESIAN_POINT ( 'NONE',  ( 6.324651560463742328, -50.88858560574520595, 2.500000000000000000 ) ) ;
#14171=CARTESIAN_POINT ( 'NONE',  ( -10.67064208003667325, -97.55764508345595232, 4.000000000000000000 ) ) ;
#14179=AXIS2_PLACEMENT_3D ( 'NONE', #88417, #27412, #65407 ) ;
#14183=ORIENTED_EDGE ( 'NONE', *, *, #72465, .F. ) ;
#14185=ORIENTED_EDGE ( 'NONE', *, *, #93607, .T. ) ;
#14192=ADVANCED_FACE ( 'NONE', ( #61764 ), #22242, .T. ) ;
#14194=CARTESIAN_POINT ( 'NONE',  ( 9.879999999999990123, 18.09999999999999787, 0.000000000000000000 ) ) ;
#14210=CIRCLE ( 'NONE', #70090, 0.2500000000000002220 ) ;
#14213=ORIENTED_EDGE ( 'NONE', *, *, #61171, .F. ) ;
#14217=DIRECTION ( 'NONE',  ( 0.000000000000000000, -1.000000000000000000, 0.000000000000000000 ) ) ;
#14220=CARTESIAN_POINT ( 'NONE',  ( -4.000000000000000000, 36.75000000000000000, 3.750000000000000000 ) ) ;
#14222=CARTESIAN_POINT ( 'NONE',  ( 15.00000000000000178, 73.00000000000000000, 6.250000000000000000 ) ) ;
#14237=ORIENTED_EDGE ( 'NONE', *, *, #47439, .F. ) ;
#14243=( NAMED_UNIT ( * ) SI_UNIT ( $, .STERADIAN. ) SOLID_ANGLE_UNIT ( ) );
#14244=STYLED_ITEM ( 'NONE', ( #45279 ), #14513 ) ;
#14246=CARTESIAN_POINT ( 'NONE',  ( 4.879999999999991900, 76.07179676972444327, 6.500000000000000888 ) ) ;
#14253=CARTESIAN_POINT ( 'NONE',  ( -4.000000000000000000, 37.00000000000000000, -2.750000000000000000 ) ) ;
#14254=STYLED_ITEM ( 'NONE', ( #42585 ), #60195 ) ;
#14268=UNCERTAINTY_MEASURE_WITH_UNIT (LENGTH_MEASURE( 1.000000000000000082E-05 ), #6832, 'distance_accuracy_value', 'NONE');
#14272=EDGE_CURVE ( 'NONE', #32382, #17988, #66910, .T. ) ;
#14273=ORIENTED_EDGE ( 'NONE', *, *, #75562, .T. ) ;
#14275=CARTESIAN_POINT ( 'NONE',  ( 11.20666035741388278, -56.81027457019842331, -3.750000000000000000 ) ) ;
#14290=EDGE_LOOP ( 'NONE', ( #16276, #19106, #82937, #51062 ) ) ;
#14292=DIRECTION ( 'NONE',  ( 0.000000000000000000, 0.000000000000000000, 1.000000000000000000 ) ) ;
#14298=CARTESIAN_POINT ( 'NONE',  ( -1.899999999999997247, 98.49999999999998579, -8.525133428036873795 ) ) ;
#14305=CIRCLE ( 'NONE', #49389, 0.2500000000000000000 ) ;
#14306=FILL_AREA_STYLE ('',( #83776 ) ) ;
#14309=ORIENTED_EDGE ( 'NONE', *, *, #52388, .T. ) ;
#14317=VERTEX_POINT ( 'NONE', #93319 ) ;
#14338=CARTESIAN_POINT ( 'NONE',  ( 4.656465524211139240, -8.255743748965677753, -3.750000000000000444 ) ) ;
#14340=FILL_AREA_STYLE_COLOUR ( '', #96352 ) ;
#14341=CARTESIAN_POINT ( 'NONE',  ( -8.099999999999999645, 80.99999999999994316, 2.900000000000001243 ) ) ;
#14345=( NAMED_UNIT ( * ) PLANE_ANGLE_UNIT ( ) SI_UNIT ( $, .RADIAN. ) );
#14355=( NAMED_UNIT ( * ) PLANE_ANGLE_UNIT ( ) SI_UNIT ( $, .RADIAN. ) );
#14359=EDGE_LOOP ( 'NONE', ( #185, #82800, #58560, #60681 ) ) ;
#14376=DIRECTION ( 'NONE',  ( -0.000000000000000000, -0.000000000000000000, 1.000000000000000000 ) ) ;
#14380=ADVANCED_FACE ( 'NONE', ( #42820 ), #38167, .T. ) ;
#14389=EDGE_CURVE ( 'NONE', #49831, #32093, #73793, .T. ) ;
#14392=CARTESIAN_POINT ( 'NONE',  ( -7.778994393464220281, -1.060811710757841198, -4.000000000000000000 ) ) ;
#14427=CARTESIAN_POINT ( 'NONE',  ( 12.99999999999999822, 75.00000000000000000, -6.500000000000000888 ) ) ;
#14432=CARTESIAN_POINT ( 'NONE',  ( 6.935087012957517949, -80.58470470491535309, 3.750000000000000000 ) ) ;
#14433=CARTESIAN_POINT ( 'NONE',  ( -7.750355510519348456, 84.07179676972448590, 4.000000000000000000 ) ) ;
#14437=CARTESIAN_POINT ( 'NONE',  ( -10.77730536144846596, -98.63085534186639336, -3.750000000000000000 ) ) ;
#14464=CARTESIAN_POINT ( 'NONE',  ( -7.037799269745396380, -86.25965645050762021, 2.499999999998388400 ) ) ;
#14468=DIRECTION ( 'NONE',  ( 0.000000000000000000, 0.000000000000000000, 1.000000000000000000 ) ) ;
#14470=ORIENTED_EDGE ( 'NONE', *, *, #5361, .F. ) ;
#14476=ADVANCED_FACE ( 'NONE', ( #96329 ), #27804, .F. ) ;
#14479=ADVANCED_FACE ( 'NONE', ( #95825 ), #53768, .F. ) ;
#14494=EDGE_CURVE ( 'NONE', #59039, #26330, #52563, .T. ) ;
#14497=LINE ( 'NONE', #92436, #76131 ) ;
#14498=( NAMED_UNIT ( * ) PLANE_ANGLE_UNIT ( ) SI_UNIT ( $, .RADIAN. ) );
#14513=ADVANCED_FACE ( 'NONE', ( #37306 ), #28544, .T. ) ;
#14521=CARTESIAN_POINT ( 'NONE',  ( -7.750000000000000000, 1.019547802438458550, -4.000000000000000000 ) ) ;
#14532=DIRECTION ( 'NONE',  ( -1.049065152435176504E-16, 1.000000000000000000, -0.000000000000000000 ) ) ;
#14544=DIRECTION ( 'NONE',  ( 1.000000000000000000, 2.569960705150826877E-16, -0.000000000000000000 ) ) ;
#14547=CARTESIAN_POINT ( 'NONE',  ( 8.900374253113422895, -1.048990366506262317, -3.750000000000001332 ) ) ;
#14548=CARTESIAN_POINT ( 'NONE',  ( -7.371446924914479837, -73.25787537890647627, -4.000000000000000888 ) ) ;
#14550=( GEOMETRIC_REPRESENTATION_CONTEXT ( 3 ) GLOBAL_UNCERTAINTY_ASSIGNED_CONTEXT ( ( #93339 ) ) GLOBAL_UNIT_ASSIGNED_CONTEXT ( ( #54088, #14138, #71079 ) ) REPRESENTATION_CONTEXT ( 'NONE', 'WORKASPACE' ) );
#14563=AXIS2_PLACEMENT_3D ( 'NONE', #23877, #16361, #24366 ) ;
#14569=CARTESIAN_POINT ( 'NONE',  ( -10.98829462902744858, 46.98606209026556968, 0.000000000000000000 ) ) ;
#14578=ADVANCED_FACE ( 'NONE', ( #48226 ), #77739, .T. ) ;
#14585=VERTEX_POINT ( 'NONE', #10730 ) ;
#14601=ORIENTED_EDGE ( 'NONE', *, *, #54627, .T. ) ;
#14605=EDGE_CURVE ( 'NONE', #2203, #54884, #38776, .T. ) ;
#14631=CARTESIAN_POINT ( 'NONE',  ( -4.247994584727555534, -13.56436116443237516, -3.750000000000000000 ) ) ;
#14661=DIRECTION ( 'NONE',  ( 1.000000000000000000, 0.000000000000000000, 0.000000000000000000 ) ) ;
#14668=EDGE_LOOP ( 'NONE', ( #68747, #73289, #52542, #40626 ) ) ;
#14669=AXIS2_PLACEMENT_3D ( 'NONE', #20292, #81281, #73773 ) ;
#14675=CARTESIAN_POINT ( 'NONE',  ( -11.37541478881037271, -75.76447409171241532, 4.000000000000000000 ) ) ;
#14703=ORIENTED_EDGE ( 'NONE', *, *, #55004, .F. ) ;
#14707=CIRCLE ( 'NONE', #89694, 0.2500000000000002220 ) ;
#14712=CARTESIAN_POINT ( 'NONE',  ( 3.969999999999999751, 10.25000000000000000, 2.750000000000000000 ) ) ;
#14737=CARTESIAN_POINT ( 'NONE',  ( 3.969999999999999751, 36.75000000000000000, -3.750000000000000000 ) ) ;
#14743=DIRECTION ( 'NONE',  ( -1.000000000000000000, -1.927470528863119542E-16, 0.000000000000000000 ) ) ;
#14751=DIRECTION ( 'NONE',  ( -0.000000000000000000, -0.000000000000000000, 1.000000000000000000 ) ) ;
#14761=AXIS2_PLACEMENT_3D ( 'NONE', #82199, #12718, #66204 ) ;
#14773=ORIENTED_EDGE ( 'NONE', *, *, #20104, .F. ) ;
#14776=CARTESIAN_POINT ( 'NONE',  ( 10.83696084481538868, -98.17058944465519232, -4.000000000000000000 ) ) ;
#14787=COLOUR_RGB ( '', 0.66274510, 0.83137255, 0.94901961) ;
#14804=CARTESIAN_POINT ( 'NONE',  ( 4.406177045957827332, -8.255047197809593840, -2.500000000000000000 ) ) ;
#14808=SURFACE_STYLE_USAGE ( .BOTH. , #23290 ) ;
#14811=ORIENTED_EDGE ( 'NONE', *, *, #68798, .F. ) ;
#14813=VERTEX_POINT ( 'NONE', #98785 ) ;
#14826=DIRECTION ( 'NONE',  ( 0.000000000000000000, 0.000000000000000000, -1.000000000000000000 ) ) ;
#14830=CIRCLE ( 'NONE', #62686, 10.65000000000000036 ) ;
#14846=VECTOR ( 'NONE', #85824, 1000.000000000000000 ) ;
#14856=ORIENTED_EDGE ( 'NONE', *, *, #42334, .T. ) ;
#14873=VERTEX_POINT ( 'NONE', #52745 ) ;
#14874=AXIS2_PLACEMENT_3D ( 'NONE', #85696, #10196, #93679 ) ;
#14877=FILL_AREA_STYLE_COLOUR ( '', #33928 ) ;
#14879=AXIS2_PLACEMENT_3D ( 'NONE', #84671, #84191, #98726 ) ;
#14884=CARTESIAN_POINT ( 'NONE',  ( 6.284583270191197002, -88.40194713205143273, -3.750000000000000000 ) ) ;
#14891=EDGE_LOOP ( 'NONE', ( #11219, #34464, #6947, #45931 ) ) ;
#14892=( NAMED_UNIT ( * ) SI_UNIT ( $, .STERADIAN. ) SOLID_ANGLE_UNIT ( ) );
#14898=DIRECTION ( 'NONE',  ( 0.000000000000000000, 1.000000000000000000, 0.000000000000000000 ) ) ;
#14910=CIRCLE ( 'NONE', #56434, 3.000000000000000888 ) ;
#14914=CARTESIAN_POINT ( 'NONE',  ( -6.000000000000000000, 78.07179676972447169, 6.250000000000000000 ) ) ;
#14927=DIRECTION ( 'NONE',  ( 1.000000000000000000, 0.000000000000000000, 0.000000000000000000 ) ) ;
#14931=CARTESIAN_POINT ( 'NONE',  ( 6.757940885639631468, -58.32678904743398363, 3.750000000000000000 ) ) ;
#14945=CARTESIAN_POINT ( 'NONE',  ( 17.75000000000000355, 84.07179676972448590, 4.000000000000000000 ) ) ;
#14950=STYLED_ITEM ( 'NONE', ( #21762 ), #40082 ) ;
#14952=EDGE_CURVE ( 'NONE', #67464, #40303, #76250, .T. ) ;
#14966=DIRECTION ( 'NONE',  ( 0.000000000000000000, -0.000000000000000000, 1.000000000000000000 ) ) ;
#14970=DIRECTION ( 'NONE',  ( 1.000000000000000000, -0.000000000000000000, -0.000000000000000000 ) ) ;
#14972=VERTEX_POINT ( 'NONE', #53244 ) ;
#14975=CIRCLE ( 'NONE', #75619, 0.2500000000000002220 ) ;
#14978=CARTESIAN_POINT ( 'NONE',  ( -11.22722615950653413, 89.90850287678183861, 6.380836486320208500 ) ) ;
#14986=CARTESIAN_POINT ( 'NONE',  ( 4.526800700887880780, -5.190657137169758073, -2.750000000000000000 ) ) ;
#15001=ORIENTED_EDGE ( 'NONE', *, *, #87170, .T. ) ;
#15018=PRESENTATION_STYLE_ASSIGNMENT (( #29484 ) ) ;
#15029=( LENGTH_UNIT ( ) NAMED_UNIT ( * ) SI_UNIT ( .MILLI., .METRE. ) );
#15038=DIRECTION ( 'NONE',  ( 1.000000000000000000, -0.000000000000000000, -0.000000000000000000 ) ) ;
#15041=DIRECTION ( 'NONE',  ( 0.000000000000000000, 0.000000000000000000, -1.000000000000000000 ) ) ;
#15046=CARTESIAN_POINT ( 'NONE',  ( -7.124934413272103306, -78.83349193436582425, -4.000000000000001776 ) ) ;
#15053=COLOUR_RGB ( '', 0.72549020, 0.75294118, 0.79215686) ;
#15063=AXIS2_PLACEMENT_3D ( 'NONE', #63652, #55684, #86184 ) ;
#15068=VERTEX_POINT ( 'NONE', #24241 ) ;
#15078=EDGE_CURVE ( 'NONE', #14052, #73541, #65087, .T. ) ;
#15092=CARTESIAN_POINT ( 'NONE',  ( 8.742110228208591849, -4.148858702914717256, 4.000000000000000000 ) ) ;
#15093=VERTEX_POINT ( 'NONE', #78204 ) ;
#15095=EDGE_LOOP ( 'NONE', ( #90786, #69838, #57977, #30280 ) ) ;
#15098=PLANE ( 'NONE',  #88958 ) ;
#15099=DIRECTION ( 'NONE',  ( 1.000000000000000000, 0.000000000000000000, 0.000000000000000000 ) ) ;
#15101=DIRECTION ( 'NONE',  ( 1.000000000000000000, 2.107602052970794797E-16, -0.000000000000000000 ) ) ;
#15110=DIRECTION ( 'NONE',  ( -1.000000000000000000, -0.000000000000000000, -0.000000000000000000 ) ) ;
#15114=( GEOMETRIC_REPRESENTATION_CONTEXT ( 3 ) GLOBAL_UNCERTAINTY_ASSIGNED_CONTEXT ( ( #6467 ) ) GLOBAL_UNIT_ASSIGNED_CONTEXT ( ( #63702, #93717, #3721 ) ) REPRESENTATION_CONTEXT ( 'NONE', 'WORKASPACE' ) );
#15120=LINE ( 'NONE', #45596, #87932 ) ;
#15122=AXIS2_PLACEMENT_3D ( 'NONE', #49523, #43505, #72520 ) ;
#15123=PLANE ( 'NONE',  #98130 ) ;
#15132=DIRECTION ( 'NONE',  ( -1.049065152435176504E-16, 1.000000000000000000, -0.000000000000000000 ) ) ;
#15133=FILL_AREA_STYLE ('',( #23626 ) ) ;
#15139=UNCERTAINTY_MEASURE_WITH_UNIT (LENGTH_MEASURE( 1.000000000000000082E-05 ), #11881, 'distance_accuracy_value', 'NONE');
#15142=DIRECTION ( 'NONE',  ( -1.000000000000000000, 0.000000000000000000, 0.000000000000000000 ) ) ;
#15147=PRESENTATION_STYLE_ASSIGNMENT (( #44634 ) ) ;
#15156=ADVANCED_FACE ( 'NONE', ( #55713 ), #38687, .F. ) ;
#15164=CARTESIAN_POINT ( 'NONE',  ( -10.32520421616337813, -40.46224970679962496, 4.000000000000000000 ) ) ;
#15169=EDGE_CURVE ( 'NONE', #6847, #85540, #17242, .T. ) ;
#15171=FACE_OUTER_BOUND ( 'NONE', #47847, .T. ) ;
#15176=CARTESIAN_POINT ( 'NONE',  ( -8.000000000000000000, 41.24999999999999289, 6.500000000000000888 ) ) ;
#15178=VERTEX_POINT ( 'NONE', #80669 ) ;
#15179=DIRECTION ( 'NONE',  ( 0.000000000000000000, 0.000000000000000000, -1.000000000000000000 ) ) ;
#15198=DIRECTION ( 'NONE',  ( 0.000000000000000000, -0.000000000000000000, 1.000000000000000000 ) ) ;
#15206=DIRECTION ( 'NONE',  ( 0.000000000000000000, -0.000000000000000000, -1.000000000000000000 ) ) ;
#15210=FILL_AREA_STYLE_COLOUR ( '', #97275 ) ;
#15212=CARTESIAN_POINT ( 'NONE',  ( -18.00000000000000355, 75.73428692542562146, 3.000000000000000000 ) ) ;
#15230=FACE_OUTER_BOUND ( 'NONE', #15484, .T. ) ;
#15242=B_SPLINE_CURVE_WITH_KNOTS ( 'NONE', 3,
 ( #79081, #29025, #97073, #43059, #82034, #52524, #59532, #66545, #28546, #21054, #6052, #67541, #59038, #14048, #50555, #51545, #98055, #27549, #36550, #13545, #20558, #67040, #44530, #35551, #14547, #45018, #37043 ),
 .UNSPECIFIED., .F., .F.,
 ( 4, 2, 2, 2, 1, 2, 2, 2, 2, 2, 2, 2, 2, 4 ),
 ( -6.000000001272176776E-08, 0.0007750911056877003409, 0.001550242211375413553, 0.003100544422750839760, 0.006201148845501692174, 0.01240235769100339613, 0.02480477538200680579, 0.03720719307301021544, 0.04960961076401360775, 0.07441444614602037155, 0.08681686383702374998, 0.09301807268252543226, 0.09611867710527627340, 0.09921928152802711454 ),
 .UNSPECIFIED. ) ;
#15244=CARTESIAN_POINT ( 'NONE',  ( -7.750000000000000000, 79.82179676972448590, -4.250000000000000000 ) ) ;
#15264=CARTESIAN_POINT ( 'NONE',  ( -8.924603092375777535, 75.06466731010172566, 3.000000000000000000 ) ) ;
#15271=CARTESIAN_POINT ( 'NONE',  ( 10.47193227291256790, -40.28585825689869893, -4.000000000000000000 ) ) ;
#15276=SURFACE_SIDE_STYLE ('',( #98790 ) ) ;
#15280=FILL_AREA_STYLE_COLOUR ( '', #11240 ) ;
#15292=CARTESIAN_POINT ( 'NONE',  ( -18.89999999999999147, 99.99999999999998579, -7.750000000000000000 ) ) ;
#15294=EDGE_CURVE ( 'NONE', #32092, #96723, #89089, .T. ) ;
#15299=CARTESIAN_POINT ( 'NONE',  ( -3.750000000000000888, 1.019547802438453887, 4.000000000000000000 ) ) ;
#15309=ORIENTED_EDGE ( 'NONE', *, *, #73045, .T. ) ;
#15311=CIRCLE ( 'NONE', #56613, 0.2500000000000002220 ) ;
#15312=EDGE_CURVE ( 'NONE', #63974, #58305, #61892, .T. ) ;
#15313=ORIENTED_EDGE ( 'NONE', *, *, #88300, .F. ) ;
#15320=CARTESIAN_POINT ( 'NONE',  ( -4.250000000000000000, 0.000000000000000000, -3.750000000000000000 ) ) ;
#15322=DIRECTION ( 'NONE',  ( 1.000000000000000000, -0.000000000000000000, -0.000000000000000000 ) ) ;
#15326=VECTOR ( 'NONE', #93095, 999.9999999999998863 ) ;
#15327=VECTOR ( 'NONE', #43308, 999.9999999999998863 ) ;
#15329=ORIENTED_EDGE ( 'NONE', *, *, #15680, .T. ) ;
#15332=FACE_OUTER_BOUND ( 'NONE', #79308, .T. ) ;
#15333=CIRCLE ( 'NONE', #4181, 0.2500000000000002220 ) ;
#15354=CARTESIAN_POINT ( 'NONE',  ( 5.783743716939243384, -36.05632648146325181, -2.499999999999999112 ) ) ;
#15358=CARTESIAN_POINT ( 'NONE',  ( 0.000000000000000000, 80.32179676972448590, -4.250000000000000000 ) ) ;
#15370=DIRECTION ( 'NONE',  ( 0.06975647374412535795, 0.9975640502598243087, -0.000000000000000000 ) ) ;
#15371=( NAMED_UNIT ( * ) SI_UNIT ( $, .STERADIAN. ) SOLID_ANGLE_UNIT ( ) );
#15374=FILL_AREA_STYLE ('',( #23362 ) ) ;
#15401=MECHANICAL_DESIGN_GEOMETRIC_PRESENTATION_REPRESENTATION('',(#85610),#71265);
#15403=AXIS2_PLACEMENT_3D ( 'NONE', #9756, #57206, #40746 ) ;
#15408=VECTOR ( 'NONE', #88590, 1000.000000000000000 ) ;
#15430=AXIS2_PLACEMENT_3D ( 'NONE', #84923, #37965, #76437 ) ;
#15435=CARTESIAN_POINT ( 'NONE',  ( -5.320211218918606377, -24.96484130673365343, -3.999999999999999112 ) ) ;
#15462=CARTESIAN_POINT ( 'NONE',  ( 3.969999999999999751, 36.75000000000000000, -2.750000000000000000 ) ) ;
#15466=CARTESIAN_POINT ( 'NONE',  ( 4.721516313243696139, -3.620689210586685913, -3.999999999999998224 ) ) ;
#15474=CARTESIAN_POINT ( 'NONE',  ( -13.59072821818278065, 90.85999462608739918, 7.686992381056737322 ) ) ;
#15482=CARTESIAN_POINT ( 'NONE',  ( 5.429204171145670443, -28.64228857780832982, 2.500000000000000000 ) ) ;
#15484=EDGE_LOOP ( 'NONE', ( #32942, #50065, #14119, #30605 ) ) ;
#15499=CARTESIAN_POINT ( 'NONE',  ( 8.629999999999995453, 40.99999999999999289, 6.250000000000000000 ) ) ;
#15515=VERTEX_POINT ( 'NONE', #50564 ) ;
#15522=AXIS2_PLACEMENT_3D ( 'NONE', #83688, #15206, #45686 ) ;
#15530=ADVANCED_FACE ( 'NONE', ( #4589 ), #79592, .T. ) ;
#15537=FACE_OUTER_BOUND ( 'NONE', #72454, .T. ) ;
#15541=CARTESIAN_POINT ( 'NONE',  ( -6.868018881897137717, -58.39307134327864901, -3.749999999999999556 ) ) ;
#15542=ORIENTED_EDGE ( 'NONE', *, *, #15869, .T. ) ;
#15543=ORIENTED_EDGE ( 'NONE', *, *, #27469, .T. ) ;
#15548=CARTESIAN_POINT ( 'NONE',  ( -9.286179496275984491, 88.06418697516615168, -4.851265792414058531 ) ) ;
#15558=ORIENTED_EDGE ( 'NONE', *, *, #1003, .T. ) ;
#15560=EDGE_LOOP ( 'NONE', ( #96733, #76359, #664, #88824 ) ) ;
#15567=EDGE_CURVE ( 'NONE', #82021, #73831, #70657, .T. ) ;
#15569=COLOUR_RGB ( '', 0.72549020, 0.75294118, 0.79215686) ;
#15576=EDGE_CURVE ( 'NONE', #97363, #37672, #85892, .T. ) ;
#15584=ORIENTED_EDGE ( 'NONE', *, *, #78572, .T. ) ;
#15602=CARTESIAN_POINT ( 'NONE',  ( 6.880000000000007887, 41.24999999999999289, -6.250000000000000000 ) ) ;
#15603=MECHANICAL_DESIGN_GEOMETRIC_PRESENTATION_REPRESENTATION('',(#9234),#63534);
#15614=DIRECTION ( 'NONE',  ( -0.000000000000000000, 0.000000000000000000, 1.000000000000000000 ) ) ;
#15623=CYLINDRICAL_SURFACE ( 'NONE', #53217, 0.2500000000000002220 ) ;
#15636=DIRECTION ( 'NONE',  ( -1.000000000000000000, 0.000000000000000000, 0.000000000000000000 ) ) ;
#15638=VERTEX_POINT ( 'NONE', #66049 ) ;
#15642=FACE_OUTER_BOUND ( 'NONE', #91752, .T. ) ;
#15648=( NAMED_UNIT ( * ) SI_UNIT ( $, .STERADIAN. ) SOLID_ANGLE_UNIT ( ) );
#15652=EDGE_LOOP ( 'NONE', ( #34778, #33299, #29678, #6761 ) ) ;
#15659=CARTESIAN_POINT ( 'NONE',  ( -11.33435148538996096, -69.53340079812301155, 4.000000000000000000 ) ) ;
#15669=ORIENTED_EDGE ( 'NONE', *, *, #93405, .T. ) ;
#15680=EDGE_CURVE ( 'NONE', #52137, #43409, #84267, .T. ) ;
#15681=AXIS2_PLACEMENT_3D ( 'NONE', #49182, #64167, #20159 ) ;
#15689=AXIS2_PLACEMENT_3D ( 'NONE', #19127, #2189, #48143 ) ;
#15696=STYLED_ITEM ( 'NONE', ( #55732 ), #59598 ) ;
#15697=( GEOMETRIC_REPRESENTATION_CONTEXT ( 3 ) GLOBAL_UNCERTAINTY_ASSIGNED_CONTEXT ( ( #9233 ) ) GLOBAL_UNIT_ASSIGNED_CONTEXT ( ( #25621, #94590, #57082 ) ) REPRESENTATION_CONTEXT ( 'NONE', 'WORKASPACE' ) );
#15701=DIRECTION ( 'NONE',  ( 0.000000000000000000, -0.000000000000000000, -1.000000000000000000 ) ) ;
#15703=CARTESIAN_POINT ( 'NONE',  ( 8.630000001799311704, -0.01509713870841188424, 4.000000000000000000 ) ) ;
#15707=DIRECTION ( 'NONE',  ( -0.000000000000000000, -0.000000000000000000, -1.000000000000000000 ) ) ;
#15724=EDGE_CURVE ( 'NONE', #11101, #6373, #96576, .T. ) ;
#15726=EDGE_CURVE ( 'NONE', #44602, #51203, #58751, .T. ) ;
#15728=ORIENTED_EDGE ( 'NONE', *, *, #4857, .F. ) ;
#15742=CARTESIAN_POINT ( 'NONE',  ( -6.000000000000009770, 40.99999999999999289, 6.250000000000000000 ) ) ;
#15746=VERTEX_POINT ( 'NONE', #89054 ) ;
#15752=DIRECTION ( 'NONE',  ( 0.000000000000000000, -1.000000000000000000, 0.000000000000000000 ) ) ;
#15758=EDGE_CURVE ( 'NONE', #96487, #45519, #90035, .T. ) ;
#15759=CARTESIAN_POINT ( 'NONE',  ( 11.04400142293669518, -89.88311504651142059, -4.000000000000000000 ) ) ;
#15762=CARTESIAN_POINT ( 'NONE',  ( -9.000000000000001776, 83.89999999999994884, 0.000000000000000000 ) ) ;
#15768=EDGE_LOOP ( 'NONE', ( #39043, #58107, #45153, #40912 ) ) ;
#15776=CARTESIAN_POINT ( 'NONE',  ( 4.469999999999999751, 10.25000000000000000, -4.000000000000000000 ) ) ;
#15783=SURFACE_SIDE_STYLE ('',( #68293 ) ) ;
#15784=AXIS2_PLACEMENT_3D ( 'NONE', #47986, #86503, #18001 ) ;
#15785=ORIENTED_EDGE ( 'NONE', *, *, #36578, .F. ) ;
#15787=ORIENTED_EDGE ( 'NONE', *, *, #97123, .T. ) ;
#15793=FILL_AREA_STYLE_COLOUR ( '', #32924 ) ;
#15802=ORIENTED_EDGE ( 'NONE', *, *, #86156, .F. ) ;
#15806=CYLINDRICAL_SURFACE ( 'NONE', #76909, 1.249999999999987121 ) ;
#15807=DIRECTION ( 'NONE',  ( 0.000000000000000000, 0.000000000000000000, 1.000000000000000000 ) ) ;
#15812=DIRECTION ( 'NONE',  ( -0.000000000000000000, 0.000000000000000000, 1.000000000000000000 ) ) ;
#15827=SURFACE_STYLE_USAGE ( .BOTH. , #30806 ) ;
#15828=AXIS2_PLACEMENT_3D ( 'NONE', #16031, #62499, #92023 ) ;
#15835=SHAPE_REPRESENTATION_RELATIONSHIP ( 'NONE' , 'NONE' ,  #51695, #95471 ) ;
#15837=ADVANCED_FACE ( 'NONE', ( #81542 ), #97081, .T. ) ;
#15838=CARTESIAN_POINT ( 'NONE',  ( 6.033511671488541950, -36.04540650267416879, -2.750000000001608935 ) ) ;
#15847=SPHERICAL_SURFACE ( 'NONE', #17523, 0.2500000000000000000 ) ;
#15851=MECHANICAL_DESIGN_GEOMETRIC_PRESENTATION_REPRESENTATION('',(#3083),#30171);
#15853=CARTESIAN_POINT ( 'NONE',  ( -7.909660991811269248, -4.175919252832432704, -4.000000000000000000 ) ) ;
#15857=EDGE_LOOP ( 'NONE', ( #24737, #9115, #31855, #7982, #13692, #46537 ) ) ;
#15869=EDGE_CURVE ( 'NONE', #1559, #82102, #76321, .T. ) ;
#15905=DIRECTION ( 'NONE',  ( -0.000000000000000000, 0.000000000000000000, 1.000000000000000000 ) ) ;
#15909=CARTESIAN_POINT ( 'NONE',  ( -7.287667432647799259, -86.26780665046146623, -4.000000000000000000 ) ) ;
#15936=FACE_OUTER_BOUND ( 'NONE', #43012, .T. ) ;
#15939=CARTESIAN_POINT ( 'NONE',  ( 4.823525747195460234, -6.402798798525329182, -3.999999999999998224 ) ) ;
#15970=ADVANCED_FACE ( 'NONE', ( #16019 ), #39657, .T. ) ;
#15972=( LENGTH_UNIT ( ) NAMED_UNIT ( * ) SI_UNIT ( .MILLI., .METRE. ) );
#15976=CARTESIAN_POINT ( 'NONE',  ( 6.579634127946654587, -87.99828267815715321, 4.000000000000000000 ) ) ;
#15988=AXIS2_PLACEMENT_3D ( 'NONE', #54388, #16413, #16905 ) ;
#16000=ORIENTED_EDGE ( 'NONE', *, *, #87262, .T. ) ;
#16005=CARTESIAN_POINT ( 'NONE',  ( -7.750000000000000000, 41.24999999999999289, 4.250000000000000000 ) ) ;
#16007=DIRECTION ( 'NONE',  ( 1.000000000000000000, -0.000000000000000000, 0.000000000000000000 ) ) ;
#16011=CARTESIAN_POINT ( 'NONE',  ( -6.031993939708431895, -39.82530731230059473, -3.749999999998387512 ) ) ;
#16017=VECTOR ( 'NONE', #1096, 1000.000000000000000 ) ;
#16019=FACE_OUTER_BOUND ( 'NONE', #3523, .T. ) ;
#16031=CARTESIAN_POINT ( 'NONE',  ( 0.000000000000000000, 0.000000000000000000, 2.500000000000000000 ) ) ;
#16050=CIRCLE ( 'NONE', #73554, 1.000000000000000888 ) ;
#16055=AXIS2_PLACEMENT_3D ( 'NONE', #8905, #43823, #72842 ) ;
#16056=DIRECTION ( 'NONE',  ( 0.6246950475544238435, 0.7808688094430307203, 0.000000000000000000 ) ) ;
#16057=DIRECTION ( 'NONE',  ( 0.000000000000000000, 0.000000000000000000, 1.000000000000000000 ) ) ;
#16059=VERTEX_POINT ( 'NONE', #1536 ) ;
#16063=ORIENTED_EDGE ( 'NONE', *, *, #18847, .T. ) ;
#16065=DIRECTION ( 'NONE',  ( 0.000000000000000000, 0.000000000000000000, 1.000000000000000000 ) ) ;
#16067=VECTOR ( 'NONE', #63064, 999.9999999999998863 ) ;
#16081=AXIS2_PLACEMENT_3D ( 'NONE', #83210, #90203, #68221 ) ;
#16116=EDGE_CURVE ( 'NONE', #46764, #9418, #18479, .T. ) ;
#16118=CARTESIAN_POINT ( 'NONE',  ( 9.879999999999990123, 20.99999999999999645, 0.000000000000000000 ) ) ;
#16128=ORIENTED_EDGE ( 'NONE', *, *, #87707, .T. ) ;
#16134=CARTESIAN_POINT ( 'NONE',  ( -11.51383254012985802, -65.37322064360738239, 3.750000000000000000 ) ) ;
#16144=CARTESIAN_POINT ( 'NONE',  ( -5.999999999999994671, 43.00000000000000000, 4.250000000000000000 ) ) ;
#16146=( LENGTH_UNIT ( ) NAMED_UNIT ( * ) SI_UNIT ( .MILLI., .METRE. ) );
#16148=CIRCLE ( 'NONE', #54463, 0.2500000000000004441 ) ;
#16154=SURFACE_SIDE_STYLE ('',( #9139 ) ) ;
#16155=VECTOR ( 'NONE', #67863, 999.9999999999998863 ) ;
#16158=COLOUR_RGB ( '', 0.72549020, 0.75294118, 0.79215686) ;
#16171=CARTESIAN_POINT ( 'NONE',  ( -3.250000000000000444, 1.019547802438465656, 2.500000000000000000 ) ) ;
#16182=CARTESIAN_POINT ( 'NONE',  ( 8.900267494866982432, -1.043573704937230007, 4.000000000000000000 ) ) ;
#16190=LINE ( 'NONE', #84201, #79550 ) ;
#16232=CARTESIAN_POINT ( 'NONE',  ( 17.75000000000000000, 77.07179676972445748, 6.250000000000000000 ) ) ;
#16234=UNCERTAINTY_MEASURE_WITH_UNIT (LENGTH_MEASURE( 1.000000000000000082E-05 ), #80918, 'distance_accuracy_value', 'NONE');
#16246=CARTESIAN_POINT ( 'NONE',  ( -6.732636091893168029, -88.11213685669366669, 3.750000000000000000 ) ) ;
#16254=CARTESIAN_POINT ( 'NONE',  ( -10.88853822400146676, 46.97908644289115188, 3.000000000000000000 ) ) ;
#16265=ADVANCED_FACE ( 'NONE', ( #11461 ), #7749, .T. ) ;
#16270=CARTESIAN_POINT ( 'NONE',  ( -4.787219229848344249, -17.54708441702821631, 3.999999999999999112 ) ) ;
#16273=AXIS2_PLACEMENT_3D ( 'NONE', #14102, #13600, #5618 ) ;
#16276=ORIENTED_EDGE ( 'NONE', *, *, #89073, .F. ) ;
#16284=EDGE_CURVE ( 'NONE', #98330, #49831, #48475, .T. ) ;
#16289=VERTEX_POINT ( 'NONE', #56479 ) ;
#16293=DIRECTION ( 'NONE',  ( -2.107602052970794797E-16, 1.000000000000000000, -0.000000000000000000 ) ) ;
#16320=CARTESIAN_POINT ( 'NONE',  ( -10.17588876012433197, 89.26462023800682744, 5.905476706514949825 ) ) ;
#16321=CARTESIAN_POINT ( 'NONE',  ( 4.380000000000000782, 1.019547802438464768, -2.500000000000000000 ) ) ;
#16323=AXIS2_PLACEMENT_3D ( 'NONE', #54773, #64232, #79749 ) ;
#16325=( NAMED_UNIT ( * ) PLANE_ANGLE_UNIT ( ) SI_UNIT ( $, .RADIAN. ) );
#16334=LINE ( 'NONE', #45344, #49669 ) ;
#16337=CARTESIAN_POINT ( 'NONE',  ( -10.57486859793700873, -40.44919682093607349, -4.000000000000000000 ) ) ;
#16353=ORIENTED_EDGE ( 'NONE', *, *, #80768, .T. ) ;
#16354=DIRECTION ( 'NONE',  ( 2.569960705150826877E-16, -1.000000000000000000, 0.000000000000000000 ) ) ;
#16360=DIRECTION ( 'NONE',  ( 1.000000000000000000, 0.000000000000000000, 0.000000000000000000 ) ) ;
#16361=DIRECTION ( 'NONE',  ( -0.000000000000000000, -0.000000000000000000, -1.000000000000000000 ) ) ;
#16383=VERTEX_POINT ( 'NONE', #42950 ) ;
#16387=VERTEX_POINT ( 'NONE', #20944 ) ;
#16395=SURFACE_STYLE_USAGE ( .BOTH. , #69392 ) ;
#16402=STYLED_ITEM ( 'NONE', ( #57008 ), #48631 ) ;
#16412=DIRECTION ( 'NONE',  ( -0.000000000000000000, -0.000000000000000000, 1.000000000000000000 ) ) ;
#16413=DIRECTION ( 'NONE',  ( 0.000000000000000000, 0.000000000000000000, 1.000000000000000000 ) ) ;
#16416=VECTOR ( 'NONE', #12666, 1000.000000000000000 ) ;
#16419=VERTEX_POINT ( 'NONE', #12935 ) ;
#16430=CARTESIAN_POINT ( 'NONE',  ( -8.124115902427741176, 75.04369783535877048, 2.900000000000000355 ) ) ;
#16438=STYLED_ITEM ( 'NONE', ( #45192 ), #83936 ) ;
#16448=DIRECTION ( 'NONE',  ( 0.02970531260815257105, -0.9995586998285053149, -1.030610062851841046E-16 ) ) ;
#16449=CARTESIAN_POINT ( 'NONE',  ( 6.004190426492125532, -34.81345361117713111, -3.750000000000000888 ) ) ;
#16450=CARTESIAN_POINT ( 'NONE',  ( -7.750000000000000000, 80.07179676972448590, 6.250000000000000000 ) ) ;
#16462=ORIENTED_EDGE ( 'NONE', *, *, #2294, .F. ) ;
#16468=VECTOR ( 'NONE', #715, 1000.000000000000000 ) ;
#16476=EDGE_CURVE ( 'NONE', #69849, #89406, #1339, .T. ) ;
#16482=STYLED_ITEM ( 'NONE', ( #23332 ), #77518 ) ;
#16488=EDGE_CURVE ( 'NONE', #43409, #52137, #10944, .T. ) ;
#16491=CARTESIAN_POINT ( 'NONE',  ( -6.732636091893172470, -88.11213685669366669, 2.750000000000000000 ) ) ;
#16497=CARTESIAN_POINT ( 'NONE',  ( 6.579634127946608402, -87.99828267815712479, 2.750000000000000000 ) ) ;
#16501=LINE ( 'NONE', #8501, #35017 ) ;
#16512=AXIS2_PLACEMENT_3D ( 'NONE', #96655, #90973, #88633 ) ;
#16519=ADVANCED_FACE ( 'NONE', ( #22428 ), #80944, .F. ) ;
#16540=MECHANICAL_DESIGN_GEOMETRIC_PRESENTATION_REPRESENTATION('',(#42094),#72391);
#16542=EDGE_CURVE ( 'NONE', #44301, #5283, #67422, .T. ) ;
#16555=DIRECTION ( 'NONE',  ( 1.000000000000000000, 0.000000000000000000, 0.000000000000000000 ) ) ;
#16560=EDGE_LOOP ( 'NONE', ( #38709, #35163 ) ) ;
#16567=FILL_AREA_STYLE ('',( #77537 ) ) ;
#16571=VERTEX_POINT ( 'NONE', #14433 ) ;
#16576=SURFACE_STYLE_FILL_AREA ( #53081 ) ;
#16580=EDGE_LOOP ( 'NONE', ( #48582, #54977, #4717, #97486 ) ) ;
#16589=FILL_AREA_STYLE ('',( #77563 ) ) ;
#16594=DIRECTION ( 'NONE',  ( -0.5905099943842175847, -0.8070303256584298035, 0.000000000000000000 ) ) ;
#16596=CARTESIAN_POINT ( 'NONE',  ( -8.000000000000000000, 75.73428692542562146, 2.900000000000000355 ) ) ;
#16601=B_SPLINE_CURVE_WITH_KNOTS ( 'NONE', 3,
 ( #80420, #50398, #18439, #95922, #3932, #86927, #88901, #80908, #41456, #49909, #12402, #42908, #27403, #71923, #27893, #3444, #35396, #79913, #20411, #50897, #81392, #12894 ),
 .UNSPECIFIED., .F., .F.,
 ( 4, 2, 2, 2, 2, 2, 2, 2, 2, 2, 4 ),
 ( 0.000000000000000000, 0.005577272106129050298, 0.01115454421225810060, 0.02230908842451620119, 0.04461817684903233300, 0.05577272106129038676, 0.06692726527354844746, 0.07808180948580650815, 0.08365908159193553850, 0.08644771764500004674, 0.08923635369806456885 ),
 .UNSPECIFIED. ) ;
#16610=ORIENTED_EDGE ( 'NONE', *, *, #60064, .T. ) ;
#16614=FACE_OUTER_BOUND ( 'NONE', #14668, .T. ) ;
#16623=FACE_OUTER_BOUND ( 'NONE', #59185, .T. ) ;
#16628=EDGE_CURVE ( 'NONE', #58305, #3713, #27930, .T. ) ;
#16632=CARTESIAN_POINT ( 'NONE',  ( -7.858200837510024073, -3.137962441271501479, 4.000000000000000000 ) ) ;
#16638=ADVANCED_FACE ( 'NONE', ( #83902 ), #60896, .F. ) ;
#16659=VERTEX_POINT ( 'NONE', #46395 ) ;
#16661=DIRECTION ( 'NONE',  ( -0.000000000000000000, -1.000000000000000000, -0.000000000000000000 ) ) ;
#16672=AXIS2_PLACEMENT_3D ( 'NONE', #98981, #98485, #53434 ) ;
#16674=CARTESIAN_POINT ( 'NONE',  ( -3.585386599411522823, -2.690194976751941969, 2.500000000000404121 ) ) ;
#16676=CARTESIAN_POINT ( 'NONE',  ( 9.112672642667108747, -7.236390792799208604, 3.750000000000000000 ) ) ;
#16680=SURFACE_SIDE_STYLE ('',( #70173 ) ) ;
#16681=CARTESIAN_POINT ( 'NONE',  ( 11.49999999999999645, 75.00000000000000000, -6.500000000000000888 ) ) ;
#16701=DIRECTION ( 'NONE',  ( 1.000000000000000000, -0.000000000000000000, 0.000000000000000000 ) ) ;
#16712=MECHANICAL_DESIGN_GEOMETRIC_PRESENTATION_REPRESENTATION('',(#8781),#48666);
#16729=ORIENTED_EDGE ( 'NONE', *, *, #92831, .T. ) ;
#16731=CARTESIAN_POINT ( 'NONE',  ( 9.112669733836950670, -7.236323975091223382, -4.000000000000000000 ) ) ;
#16739=CARTESIAN_POINT ( 'NONE',  ( -3.999999999999999112, 78.07179676972445748, -6.250000000000000000 ) ) ;
#16760=ADVANCED_FACE ( 'NONE', ( #47368 ), #77866, .F. ) ;
#16763=CARTESIAN_POINT ( 'NONE',  ( -6.868018881897138606, -58.39307134327875559, 3.750000000000000444 ) ) ;
#16765=DIRECTION ( 'NONE',  ( -0.000000000000000000, -0.000000000000000000, -1.000000000000000000 ) ) ;
#16772=( LENGTH_UNIT ( ) NAMED_UNIT ( * ) SI_UNIT ( .MILLI., .METRE. ) );
#16778=ORIENTED_EDGE ( 'NONE', *, *, #92786, .F. ) ;
#16792=LINE ( 'NONE', #1805, #6866 ) ;
#16802=CIRCLE ( 'NONE', #50322, 0.2500000000000002220 ) ;
#16804=CARTESIAN_POINT ( 'NONE',  ( -7.079946191729883154, -69.52844198715558832, -2.750000000000000888 ) ) ;
#16815=FACE_OUTER_BOUND ( 'NONE', #20673, .T. ) ;
#16818=FILL_AREA_STYLE ('',( #17319 ) ) ;
#16824=CARTESIAN_POINT ( 'NONE',  ( -10.98829462902744680, 46.98606209026556968, 0.000000000000000000 ) ) ;
#16827=DIRECTION ( 'NONE',  ( -0.9975640502598257520, 0.06975647374410356982, 0.000000000000000000 ) ) ;
#16828=EDGE_CURVE ( 'NONE', #33199, #26706, #48841, .T. ) ;
#16829=( NAMED_UNIT ( * ) PLANE_ANGLE_UNIT ( ) SI_UNIT ( $, .RADIAN. ) );
#16847=CARTESIAN_POINT ( 'NONE',  ( -9.990730578767623271, 46.91630561652144138, 2.899999999999999467 ) ) ;
#16865=TOROIDAL_SURFACE ( 'NONE', #21648, 3.690000000000000391, 0.2500000000000000000 ) ;
#16894=STYLED_ITEM ( 'NONE', ( #15018 ), #86133 ) ;
#16895=CARTESIAN_POINT ( 'NONE',  ( -6.281451360760612168, -39.80862496263591055, -3.999999999999998224 ) ) ;
#16898=VERTEX_POINT ( 'NONE', #87340 ) ;
#16905=DIRECTION ( 'NONE',  ( 1.000000000000000000, 0.000000000000000000, 0.000000000000000000 ) ) ;
#16909=VECTOR ( 'NONE', #85688, 1000.000000000000000 ) ;
#16923=VECTOR ( 'NONE', #16701, 1000.000000000000000 ) ;
#16931=CARTESIAN_POINT ( 'NONE',  ( -13.77612262535527954, 90.93158326518027934, 7.883772450803742338 ) ) ;
#16942=CARTESIAN_POINT ( 'NONE',  ( 4.380000000000000782, 1.019547802438464545, 2.750000000000000000 ) ) ;
#16945=FACE_OUTER_BOUND ( 'NONE', #18151, .T. ) ;
#16953=CIRCLE ( 'NONE', #66399, 0.2500000000000002220 ) ;
#16955=EDGE_LOOP ( 'NONE', ( #3205, #68800, #25713, #12668 ) ) ;
#16966=DIRECTION ( 'NONE',  ( 0.06975647374412544122, 0.9975640502598241977, -0.000000000000000000 ) ) ;
#16969=DIRECTION ( 'NONE',  ( 0.000000000000000000, -0.000000000000000000, 1.000000000000000000 ) ) ;
#16980=EDGE_CURVE ( 'NONE', #45794, #79527, #64810, .T. ) ;
#17012=DIRECTION ( 'NONE',  ( 1.000000000000000000, 0.000000000000000000, 0.000000000000000000 ) ) ;
#17041=ORIENTED_EDGE ( 'NONE', *, *, #52861, .F. ) ;
#17048=( NAMED_UNIT ( * ) SI_UNIT ( $, .STERADIAN. ) SOLID_ANGLE_UNIT ( ) );
#17058=CARTESIAN_POINT ( 'NONE',  ( 4.630000000000003446, 1.019547802438464323, -3.750000000000000000 ) ) ;
#17067=ORIENTED_EDGE ( 'NONE', *, *, #33608, .F. ) ;
#17072=DIRECTION ( 'NONE',  ( -0.000000000000000000, 0.000000000000000000, 1.000000000000000000 ) ) ;
#17075=AXIS2_PLACEMENT_3D ( 'NONE', #39174, #1190, #31649 ) ;
#17079=VERTEX_POINT ( 'NONE', #10370 ) ;
#17090=LINE ( 'NONE', #1107, #54992 ) ;
#17098=CARTESIAN_POINT ( 'NONE',  ( -11.23896940083325013, -88.22260584720305587, 4.000000000000000000 ) ) ;
#17103=DIRECTION ( 'NONE',  ( -0.9961946980917462113, 0.08715574274765140739, -0.000000000000000000 ) ) ;
#17105=AXIS2_PLACEMENT_3D ( 'NONE', #58093, #58598, #27606 ) ;
#17125=AXIS2_PLACEMENT_3D ( 'NONE', #41535, #33987, #47539 ) ;
#17126=UNCERTAINTY_MEASURE_WITH_UNIT (LENGTH_MEASURE( 1.000000000000000082E-05 ), #1365, 'distance_accuracy_value', 'NONE');
#17127=DIRECTION ( 'NONE',  ( 1.000000000000000000, 0.000000000000000000, 0.000000000000000000 ) ) ;
#17136=DIRECTION ( 'NONE',  ( -0.000000000000000000, 0.000000000000000000, 1.000000000000000000 ) ) ;
#17148=ORIENTED_EDGE ( 'NONE', *, *, #95568, .F. ) ;
#17158=ORIENTED_EDGE ( 'NONE', *, *, #21840, .F. ) ;
#17170=EDGE_CURVE ( 'NONE', #70499, #63050, #37678, .T. ) ;
#17171=CARTESIAN_POINT ( 'NONE',  ( -18.89999999999999147, 91.00000000000000000, 7.750000000000000000 ) ) ;
#17179=FACE_OUTER_BOUND ( 'NONE', #98946, .T. ) ;
#17181=VECTOR ( 'NONE', #7082, 1000.000000000000000 ) ;
#17183=DIRECTION ( 'NONE',  ( 2.107602052970794797E-16, -1.000000000000000000, 0.000000000000000000 ) ) ;
#17195=AXIS2_PLACEMENT_3D ( 'NONE', #92977, #60514, #30994 ) ;
#17196=CARTESIAN_POINT ( 'NONE',  ( 4.920090861807432603, -13.81657824355479036, -2.750000000000000000 ) ) ;
#17214=DIRECTION ( 'NONE',  ( 1.000000000000000000, 0.000000000000000000, 0.000000000000000000 ) ) ;
#17231=VERTEX_POINT ( 'NONE', #97701 ) ;
#17232=CARTESIAN_POINT ( 'NONE',  ( 8.900267061692415993, -1.043551099208791966, -4.000000000000000000 ) ) ;
#17238=CARTESIAN_POINT ( 'NONE',  ( 14.99999999999998046, 70.25000000000000000, -6.250000000000000000 ) ) ;
#17242=CIRCLE ( 'NONE', #15681, 0.2500000000000002220 ) ;
#17261=CARTESIAN_POINT ( 'NONE',  ( -4.511928667084688094, -13.83795187542449412, 4.000000000000000000 ) ) ;
#17266=ORIENTED_EDGE ( 'NONE', *, *, #57339, .T. ) ;
#17270=VECTOR ( 'NONE', #50022, 1000.000000000000000 ) ;
#17276=ORIENTED_EDGE ( 'NONE', *, *, #21144, .T. ) ;
#17279=ORIENTED_EDGE ( 'NONE', *, *, #34885, .T. ) ;
#17288=ORIENTED_EDGE ( 'NONE', *, *, #93247, .T. ) ;
#17302=DIRECTION ( 'NONE',  ( 0.000000000000000000, 0.000000000000000000, 1.000000000000000000 ) ) ;
#17303=CARTESIAN_POINT ( 'NONE',  ( -4.536330484516918560, -17.54398402260299861, -2.750000000000000000 ) ) ;
#17312=EDGE_CURVE ( 'NONE', #47751, #5309, #26498, .T. ) ;
#17315=DIRECTION ( 'NONE',  ( 1.000000000000000000, 0.000000000000000000, 0.000000000000000000 ) ) ;
#17319=FILL_AREA_STYLE_COLOUR ( '', #64710 ) ;
#17329=COLOUR_RGB ( '', 0.66274510, 0.83137255, 0.94901961) ;
#17334=FACE_OUTER_BOUND ( 'NONE', #70409, .T. ) ;
#17339=CARTESIAN_POINT ( 'NONE',  ( 4.879999999999991900, 76.07179676972444327, 4.250000000000000000 ) ) ;
#17346=ORIENTED_EDGE ( 'NONE', *, *, #23549, .F. ) ;
#17347=CARTESIAN_POINT ( 'NONE',  ( -6.000000000000012434, 79.82179676972448590, -6.250000000000000000 ) ) ;
#17348=DIRECTION ( 'NONE',  ( 0.000000000000000000, -0.000000000000000000, -1.000000000000000000 ) ) ;
#17354=ADVANCED_FACE ( 'NONE', ( #76642 ), #83663, .T. ) ;
#17357=( LENGTH_UNIT ( ) NAMED_UNIT ( * ) SI_UNIT ( .MILLI., .METRE. ) );
#17368=DIRECTION ( 'NONE',  ( 0.7808688094430307203, -0.6246950475544238435, 0.000000000000000000 ) ) ;
#17378=ORIENTED_EDGE ( 'NONE', *, *, #73140, .T. ) ;
#17382=CARTESIAN_POINT ( 'NONE',  ( 18.00000000000000355, 73.00000000000001421, 6.250000000000000000 ) ) ;
#17406=CIRCLE ( 'NONE', #57266, 0.2500000000000002220 ) ;
#17411=EDGE_CURVE ( 'NONE', #60629, #6181, #16953, .T. ) ;
#17421=PRESENTATION_STYLE_ASSIGNMENT (( #944 ) ) ;
#17428=ORIENTED_EDGE ( 'NONE', *, *, #36807, .T. ) ;
#17431=EDGE_CURVE ( 'NONE', #13947, #48651, #48837, .T. ) ;
#17445=CARTESIAN_POINT ( 'NONE',  ( 4.380000000000000782, 0.09385850579273792571, 2.750000000000000000 ) ) ;
#17464=( LENGTH_UNIT ( ) NAMED_UNIT ( * ) SI_UNIT ( .MILLI., .METRE. ) );
#17475=ORIENTED_EDGE ( 'NONE', *, *, #33005, .T. ) ;
#17476=TOROIDAL_SURFACE ( 'NONE', #49354, 0.5000000000000000000, 0.2500000000000000000 ) ;
#17501=ORIENTED_EDGE ( 'NONE', *, *, #36990, .T. ) ;
#17503=MECHANICAL_DESIGN_GEOMETRIC_PRESENTATION_REPRESENTATION('',(#20701),#59013);
#17517=CARTESIAN_POINT ( 'NONE',  ( 12.30000000000000249, 99.99999999999998579, -8.000000000000000000 ) ) ;
#17519=FACE_OUTER_BOUND ( 'NONE', #26732, .T. ) ;
#17523=AXIS2_PLACEMENT_3D ( 'NONE', #52349, #30327, #76334 ) ;
#17533=EDGE_CURVE ( 'NONE', #4322, #33828, #29290, .T. ) ;
#17543=DIRECTION ( 'NONE',  ( 0.000000000000000000, 9.540979117872431131E-15, 1.000000000000000000 ) ) ;
#17557=AXIS2_PLACEMENT_3D ( 'NONE', #8362, #45368, #29864 ) ;
#17573=ORIENTED_EDGE ( 'NONE', *, *, #15567, .F. ) ;
#17594=DIRECTION ( 'NONE',  ( -0.000000000000000000, -0.000000000000000000, 1.000000000000000000 ) ) ;
#17599=LINE ( 'NONE', #87064, #73614 ) ;
#17605=CARTESIAN_POINT ( 'NONE',  ( 8.921421356237301481, 27.04185244743870697, 2.999999999999998668 ) ) ;
#17611=SURFACE_SIDE_STYLE ('',( #48081 ) ) ;
#17614=CARTESIAN_POINT ( 'NONE',  ( -6.732636091893170693, -88.11213685669366669, -2.750000000000000000 ) ) ;
#17617=ORIENTED_EDGE ( 'NONE', *, *, #72463, .F. ) ;
#17624=CARTESIAN_POINT ( 'NONE',  ( 11.34661744925197624, 54.08985607419764818, 2.900000000000000355 ) ) ;
#17639=ORIENTED_EDGE ( 'NONE', *, *, #95368, .F. ) ;
#17663=CARTESIAN_POINT ( 'NONE',  ( -3.500000000000000444, 1.019547802438453887, 2.750000000000000000 ) ) ;
#17666=PLANE ( 'NONE',  #22902 ) ;
#17669=CARTESIAN_POINT ( 'NONE',  ( -3.500000000000000444, 1.019547802438453887, 2.750000000000000000 ) ) ;
#17674=CARTESIAN_POINT ( 'NONE',  ( -0.5000000000000073275, 80.99999999999994316, -1.249999999999987121 ) ) ;
#17676=CYLINDRICAL_SURFACE ( 'NONE', #83173, 0.2500000000000002220 ) ;
#17694=VECTOR ( 'NONE', #29495, 1000.000000000000000 ) ;
#17720=DIRECTION ( 'NONE',  ( -1.000000000000000000, -2.569960705150826877E-16, 0.000000000000000000 ) ) ;
#17732=EDGE_LOOP ( 'NONE', ( #98471, #85004, #60041, #35568 ) ) ;
#17735=CARTESIAN_POINT ( 'NONE',  ( -18.89999999999999147, 91.25000000000000000, -8.000000000000000000 ) ) ;
#17741=DIRECTION ( 'NONE',  ( -1.000000000000000000, 0.000000000000000000, 0.000000000000000000 ) ) ;
#17745=DIRECTION ( 'NONE',  ( -1.000000000000000000, 0.000000000000000000, 0.000000000000000000 ) ) ;
#17749=ORIENTED_EDGE ( 'NONE', *, *, #49339, .F. ) ;
#17762=EDGE_CURVE ( 'NONE', #10214, #4322, #13809, .T. ) ;
#17764=ADVANCED_FACE ( 'NONE', ( #65306 ), #50308, .T. ) ;
#17789=SURFACE_STYLE_FILL_AREA ( #47278 ) ;
#17798=LINE ( 'NONE', #78286, #51864 ) ;
#17799=CIRCLE ( 'NONE', #22657, 0.2500000000000002220 ) ;
#17809=CARTESIAN_POINT ( 'NONE',  ( 3.969999999999999751, 36.75000000000000000, -2.750000000000000000 ) ) ;
#17814=CIRCLE ( 'NONE', #56145, 2.250000000000001332 ) ;
#17818=LINE ( 'NONE', #48300, #14846 ) ;
#17819=CARTESIAN_POINT ( 'NONE',  ( -8.636324037029986300, 86.94567068113131825, -4.522730969307667159 ) ) ;
#17834=CARTESIAN_POINT ( 'NONE',  ( 8.630000000000000782, 1.019547802438458550, -4.000000000000000000 ) ) ;
#17836=DIRECTION ( 'NONE',  ( 1.000000000000000000, 0.000000000000000000, 0.000000000000000000 ) ) ;
#17848=CARTESIAN_POINT ( 'NONE',  ( 11.10000000000000142, 98.49999999999998579, -8.525133428036873795 ) ) ;
#17868=DIRECTION ( 'NONE',  ( 1.000000000000000000, 0.000000000000000000, 0.000000000000000000 ) ) ;
#17873=EDGE_CURVE ( 'NONE', #93548, #10214, #23300, .T. ) ;
#17877=ORIENTED_EDGE ( 'NONE', *, *, #44488, .T. ) ;
#17901=CARTESIAN_POINT ( 'NONE',  ( -11.16113486365330587, -52.93448945038705489, 3.750000000000000444 ) ) ;
#17908=FACE_OUTER_BOUND ( 'NONE', #50832, .T. ) ;
#17911=SURFACE_STYLE_FILL_AREA ( #40425 ) ;
#17914=DIRECTION ( 'NONE',  ( -0.000000000000000000, -0.000000000000000000, 1.000000000000000000 ) ) ;
#17937=ORIENTED_EDGE ( 'NONE', *, *, #90627, .F. ) ;
#17939=CARTESIAN_POINT ( 'NONE',  ( -19.00000000000000000, 75.76920769491739804, 2.900000000000000355 ) ) ;
#17940=CARTESIAN_POINT ( 'NONE',  ( -5.328486666281219364, -28.65465727419595510, -2.500000000001614264 ) ) ;
#17943=( NAMED_UNIT ( * ) SI_UNIT ( $, .STERADIAN. ) SOLID_ANGLE_UNIT ( ) );
#17945=CARTESIAN_POINT ( 'NONE',  ( 4.380000001274070520, 0.08775168531748565870, -4.000000000000000000 ) ) ;
#17957=ORIENTED_EDGE ( 'NONE', *, *, #1732, .F. ) ;
#17961=DIRECTION ( 'NONE',  ( 2.569960705150826877E-16, -1.000000000000000000, 0.000000000000000000 ) ) ;
#17974=SURFACE_STYLE_FILL_AREA ( #79453 ) ;
#17985=CARTESIAN_POINT ( 'NONE',  ( -11.64999999999999680, 98.49999999999998579, -8.525133428036873795 ) ) ;
#17986=CIRCLE ( 'NONE', #5214, 0.2500000000000002220 ) ;
#17987=ORIENTED_EDGE ( 'NONE', *, *, #42164, .T. ) ;
#17988=VERTEX_POINT ( 'NONE', #91779 ) ;
#17991=ADVANCED_FACE ( 'NONE', ( #84295 ), #2633, .T. ) ;
#17998=CARTESIAN_POINT ( 'NONE',  ( -8.000000000000000000, 1.019547802438458550, -3.750000000000000000 ) ) ;
#18001=DIRECTION ( 'NONE',  ( 0.000000000000000000, 0.000000000000000000, 1.000000000000000000 ) ) ;
#18012=VECTOR ( 'NONE', #36718, 1000.000000000000000 ) ;
#18022=PRESENTATION_STYLE_ASSIGNMENT (( #55532 ) ) ;
#18028=MECHANICAL_DESIGN_GEOMETRIC_PRESENTATION_REPRESENTATION('',(#37163),#43491);
#18029=ORIENTED_EDGE ( 'NONE', *, *, #27641, .T. ) ;
#18030=CARTESIAN_POINT ( 'NONE',  ( 41.74544750096863055, 57.05211158465706944, -8.000000000000000000 ) ) ;
#18044=SURFACE_STYLE_USAGE ( .BOTH. , #86539 ) ;
#18061=EDGE_CURVE ( 'NONE', #86010, #76841, #36132, .T. ) ;
#18064=CARTESIAN_POINT ( 'NONE',  ( -10.79772875661416265, 89.74400587740485946, 6.349085400557794578 ) ) ;
#18066=( NAMED_UNIT ( * ) SI_UNIT ( $, .STERADIAN. ) SOLID_ANGLE_UNIT ( ) );
#18072=CIRCLE ( 'NONE', #79369, 0.5000000000000004441 ) ;
#18074=EDGE_CURVE ( 'NONE', #41505, #39745, #55412, .T. ) ;
#18077=AXIS2_PLACEMENT_3D ( 'NONE', #28705, #50215, #96737 ) ;
#18087=CARTESIAN_POINT ( 'NONE',  ( -3.585700563647884032, -2.697940300814421377, -3.750000000000000888 ) ) ;
#18088=( NAMED_UNIT ( * ) SI_UNIT ( $, .STERADIAN. ) SOLID_ANGLE_UNIT ( ) );
#18103=CARTESIAN_POINT ( 'NONE',  ( 15.00000000000000000, 77.07179676972447169, 4.250000000000000000 ) ) ;
#18106=VERTEX_POINT ( 'NONE', #72213 ) ;
#18134=FILL_AREA_STYLE_COLOUR ( '', #50229 ) ;
#18148=DIRECTION ( 'NONE',  ( 0.000000000000000000, 0.000000000000000000, 1.000000000000000000 ) ) ;
#18150=CARTESIAN_POINT ( 'NONE',  ( -3.250000000000000444, 1.019547802438453887, 2.500000000000000000 ) ) ;
#18151=EDGE_LOOP ( 'NONE', ( #9563, #88538, #7582, #86643 ) ) ;
#18152=CARTESIAN_POINT ( 'NONE',  ( 10.89309003818156718, -97.65096242258067605, 3.999999999994602096 ) ) ;
#18160=ORIENTED_EDGE ( 'NONE', *, *, #66533, .T. ) ;
#18163=FACE_OUTER_BOUND ( 'NONE', #40378, .T. ) ;
#18167=CARTESIAN_POINT ( 'NONE',  ( 6.757645195923023707, -58.31151720875058686, -2.750000000000000888 ) ) ;
#18168=MECHANICAL_DESIGN_GEOMETRIC_PRESENTATION_REPRESENTATION('',(#32574),#86832);
#18205=ORIENTED_EDGE ( 'NONE', *, *, #59715, .F. ) ;
#18206=CARTESIAN_POINT ( 'NONE',  ( 8.880000001778796559, -0.01161165531860094795, -4.000000000000000000 ) ) ;
#18207=CARTESIAN_POINT ( 'NONE',  ( 6.930493939446634499, -71.55570417525920845, 2.750000000000000000 ) ) ;
#18231=DIRECTION ( 'NONE',  ( 1.000000000000000000, -0.000000000000000000, -0.000000000000000000 ) ) ;
#18233=EDGE_CURVE ( 'NONE', #6181, #79829, #11715, .T. ) ;
#18235=CARTESIAN_POINT ( 'NONE',  ( -5.070949216186721564, -24.98410106516554308, 3.749999999997579714 ) ) ;
#18240=VERTEX_POINT ( 'NONE', #36190 ) ;
#18248=TOROIDAL_SURFACE ( 'NONE', #78900, 6.599999999999995204, 0.2500000000000000000 ) ;
#18250=ORIENTED_EDGE ( 'NONE', *, *, #75964, .F. ) ;
#18253=ORIENTED_EDGE ( 'NONE', *, *, #50359, .T. ) ;
#18263=( NAMED_UNIT ( * ) PLANE_ANGLE_UNIT ( ) SI_UNIT ( $, .RADIAN. ) );
#18272=DIRECTION ( 'NONE',  ( 1.000000000000000000, 2.107602052970794797E-16, -0.000000000000000000 ) ) ;
#18286=CARTESIAN_POINT ( 'NONE',  ( -9.538220187641574199, 88.39559135149089286, 5.063080553069074341 ) ) ;
#18288=EDGE_LOOP ( 'NONE', ( #82799, #11230, #22870, #85996 ) ) ;
#18295=FILL_AREA_STYLE ('',( #24823 ) ) ;
#18300=DIRECTION ( 'NONE',  ( -0.000000000000000000, 0.000000000000000000, 1.000000000000000000 ) ) ;
#18304=EDGE_CURVE ( 'NONE', #87018, #10746, #4928, .T. ) ;
#18309=DIRECTION ( 'NONE',  ( -1.000000000000000000, 0.000000000000000000, 0.000000000000000000 ) ) ;
#18310=CARTESIAN_POINT ( 'NONE',  ( 6.880000000000007887, 41.24999999999999289, -6.500000000000000888 ) ) ;
#18328=PRESENTATION_STYLE_ASSIGNMENT (( #2855 ) ) ;
#18336=MECHANICAL_DESIGN_GEOMETRIC_PRESENTATION_REPRESENTATION('',(#10343),#74190);
#18359=ORIENTED_EDGE ( 'NONE', *, *, #67868, .T. ) ;
#18373=AXIS2_PLACEMENT_3D ( 'NONE', #37298, #29762, #51293 ) ;
#18384=CIRCLE ( 'NONE', #74242, 0.09999999999999939493 ) ;
#18391=CARTESIAN_POINT ( 'NONE',  ( -10.85079341422219734, -98.11281374797032129, 3.750000000000000888 ) ) ;
#18399=FACE_OUTER_BOUND ( 'NONE', #12583, .T. ) ;
#18413=CARTESIAN_POINT ( 'NONE',  ( -15.00000000000004974, 91.00000000000000000, 7.750000000000000000 ) ) ;
#18428=AXIS2_PLACEMENT_3D ( 'NONE', #98278, #15752, #761 ) ;
#18431=CARTESIAN_POINT ( 'NONE',  ( -6.356892395138682872, -50.94284410517786910, -2.500000000000000000 ) ) ;
#18439=CARTESIAN_POINT ( 'NONE',  ( -7.322384435959395255, -84.40865712959148937, 3.999999999999999112 ) ) ;
#18441=AXIS2_PLACEMENT_3D ( 'NONE', #46061, #38079, #7587 ) ;
#18460=CYLINDRICAL_SURFACE ( 'NONE', #43029, 1.249999999999987121 ) ;
#18478=FACE_OUTER_BOUND ( 'NONE', #5821, .T. ) ;
#18479=LINE ( 'NONE', #50439, #26850 ) ;
#18484=CARTESIAN_POINT ( 'NONE',  ( -11.58008864090154688, -84.10931438318498010, -3.750000000000000444 ) ) ;
#18502=EDGE_LOOP ( 'NONE', ( #41140, #47514, #26704, #55378 ) ) ;
#18504=CARTESIAN_POINT ( 'NONE',  ( -3.250000000000000888, 0.08822490956012897512, 2.500000000000000000 ) ) ;
#18520=SPHERICAL_SURFACE ( 'NONE', #44213, 0.2500000000000000000 ) ;
#18522=UNCERTAINTY_MEASURE_WITH_UNIT (LENGTH_MEASURE( 1.000000000000000082E-05 ), #37169, 'distance_accuracy_value', 'NONE');
#18526=CARTESIAN_POINT ( 'NONE',  ( 4.629999999999999893, 4.857171655774867594E-16, -4.250000000000000000 ) ) ;
#18529=SURFACE_STYLE_FILL_AREA ( #78540 ) ;
#18530=ORIENTED_EDGE ( 'NONE', *, *, #74263, .F. ) ;
#18536=DIRECTION ( 'NONE',  ( -1.000000000000000000, 0.000000000000000000, -0.000000000000000000 ) ) ;
#18543=EDGE_CURVE ( 'NONE', #6107, #37093, #91160, .T. ) ;
#18550=DIRECTION ( 'NONE',  ( -0.5905099943842175847, -0.8070303256584298035, 0.000000000000000000 ) ) ;
#18553=EDGE_CURVE ( 'NONE', #92036, #40169, #35226, .T. ) ;
#18563=CARTESIAN_POINT ( 'NONE',  ( -10.67064208068036102, -97.55764508346746311, 4.000000000000000000 ) ) ;
#18567=CARTESIAN_POINT ( 'NONE',  ( 8.879999999999991900, 69.99999999999998579, -6.250000000000000000 ) ) ;
#18616=DIRECTION ( 'NONE',  ( -1.000000000000000000, -6.938893903907221278E-15, 0.000000000000000000 ) ) ;
#18627=FILL_AREA_STYLE ('',( #35593 ) ) ;
#18631=EDGE_CURVE ( 'NONE', #34917, #59039, #29657, .T. ) ;
#18632=DIRECTION ( 'NONE',  ( 0.000000000000000000, 1.000000000000000000, 0.000000000000000000 ) ) ;
#18636=CARTESIAN_POINT ( 'NONE',  ( 11.40632860306172702, -69.21585191270308712, 3.750000000000000000 ) ) ;
#18641=CARTESIAN_POINT ( 'NONE',  ( -5.112373461513591621, -25.53775085953292390, 3.750000000000000444 ) ) ;
#18642=VERTEX_POINT ( 'NONE', #14194 ) ;
#18644=CARTESIAN_POINT ( 'NONE',  ( 8.879999999999995453, 41.24999999999999289, 6.250000000000000000 ) ) ;
#18648=EDGE_LOOP ( 'NONE', ( #7795, #47485, #56642, #15584, #95017, #79024, #9383, #29334 ) ) ;
#18649=CYLINDRICAL_SURFACE ( 'NONE', #94287, 0.2500000000000002220 ) ;
#18652=DIRECTION ( 'NONE',  ( -1.000000000000000000, 0.000000000000000000, 0.000000000000000000 ) ) ;
#18661=ORIENTED_EDGE ( 'NONE', *, *, #10407, .F. ) ;
#18667=CIRCLE ( 'NONE', #84127, 0.09999999999999982514 ) ;
#18669=EDGE_CURVE ( 'NONE', #69653, #62017, #61632, .T. ) ;
#18676=DIRECTION ( 'NONE',  ( 1.000000000000000000, 0.000000000000000000, -0.000000000000000000 ) ) ;
#18693=CARTESIAN_POINT ( 'NONE',  ( -3.749999999999988010, -5.564482262735336175E-16, 4.000000000000000000 ) ) ;
#18698=DIRECTION ( 'NONE',  ( 0.000000000000000000, 0.000000000000000000, 1.000000000000000000 ) ) ;
#18699=CARTESIAN_POINT ( 'NONE',  ( 6.829574850499570360, -88.00372650123708240, 2.749999999999999556 ) ) ;
#18710=( LENGTH_UNIT ( ) NAMED_UNIT ( * ) SI_UNIT ( .MILLI., .METRE. ) );
#18724=MECHANICAL_DESIGN_GEOMETRIC_PRESENTATION_REPRESENTATION('',(#66596),#23585);
#18742=AXIS2_PLACEMENT_3D ( 'NONE', #18526, #39568, #31547 ) ;
#18753=LINE ( 'NONE', #65706, #28814 ) ;
#18759=FACE_OUTER_BOUND ( 'NONE', #48523, .T. ) ;
#18760=DIRECTION ( 'NONE',  ( 0.000000000000000000, 0.000000000000000000, 1.000000000000000000 ) ) ;
#18782=CARTESIAN_POINT ( 'NONE',  ( -11.82883858055346415, 90.33605471726345115, 7.015824399821311452 ) ) ;
#18796=EDGE_CURVE ( 'NONE', #12912, #70565, #72096, .T. ) ;
#18817=AXIS2_PLACEMENT_3D ( 'NONE', #71124, #63109, #24641 ) ;
#18820=FILL_AREA_STYLE_COLOUR ( '', #24115 ) ;
#18822=( NAMED_UNIT ( * ) PLANE_ANGLE_UNIT ( ) SI_UNIT ( $, .RADIAN. ) );
#18839=CARTESIAN_POINT ( 'NONE',  ( 4.221203097589939723, -3.619724449958656276, -2.500000000000000000 ) ) ;
#18847=EDGE_CURVE ( 'NONE', #28374, #69849, #81341, .T. ) ;
#18864=ORIENTED_EDGE ( 'NONE', *, *, #65570, .F. ) ;
#18876=EDGE_LOOP ( 'NONE', ( #10127, #44241, #6183, #27664 ) ) ;
#18880=VERTEX_POINT ( 'NONE', #55633 ) ;
#18886=DIRECTION ( 'NONE',  ( 0.000000000000000000, 0.000000000000000000, -1.000000000000000000 ) ) ;
#18889=DIRECTION ( 'NONE',  ( 0.9975640502598257520, -0.06975647374410356982, 0.000000000000000000 ) ) ;
#18891=AXIS2_PLACEMENT_3D ( 'NONE', #10573, #17103, #94555 ) ;
#18893=DIRECTION ( 'NONE',  ( -0.000000000000000000, 0.000000000000000000, 1.000000000000000000 ) ) ;
#18896=AXIS2_PLACEMENT_3D ( 'NONE', #34943, #78980, #94470 ) ;
#18922=DIRECTION ( 'NONE',  ( -0.000000000000000000, 0.000000000000000000, 1.000000000000000000 ) ) ;
#18923=ORIENTED_EDGE ( 'NONE', *, *, #62271, .T. ) ;
#18926=CARTESIAN_POINT ( 'NONE',  ( -4.535014064372608011, -17.52590857052054929, -2.750000000000000000 ) ) ;
#18931=CARTESIAN_POINT ( 'NONE',  ( -8.000000000000000000, 40.99999999999999289, 6.250000000000000000 ) ) ;
#18933=DIRECTION ( 'NONE',  ( 1.000000000000000000, -0.000000000000000000, 0.000000000000000000 ) ) ;
#18936=AXIS2_PLACEMENT_3D ( 'NONE', #85335, #31828, #62324 ) ;
#18963=ADVANCED_FACE ( 'NONE', ( #47635 ), #9141, .T. ) ;
#18978=CARTESIAN_POINT ( 'NONE',  ( -11.42220087045558330, -90.34422636326586087, -3.749999999999999556 ) ) ;
#18983=VERTEX_POINT ( 'NONE', #43563 ) ;
#18998=EDGE_CURVE ( 'NONE', #24577, #40665, #96587, .T. ) ;
#19013=DIRECTION ( 'NONE',  ( 1.000000000000000000, 0.000000000000000000, 0.000000000000000000 ) ) ;
#19021=CARTESIAN_POINT ( 'NONE',  ( -7.750000000000000000, 0.000000000000000000, -6.250000000000000000 ) ) ;
#19031=CIRCLE ( 'NONE', #55790, 0.1000000000000001166 ) ;
#19032=CARTESIAN_POINT ( 'NONE',  ( 18.00000000000000000, 78.80384757729336798, 3.750000000000000000 ) ) ;
#19047=CARTESIAN_POINT ( 'NONE',  ( -5.078940136053648580, -28.66985681914853146, -2.500000000000000000 ) ) ;
#19052=AXIS2_PLACEMENT_3D ( 'NONE', #75577, #37591, #1080 ) ;
#19057=CARTESIAN_POINT ( 'NONE',  ( 18.00000000000000000, 77.07179676972447169, -4.250000000000000000 ) ) ;
#19070=AXIS2_PLACEMENT_3D ( 'NONE', #74853, #42393, #36863 ) ;
#19075=AXIS2_PLACEMENT_3D ( 'NONE', #58379, #87051, #13893 ) ;
#19078=CARTESIAN_POINT ( 'NONE',  ( -3.500000001642929792, 0.08393865083518964321, -4.000000000003232081 ) ) ;
#19106=ORIENTED_EDGE ( 'NONE', *, *, #16488, .F. ) ;
#19111=DIRECTION ( 'NONE',  ( -0.9975640502598243087, 0.06975647374412544122, 0.000000000000000000 ) ) ;
#19113=TOROIDAL_SURFACE ( 'NONE', #41550, 2.899999999999999467, 0.1000000000000000056 ) ;
#19115=CARTESIAN_POINT ( 'NONE',  ( -8.000000000000000000, 80.99999999999994316, 0.000000000000000000 ) ) ;
#19119=CARTESIAN_POINT ( 'NONE',  ( 9.479672251299419372, -19.63639846205726158, 4.000000000000000000 ) ) ;
#19123=CARTESIAN_POINT ( 'NONE',  ( -4.247994584727555534, -13.56436116443237516, 2.750000000000000000 ) ) ;
#19125=CIRCLE ( 'NONE', #4733, 2.900000000000002576 ) ;
#19126=EDGE_CURVE ( 'NONE', #14813, #105, #74880, .T. ) ;
#19127=CARTESIAN_POINT ( 'NONE',  ( -4.250000000000000000, 10.25000000000000000, 3.750000000000000000 ) ) ;
#19132=DIRECTION ( 'NONE',  ( 0.9961946980917462113, -0.08715574274765140739, 0.000000000000000000 ) ) ;
#19133=ORIENTED_EDGE ( 'NONE', *, *, #34208, .F. ) ;
#19141=( LENGTH_UNIT ( ) NAMED_UNIT ( * ) SI_UNIT ( .MILLI., .METRE. ) );
#19159=CARTESIAN_POINT ( 'NONE',  ( -11.02864780780833520, -96.54579228622785081, -3.999999999999996891 ) ) ;
#19178=CARTESIAN_POINT ( 'NONE',  ( 4.526800700887880780, -5.190657137169758073, 3.750000000000001776 ) ) ;
#19185=FACE_OUTER_BOUND ( 'NONE', #29299, .T. ) ;
#19187=STYLED_ITEM ( 'NONE', ( #33246 ), #28482 ) ;
#19210=ORIENTED_EDGE ( 'NONE', *, *, #51136, .T. ) ;
#19212=ORIENTED_EDGE ( 'NONE', *, *, #15567, .T. ) ;
#19227=EDGE_CURVE ( 'NONE', #89066, #29532, #55877, .T. ) ;
#19238=CARTESIAN_POINT ( 'NONE',  ( -3.750000000000000000, 10.25000000000000000, -2.750000000000000000 ) ) ;
#19256=EDGE_CURVE ( 'NONE', #35385, #63050, #70227, .T. ) ;
#19260=CARTESIAN_POINT ( 'NONE',  ( -11.13303098458958296, 89.96146600687833939, 6.578309274437964760 ) ) ;
#19264=CARTESIAN_POINT ( 'NONE',  ( 5.800000000000003375, 99.99999999999998579, 8.000000000000000000 ) ) ;
#19273=DIRECTION ( 'NONE',  ( 1.000000000000000000, 0.000000000000000000, 0.000000000000000000 ) ) ;
#19277=( NAMED_UNIT ( * ) SI_UNIT ( $, .STERADIAN. ) SOLID_ANGLE_UNIT ( ) );
#19286=CARTESIAN_POINT ( 'NONE',  ( -6.430724159521290950, -88.51069574204372259, -3.750000000000000000 ) ) ;
#19295=ORIENTED_EDGE ( 'NONE', *, *, #43911, .T. ) ;
#19303=CARTESIAN_POINT ( 'NONE',  ( 11.19532855855632292, -77.48518070178161565, -3.999999999999999112 ) ) ;
#19312=FILL_AREA_STYLE ('',( #35289 ) ) ;
#19319=ADVANCED_FACE ( 'NONE', ( #19909 ), #81883, .T. ) ;
#19324=MECHANICAL_DESIGN_GEOMETRIC_PRESENTATION_REPRESENTATION('',(#8123),#54502);
#19328=FILL_AREA_STYLE ('',( #89302 ) ) ;
#19329=ORIENTED_EDGE ( 'NONE', *, *, #30598, .F. ) ;
#19332=ORIENTED_EDGE ( 'NONE', *, *, #86156, .T. ) ;
#19346=VERTEX_POINT ( 'NONE', #13395 ) ;
#19364=EDGE_LOOP ( 'NONE', ( #85820, #84549, #87998, #63599 ) ) ;
#19368=ORIENTED_EDGE ( 'NONE', *, *, #40332, .F. ) ;
#19375=DIRECTION ( 'NONE',  ( 0.000000000000000000, 0.000000000000000000, -1.000000000000000000 ) ) ;
#19381=AXIS2_PLACEMENT_3D ( 'NONE', #53483, #29488, #45492 ) ;
#19393=VECTOR ( 'NONE', #11570, 1000.000000000000000 ) ;
#19399=CARTESIAN_POINT ( 'NONE',  ( 8.880000000000000782, 1.019547802438458550, 3.750000000000000000 ) ) ;
#19404=ORIENTED_EDGE ( 'NONE', *, *, #6341, .T. ) ;
#19410=CYLINDRICAL_SURFACE ( 'NONE', #60818, 3.940000000000000835 ) ;
#19414=CARTESIAN_POINT ( 'NONE',  ( 6.034747819232443078, -36.07388523689489546, -3.750000000000000000 ) ) ;
#19416=DIRECTION ( 'NONE',  ( 0.000000000000000000, -0.000000000000000000, -1.000000000000000000 ) ) ;
#19419=CARTESIAN_POINT ( 'NONE',  ( 8.629999999999995453, 41.24999999999999289, 6.250000000000000000 ) ) ;
#19430=UNCERTAINTY_MEASURE_WITH_UNIT (LENGTH_MEASURE( 1.000000000000000082E-05 ), #27753, 'distance_accuracy_value', 'NONE');
#19439=DIRECTION ( 'NONE',  ( 0.000000000000000000, 0.000000000000000000, -1.000000000000000000 ) ) ;
#19442=CARTESIAN_POINT ( 'NONE',  ( -15.00000000000004974, 91.00000000000000000, -7.750000000000000000 ) ) ;
#19453=VECTOR ( 'NONE', #83520, 1000.000000000000000 ) ;
#19478=ADVANCED_FACE ( 'NONE', ( #76367, #30857 ), #46360, .T. ) ;
#19480=ORIENTED_EDGE ( 'NONE', *, *, #16628, .T. ) ;
#19485=ORIENTED_EDGE ( 'NONE', *, *, #4128, .F. ) ;
#19495=AXIS2_PLACEMENT_3D ( 'NONE', #43278, #74257, #57783 ) ;
#19496=DIRECTION ( 'NONE',  ( 0.8070303256584298035, -0.5905099943842175847, 0.000000000000000000 ) ) ;
#19502=UNCERTAINTY_MEASURE_WITH_UNIT (LENGTH_MEASURE( 1.000000000000000082E-05 ), #89351, 'distance_accuracy_value', 'NONE');
#19507=SURFACE_STYLE_FILL_AREA ( #80509 ) ;
#19526=CARTESIAN_POINT ( 'NONE',  ( 14.99999999999997868, 80.07179676972448590, -6.250000000000000000 ) ) ;
#19534=CARTESIAN_POINT ( 'NONE',  ( -5.559536763064314435, -36.09058695999160449, -2.500000000000000444 ) ) ;
#19537=AXIS2_PLACEMENT_3D ( 'NONE', #7505, #37996, #69464 ) ;
#19544=CARTESIAN_POINT ( 'NONE',  ( 17.99999999999999645, 78.24875198621546701, -3.965855704038845353 ) ) ;
#19553=ORIENTED_EDGE ( 'NONE', *, *, #50727, .T. ) ;
#19566=DIRECTION ( 'NONE',  ( 1.000000000000000000, 0.000000000000000000, 0.000000000000000000 ) ) ;
#19573=CARTESIAN_POINT ( 'NONE',  ( -13.57315748652532506, 90.98139137973063839, 7.967914335234096868 ) ) ;
#19598=EDGE_LOOP ( 'NONE', ( #36662, #83501, #7692, #56089 ) ) ;
#19605=DIRECTION ( 'NONE',  ( -0.000000000000000000, 0.000000000000000000, 1.000000000000000000 ) ) ;
#19608=CARTESIAN_POINT ( 'NONE',  ( 6.599999999999995204, -97.00000000000000000, 4.000000000000000000 ) ) ;
#19611=CARTESIAN_POINT ( 'NONE',  ( 10.93144397341777641, -92.98246991214814727, 4.000000000000000000 ) ) ;
#19614=CARTESIAN_POINT ( 'NONE',  ( -7.118731320094870973, -71.92838106472885329, 2.750000000000000000 ) ) ;
#19617=CARTESIAN_POINT ( 'NONE',  ( -6.982525766850297799, -88.11956318484570261, 3.750000000000000000 ) ) ;
#19622=ORIENTED_EDGE ( 'NONE', *, *, #66533, .F. ) ;
#19634=VECTOR ( 'NONE', #94244, 1000.000000000000000 ) ;
#19644=DIRECTION ( 'NONE',  ( 0.000000000000000000, 0.000000000000000000, 1.000000000000000000 ) ) ;
#19652=CARTESIAN_POINT ( 'NONE',  ( 3.969999999999999751, 9.750000000000000000, 4.000000000000000000 ) ) ;
#19654=CARTESIAN_POINT ( 'NONE',  ( 6.829574850505127692, -88.00372650098204019, -3.749999999999998668 ) ) ;
#19659=EDGE_CURVE ( 'NONE', #15178, #37810, #47865, .T. ) ;
#19665=EDGE_CURVE ( 'NONE', #42611, #67453, #68383, .T. ) ;
#19677=TOROIDAL_SURFACE ( 'NONE', #11686, 0.5000000000000000000, 0.2500000000000000000 ) ;
#19681=SURFACE_STYLE_USAGE ( .BOTH. , #35161 ) ;
#19692=CARTESIAN_POINT ( 'NONE',  ( -10.77730536144846774, -98.63085534186637915, 4.000000000000001776 ) ) ;
#19699=DIRECTION ( 'NONE',  ( 0.000000000000000000, -0.000000000000000000, -1.000000000000000000 ) ) ;
#19701=ORIENTED_EDGE ( 'NONE', *, *, #58687, .F. ) ;
#19702=( LENGTH_UNIT ( ) NAMED_UNIT ( * ) SI_UNIT ( .MILLI., .METRE. ) );
#19708=EDGE_CURVE ( 'NONE', #88687, #21472, #94250, .T. ) ;
#19711=AXIS2_PLACEMENT_3D ( 'NONE', #62394, #14966, #92415 ) ;
#19714=ORIENTED_EDGE ( 'NONE', *, *, #16542, .F. ) ;
#19716=VERTEX_POINT ( 'NONE', #60862 ) ;
#19727=AXIS2_PLACEMENT_3D ( 'NONE', #29366, #96916, #35886 ) ;
#19728=CARTESIAN_POINT ( 'NONE',  ( 8.629999999999995453, 40.99999999999999289, -6.500000000000000888 ) ) ;
#19734=DIRECTION ( 'NONE',  ( 1.000000000000000000, 0.000000000000000000, 0.000000000000000000 ) ) ;
#19751=DIRECTION ( 'NONE',  ( 0.000000000000000000, 1.000000000000000000, 0.000000000000000000 ) ) ;
#19758=DIRECTION ( 'NONE',  ( 1.000000000000000000, 0.000000000000000000, 0.000000000000000000 ) ) ;
#19761=LINE ( 'NONE', #80761, #49524 ) ;
#19765=CARTESIAN_POINT ( 'NONE',  ( 6.829574850505126804, -88.00372650098204019, 3.750000000000001332 ) ) ;
#19769=CARTESIAN_POINT ( 'NONE',  ( -7.079957095331153916, -69.52918543726779887, 2.749999999999999112 ) ) ;
#19787=CARTESIAN_POINT ( 'NONE',  ( 10.85665724878298377, -52.68265776536580347, -4.000000000000000888 ) ) ;
#19803=DIRECTION ( 'NONE',  ( 1.000000000000000000, 0.000000000000000000, 0.000000000000000000 ) ) ;
#19817=DIRECTION ( 'NONE',  ( 0.5150380749100554878, 0.000000000000000000, -0.8571673007021115565 ) ) ;
#19818=ADVANCED_FACE ( 'NONE', ( #2360 ), #78323, .T. ) ;
#19819=CARTESIAN_POINT ( 'NONE',  ( 49.67841921735763577, 67.89383959705537563, -8.000000000000000000 ) ) ;
#19824=DIRECTION ( 'NONE',  ( 1.000000000000000000, 1.759564384940674839E-15, 0.000000000000000000 ) ) ;
#19851=CARTESIAN_POINT ( 'NONE',  ( -13.80105244024794331, 90.89655890636515778, -7.750000000004162892 ) ) ;
#19854=DIRECTION ( 'NONE',  ( -0.000000000000000000, 0.000000000000000000, 1.000000000000000000 ) ) ;
#19872=VECTOR ( 'NONE', #6126, 1000.000000000000000 ) ;
#19879=AXIS2_PLACEMENT_3D ( 'NONE', #88735, #34240, #19751 ) ;
#19894=CARTESIAN_POINT ( 'NONE',  ( -7.116252256210342964, -80.68108970088772480, -2.499999999998790745 ) ) ;
#19902=VERTEX_POINT ( 'NONE', #39362 ) ;
#19904=CARTESIAN_POINT ( 'NONE',  ( 6.910361961633475936, -84.29457034760254430, -3.750000000000000000 ) ) ;
#19909=FACE_OUTER_BOUND ( 'NONE', #62254, .T. ) ;
#19917=SURFACE_STYLE_USAGE ( .BOTH. , #57904 ) ;
#19943=( NAMED_UNIT ( * ) SI_UNIT ( $, .STERADIAN. ) SOLID_ANGLE_UNIT ( ) );
#19949=AXIS2_PLACEMENT_3D ( 'NONE', #60810, #84808, #92303 ) ;
#19952=CARTESIAN_POINT ( 'NONE',  ( 0.000000000000000000, 91.00000000000000000, 8.000000000000000000 ) ) ;
#19964=VERTEX_POINT ( 'NONE', #55332 ) ;
#19976=CIRCLE ( 'NONE', #88634, 0.2500000000000024980 ) ;
#19979=FACE_OUTER_BOUND ( 'NONE', #54215, .T. ) ;
#19984=FACE_OUTER_BOUND ( 'NONE', #47251, .T. ) ;
#19986=ORIENTED_EDGE ( 'NONE', *, *, #98245, .T. ) ;
#19999=AXIS2_PLACEMENT_3D ( 'NONE', #31771, #7818, #38313 ) ;
#20021=CARTESIAN_POINT ( 'NONE',  ( -7.750000000000000000, 40.74999999999999289, -4.000000000000000000 ) ) ;
#20026=ORIENTED_EDGE ( 'NONE', *, *, #41296, .T. ) ;
#20031=CARTESIAN_POINT ( 'NONE',  ( 18.00000000000000000, 77.62863618567965318, -4.012044701513177714 ) ) ;
#20038=SURFACE_SIDE_STYLE ('',( #51028 ) ) ;
#20060=AXIS2_PLACEMENT_3D ( 'NONE', #80779, #73757, #58249 ) ;
#20065=DIRECTION ( 'NONE',  ( 1.000000000000000000, 0.000000000000000000, 0.000000000000000000 ) ) ;
#20070=ORIENTED_EDGE ( 'NONE', *, *, #44531, .F. ) ;
#20072=SURFACE_STYLE_USAGE ( .BOTH. , #88072 ) ;
#20078=PRESENTATION_STYLE_ASSIGNMENT (( #95596 ) ) ;
#20083=VECTOR ( 'NONE', #36357, 999.9999999999998863 ) ;
#20094=DIRECTION ( 'NONE',  ( -0.000000000000000000, -0.000000000000000000, -1.000000000000000000 ) ) ;
#20097=SURFACE_STYLE_FILL_AREA ( #26609 ) ;
#20104=EDGE_CURVE ( 'NONE', #3713, #97731, #68134, .T. ) ;
#20105=DIRECTION ( 'NONE',  ( 0.000000000000000000, -0.000000000000000000, 1.000000000000000000 ) ) ;
#20112=EDGE_LOOP ( 'NONE', ( #95339, #27204, #77619, #28312 ) ) ;
#20113=CARTESIAN_POINT ( 'NONE',  ( -8.124115902427742952, 75.04369783535877048, -3.000000000000000000 ) ) ;
#20129=CARTESIAN_POINT ( 'NONE',  ( -5.112373461513591621, -25.53775085953292390, -2.750000000000000444 ) ) ;
#20143=CARTESIAN_POINT ( 'NONE',  ( 6.935110064710753974, -80.58145365566650753, -3.750000000000002665 ) ) ;
#20144=STYLED_ITEM ( 'NONE', ( #67915 ), #36713 ) ;
#20146=COLOUR_RGB ( '', 0.31764706, 0.68627451, 0.89019608) ;
#20152=UNCERTAINTY_MEASURE_WITH_UNIT (LENGTH_MEASURE( 1.000000000000000082E-05 ), #19702, 'distance_accuracy_value', 'NONE');
#20156=VERTEX_POINT ( 'NONE', #51276 ) ;
#20159=DIRECTION ( 'NONE',  ( 1.000000000000000000, 0.000000000000000000, 0.000000000000000000 ) ) ;
#20167=AXIS2_PLACEMENT_3D ( 'NONE', #53699, #68712, #60704 ) ;
#20169=LINE ( 'NONE', #35667, #59292 ) ;
#20177=MECHANICAL_DESIGN_GEOMETRIC_PRESENTATION_REPRESENTATION('',(#13832),#80843);
#20182=SURFACE_STYLE_USAGE ( .BOTH. , #88674 ) ;
#20204=AXIS2_PLACEMENT_3D ( 'NONE', #87456, #72441, #49450 ) ;
#20222=FILL_AREA_STYLE ('',( #88712 ) ) ;
#20240=AXIS2_PLACEMENT_3D ( 'NONE', #28885, #75884, #66403 ) ;
#20247=CIRCLE ( 'NONE', #33016, 0.2500000000000002220 ) ;
#20248=CARTESIAN_POINT ( 'NONE',  ( -13.39911793698215270, 90.87255582226832473, 7.784798940734791728 ) ) ;
#20252=CARTESIAN_POINT ( 'NONE',  ( -4.000000000000000000, 10.00000000000000000, -2.500000000000000000 ) ) ;
#20262=FILL_AREA_STYLE ('',( #57263 ) ) ;
#20266=CARTESIAN_POINT ( 'NONE',  ( 6.575034241980325156, -50.89776066942204835, 3.750000000000000000 ) ) ;
#20267=SURFACE_SIDE_STYLE ('',( #58237 ) ) ;
#20272=PLANE ( 'NONE',  #9022 ) ;
#20276=CARTESIAN_POINT ( 'NONE',  ( -10.80370554825945284, 89.74834511847251406, -6.353281608588780216 ) ) ;
#20281=ORIENTED_EDGE ( 'NONE', *, *, #4005, .T. ) ;
#20292=CARTESIAN_POINT ( 'NONE',  ( -9.000000000000001776, 80.99999999999994316, 0.000000000000000000 ) ) ;
#20301=DIRECTION ( 'NONE',  ( 0.000000000000000000, -1.000000000000000000, 0.000000000000000000 ) ) ;
#20316=CARTESIAN_POINT ( 'NONE',  ( 14.99999999999997868, 80.32179676972448590, 4.250000000000000000 ) ) ;
#20317=EDGE_LOOP ( 'NONE', ( #90556, #65999, #49993, #92332 ) ) ;
#20334=ORIENTED_EDGE ( 'NONE', *, *, #51018, .F. ) ;
#20389=CARTESIAN_POINT ( 'NONE',  ( 8.629999999999995453, 40.74999999999999289, -4.250000000000000000 ) ) ;
#20390=EDGE_CURVE ( 'NONE', #52732, #22085, #30379, .T. ) ;
#20393=CIRCLE ( 'NONE', #41109, 0.2500000000000002220 ) ;
#20394=CARTESIAN_POINT ( 'NONE',  ( 12.30000000000000249, 99.99999999999998579, -8.525133428036873795 ) ) ;
#20396=ORIENTED_EDGE ( 'NONE', *, *, #34208, .T. ) ;
#20399=CARTESIAN_POINT ( 'NONE',  ( -7.124975165218884854, -78.82169502743931844, -2.500000000000000000 ) ) ;
#20408=CARTESIAN_POINT ( 'NONE',  ( -11.37644997956084936, -81.99697149678695496, -4.000000000000000888 ) ) ;
#20411=CARTESIAN_POINT ( 'NONE',  ( -3.836041483939800933, -2.701055130266049265, 4.000000000000000000 ) ) ;
#20421=DIRECTION ( 'NONE',  ( -1.000000000000000000, 0.000000000000000000, -0.000000000000000000 ) ) ;
#20428=DIRECTION ( 'NONE',  ( -0.000000000000000000, 0.000000000000000000, 1.000000000000000000 ) ) ;
#20442=ORIENTED_EDGE ( 'NONE', *, *, #67066, .T. ) ;
#20454=VERTEX_POINT ( 'NONE', #78086 ) ;
#20457=CIRCLE ( 'NONE', #90747, 0.1000000000000001166 ) ;
#20466=CIRCLE ( 'NONE', #30015, 1.249999999999987121 ) ;
#20481=CARTESIAN_POINT ( 'NONE',  ( -6.874974626955391521, -78.82095024088569346, 2.500000000000000000 ) ) ;
#20492=UNCERTAINTY_MEASURE_WITH_UNIT (LENGTH_MEASURE( 1.000000000000000082E-05 ), #9055, 'distance_accuracy_value', 'NONE');
#20500=AXIS2_PLACEMENT_3D ( 'NONE', #27276, #65767, #26790 ) ;
#20509=ADVANCED_FACE ( 'NONE', ( #9590 ), #70593, .T. ) ;
#20523=CARTESIAN_POINT ( 'NONE',  ( -6.874984555098657246, -78.81798443069058635, -2.499999999999999112 ) ) ;
#20528=( NAMED_UNIT ( * ) SI_UNIT ( $, .STERADIAN. ) SOLID_ANGLE_UNIT ( ) );
#20534=PRESENTATION_STYLE_ASSIGNMENT (( #43031 ) ) ;
#20535=COLOUR_RGB ( '', 0.31764706, 0.68627451, 0.89019608) ;
#20543=LINE ( 'NONE', #88038, #3410 ) ;
#20556=DIRECTION ( 'NONE',  ( 0.000000000000000000, 0.000000000000000000, -1.000000000000000000 ) ) ;
#20558=CARTESIAN_POINT ( 'NONE',  ( 9.209947446681445271, -9.314274491706216352, -3.750000000000000444 ) ) ;
#20598=( GEOMETRIC_REPRESENTATION_CONTEXT ( 3 ) GLOBAL_UNCERTAINTY_ASSIGNED_CONTEXT ( ( #24234 ) ) GLOBAL_UNIT_ASSIGNED_CONTEXT ( ( #60767, #53269, #67795 ) ) REPRESENTATION_CONTEXT ( 'NONE', 'WORKASPACE' ) );
#20636=DIRECTION ( 'NONE',  ( 1.000000000000000000, 0.000000000000000000, 0.000000000000000000 ) ) ;
#20642=CARTESIAN_POINT ( 'NONE',  ( -10.95083791927332051, -94.44918831363982292, -4.000000000000000000 ) ) ;
#20647=CARTESIAN_POINT ( 'NONE',  ( 14.99999999999997691, 80.32179676972448590, 4.000000000000000000 ) ) ;
#20667=EDGE_CURVE ( 'NONE', #93500, #71973, #98957, .T. ) ;
#20673=EDGE_LOOP ( 'NONE', ( #88088, #66176, #84875, #89987 ) ) ;
#20675=FACE_OUTER_BOUND ( 'NONE', #42187, .T. ) ;
#20682=FACE_OUTER_BOUND ( 'NONE', #36712, .T. ) ;
#20696=ORIENTED_EDGE ( 'NONE', *, *, #24985, .F. ) ;
#20701=STYLED_ITEM ( 'NONE', ( #70484 ), #27325 ) ;
#20722=CIRCLE ( 'NONE', #76602, 0.2500000000000002220 ) ;
#20726=( NAMED_UNIT ( * ) PLANE_ANGLE_UNIT ( ) SI_UNIT ( $, .RADIAN. ) );
#20729=VERTEX_POINT ( 'NONE', #57540 ) ;
#20743=CARTESIAN_POINT ( 'NONE',  ( -13.45431060380794541, 90.84076481352336430, 7.653071044410319601 ) ) ;
#20745=EDGE_LOOP ( 'NONE', ( #76134, #73033, #91440, #47676 ) ) ;
#20746=DIRECTION ( 'NONE',  ( 0.000000000000000000, -0.000000000000000000, 1.000000000000000000 ) ) ;
#20757=DIRECTION ( 'NONE',  ( -0.000000000000000000, -0.000000000000000000, 1.000000000000000000 ) ) ;
#20761=CARTESIAN_POINT ( 'NONE',  ( 4.656498301622464808, -8.256471156977859494, 3.749999999999998668 ) ) ;
#20768=EDGE_LOOP ( 'NONE', ( #3128, #66247, #61347, #45636 ) ) ;
#20771=CARTESIAN_POINT ( 'NONE',  ( -4.000000000000000000, 37.00000000000000000, 3.750000000000000000 ) ) ;
#20772=CARTESIAN_POINT ( 'NONE',  ( -12.24686443627858878, 90.44926614966340139, -7.163467944141197918 ) ) ;
#20773=FILL_AREA_STYLE ('',( #4789 ) ) ;
#20779=DIRECTION ( 'NONE',  ( -2.107602052970794797E-16, 1.000000000000000000, 0.000000000000000000 ) ) ;
#20787=SURFACE_SIDE_STYLE ('',( #49301 ) ) ;
#20796=ADVANCED_FACE ( 'NONE', ( #41087 ), #70374, .T. ) ;
#20806=EDGE_CURVE ( 'NONE', #87437, #11855, #16050, .T. ) ;
#20822=DIRECTION ( 'NONE',  ( -0.000000000000000000, -0.000000000000000000, -1.000000000000000000 ) ) ;
#20828=ORIENTED_EDGE ( 'NONE', *, *, #28948, .F. ) ;
#20837=CONICAL_SURFACE ( 'NONE', #30383, 1.249999999999987121, 1.029744258676654312 ) ;
#20842=DIRECTION ( 'NONE',  ( 1.000000000000000000, 3.945256819650108695E-12, 0.000000000000000000 ) ) ;
#20854=DIRECTION ( 'NONE',  ( 0.000000000000000000, -1.000000000000000000, 0.000000000000000000 ) ) ;
#20855=AXIS2_PLACEMENT_3D ( 'NONE', #89122, #81614, #81124 ) ;
#20861=DIRECTION ( 'NONE',  ( 0.000000000000000000, 0.000000000000000000, 1.000000000000000000 ) ) ;
#20867=EDGE_LOOP ( 'NONE', ( #86946, #42407, #9158, #64251 ) ) ;
#20870=CARTESIAN_POINT ( 'NONE',  ( -8.118176716543590743, 86.25458391402875691, -4.292297935673068388 ) ) ;
#20880=SURFACE_SIDE_STYLE ('',( #74858 ) ) ;
#20883=CARTESIAN_POINT ( 'NONE',  ( -8.099999999999999645, 83.99999999999994316, -2.900000000000000799 ) ) ;
#20892=CARTESIAN_POINT ( 'NONE',  ( -6.982525766850296023, -88.11956318484570261, -2.500000000000000888 ) ) ;
#20897=AXIS2_PLACEMENT_3D ( 'NONE', #406, #77337, #54341 ) ;
#20901=CYLINDRICAL_SURFACE ( 'NONE', #19727, 0.2500000000000002220 ) ;
#20902=CARTESIAN_POINT ( 'NONE',  ( -10.91025143199674829, -52.91559880499846003, -4.000000000000000888 ) ) ;
#20907=DIRECTION ( 'NONE',  ( 0.000000000000000000, 1.000000000000000000, 3.035766082959409260E-14 ) ) ;
#20913=LINE ( 'NONE', #3939, #3621 ) ;
#20942=( LENGTH_UNIT ( ) NAMED_UNIT ( * ) SI_UNIT ( .MILLI., .METRE. ) );
#20944=CARTESIAN_POINT ( 'NONE',  ( -8.000000000000000000, 79.82179676972448590, -4.250000000000000000 ) ) ;
#20955=EDGE_CURVE ( 'NONE', #43301, #63180, #52025, .T. ) ;
#20981=CARTESIAN_POINT ( 'NONE',  ( -5.809210876199123241, -36.07757871006187855, 2.750000000000000444 ) ) ;
#20984=VERTEX_POINT ( 'NONE', #52507 ) ;
#20986=CARTESIAN_POINT ( 'NONE',  ( 7.155629327958949126, -69.45263185074755086, 3.999999999999999112 ) ) ;
#20996=CARTESIAN_POINT ( 'NONE',  ( 6.732888861736110009, -58.30752899003807954, -2.750000000000000000 ) ) ;
#21004=EDGE_CURVE ( 'NONE', #72511, #57827, #4916, .T. ) ;
#21011=ORIENTED_EDGE ( 'NONE', *, *, #15294, .F. ) ;
#21019=DIRECTION ( 'NONE',  ( -1.000000000000000000, 0.000000000000000000, 0.000000000000000000 ) ) ;
#21028=FILL_AREA_STYLE ('',( #87543 ) ) ;
#21031=EDGE_CURVE ( 'NONE', #20454, #95449, #58524, .T. ) ;
#21054=CARTESIAN_POINT ( 'NONE',  ( 11.33948230079944253, -87.84096554735758389, -3.749999999999999556 ) ) ;
#21078=EDGE_CURVE ( 'NONE', #59804, #76742, #6036, .T. ) ;
#21081=VERTEX_POINT ( 'NONE', #58028 ) ;
#21086=ORIENTED_EDGE ( 'NONE', *, *, #38357, .F. ) ;
#21095=ORIENTED_EDGE ( 'NONE', *, *, #42772, .F. ) ;
#21099=LINE ( 'NONE', #81585, #50074 ) ;
#21104=CARTESIAN_POINT ( 'NONE',  ( 17.99999999999999645, 91.28723161455539525, -8.000000000000000000 ) ) ;
#21105=CARTESIAN_POINT ( 'NONE',  ( -7.121361074407936975, -73.24646532379340158, 3.749999999999999556 ) ) ;
#21121=EDGE_CURVE ( 'NONE', #83598, #26486, #73521, .T. ) ;
#21122=EDGE_CURVE ( 'NONE', #18240, #72111, #89558, .T. ) ;
#21129=FILL_AREA_STYLE_COLOUR ( '', #22600 ) ;
#21132=CARTESIAN_POINT ( 'NONE',  ( 15.00000000000000000, 77.07179676972447169, -6.500000000000000888 ) ) ;
#21144=EDGE_CURVE ( 'NONE', #65098, #58411, #10742, .T. ) ;
#21152=EDGE_CURVE ( 'NONE', #44437, #54112, #22473, .T. ) ;
#21167=ORIENTED_EDGE ( 'NONE', *, *, #26397, .T. ) ;
#21174=CARTESIAN_POINT ( 'NONE',  ( -11.26393249273843011, -93.42496533368144185, 3.750000000000000000 ) ) ;
#21184=AXIS2_PLACEMENT_3D ( 'NONE', #52358, #37375, #82859 ) ;
#21187=DIRECTION ( 'NONE',  ( -0.000000000000000000, -0.000000000000000000, 1.000000000000000000 ) ) ;
#21195=EDGE_CURVE ( 'NONE', #39466, #69849, #91500, .T. ) ;
#21204=ORIENTED_EDGE ( 'NONE', *, *, #98705, .F. ) ;
#21205=CIRCLE ( 'NONE', #62647, 3.000000000000002665 ) ;
#21211=DIRECTION ( 'NONE',  ( -0.9975640502598243087, 0.06975647374412452528, -0.000000000000000000 ) ) ;
#21213=DIRECTION ( 'NONE',  ( -0.000000000000000000, -0.000000000000000000, 1.000000000000000000 ) ) ;
#21222=CARTESIAN_POINT ( 'NONE',  ( 4.629999999999994564, 43.00000000000000711, 4.000000000000000000 ) ) ;
#21233=AXIS2_PLACEMENT_3D ( 'NONE', #47828, #46366, #23387 ) ;
#21238=EDGE_CURVE ( 'NONE', #82102, #2502, #54473, .T. ) ;
#21260=ORIENTED_EDGE ( 'NONE', *, *, #22376, .T. ) ;
#21265=( NAMED_UNIT ( * ) SI_UNIT ( $, .STERADIAN. ) SOLID_ANGLE_UNIT ( ) );
#21271=EDGE_CURVE ( 'NONE', #52968, #76742, #33643, .T. ) ;
#21272=CARTESIAN_POINT ( 'NONE',  ( 11.44533173448679619, -77.48526441101047624, -4.000000000000000000 ) ) ;
#21280=DIRECTION ( 'NONE',  ( 0.000000000000000000, 1.000000000000000000, 0.000000000000000000 ) ) ;
#21284=AXIS2_PLACEMENT_3D ( 'NONE', #69966, #45987, #91970 ) ;
#21300=SURFACE_STYLE_FILL_AREA ( #5804 ) ;
#21305=ORIENTED_EDGE ( 'NONE', *, *, #14272, .F. ) ;
#21315=STYLED_ITEM ( 'NONE', ( #62941 ), #96216 ) ;
#21325=MECHANICAL_DESIGN_GEOMETRIC_PRESENTATION_REPRESENTATION('',(#29301),#595);
#21334=VERTEX_POINT ( 'NONE', #23021 ) ;
#21348=SURFACE_STYLE_FILL_AREA ( #74326 ) ;
#21354=EDGE_CURVE ( 'NONE', #62017, #89406, #56023, .T. ) ;
#21359=EDGE_CURVE ( 'NONE', #15746, #2183, #60503, .T. ) ;
#21371=ORIENTED_EDGE ( 'NONE', *, *, #6894, .F. ) ;
#21372=( NAMED_UNIT ( * ) SI_UNIT ( $, .STERADIAN. ) SOLID_ANGLE_UNIT ( ) );
#21375=DIRECTION ( 'NONE',  ( -1.000000000000000000, 0.000000000000000000, 0.000000000000000000 ) ) ;
#21378=ORIENTED_EDGE ( 'NONE', *, *, #41239, .T. ) ;
#21390=ORIENTED_EDGE ( 'NONE', *, *, #90819, .F. ) ;
#21392=SURFACE_STYLE_FILL_AREA ( #90355 ) ;
#21393=EDGE_CURVE ( 'NONE', #35759, #59916, #75130, .T. ) ;
#21396=( LENGTH_UNIT ( ) NAMED_UNIT ( * ) SI_UNIT ( .MILLI., .METRE. ) );
#21400=DIRECTION ( 'NONE',  ( -0.000000000000000000, 1.000000000000000000, -0.000000000000000000 ) ) ;
#21404=DIRECTION ( 'NONE',  ( 0.000000000000000000, 0.000000000000000000, 1.000000000000000000 ) ) ;
#21407=B_SPLINE_CURVE_WITH_KNOTS ( 'NONE', 3,
 ( #32440, #989, #93441, #92939, #69468, #9451 ),
 .UNSPECIFIED., .F., .F.,
 ( 4, 2, 4 ),
 ( -1.099704249473512899E-05, 0.0008751816947074439641, 0.001761360431909623093 ),
 .UNSPECIFIED. ) ;
#21422=ORIENTED_EDGE ( 'NONE', *, *, #91077, .F. ) ;
#21427=VERTEX_POINT ( 'NONE', #72423 ) ;
#21430=CARTESIAN_POINT ( 'NONE',  ( 4.645844135293939914, -0.8374644621422210333, 4.000000000000000000 ) ) ;
#21431=CARTESIAN_POINT ( 'NONE',  ( 0.000000000000000000, 0.000000000000000000, 8.000000000000000000 ) ) ;
#21433=DIRECTION ( 'NONE',  ( 1.000000000000000000, 0.000000000000000000, 0.000000000000000000 ) ) ;
#21441=ORIENTED_EDGE ( 'NONE', *, *, #74292, .F. ) ;
#21446=SURFACE_STYLE_FILL_AREA ( #8292 ) ;
#21454=VECTOR ( 'NONE', #48016, 1000.000000000000000 ) ;
#21462=ORIENTED_EDGE ( 'NONE', *, *, #64553, .F. ) ;
#21467=DIRECTION ( 'NONE',  ( 0.000000000000000000, 0.000000000000000000, 1.000000000000000000 ) ) ;
#21470=CARTESIAN_POINT ( 'NONE',  ( 9.209315896035914051, -9.300848983899108191, 3.750000000000000000 ) ) ;
#21472=VERTEX_POINT ( 'NONE', #86471 ) ;
#21480=UNCERTAINTY_MEASURE_WITH_UNIT (LENGTH_MEASURE( 1.000000000000000082E-05 ), #65012, 'distance_accuracy_value', 'NONE');
#21486=CARTESIAN_POINT ( 'NONE',  ( -13.76191411541410048, 90.94479608829072959, -7.905863191225801501 ) ) ;
#21489=ORIENTED_EDGE ( 'NONE', *, *, #77434, .T. ) ;
#21525=FACE_OUTER_BOUND ( 'NONE', #74586, .T. ) ;
#21532=CARTESIAN_POINT ( 'NONE',  ( 17.88828545106793655, 91.03678680451055527, 8.000000000000001776 ) ) ;
#21534=ORIENTED_EDGE ( 'NONE', *, *, #53716, .T. ) ;
#21545=( LENGTH_UNIT ( ) NAMED_UNIT ( * ) SI_UNIT ( .MILLI., .METRE. ) );
#21557=VECTOR ( 'NONE', #39348, 1000.000000000000000 ) ;
#21560=CARTESIAN_POINT ( 'NONE',  ( -12.79762580179198039, 90.64749249312866652, -7.346077433012456304 ) ) ;
#21570=ORIENTED_EDGE ( 'NONE', *, *, #25455, .T. ) ;
#21594=CARTESIAN_POINT ( 'NONE',  ( -3.999999999999999112, 78.07179676972445748, -4.250000000000000000 ) ) ;
#21599=ORIENTED_EDGE ( 'NONE', *, *, #87049, .T. ) ;
#21618=FACE_OUTER_BOUND ( 'NONE', #83419, .T. ) ;
#21620=( LENGTH_UNIT ( ) NAMED_UNIT ( * ) SI_UNIT ( .MILLI., .METRE. ) );
#21631=DIRECTION ( 'NONE',  ( -0.5905099943842175847, -0.8070303256584298035, 0.000000000000000000 ) ) ;
#21640=STYLED_ITEM ( 'NONE', ( #86298 ), #53296 ) ;
#21641=EDGE_CURVE ( 'NONE', #38304, #23275, #24122, .T. ) ;
#21646=CARTESIAN_POINT ( 'NONE',  ( 8.979999999999991545, 0.000000000000000000, 3.000000000000000000 ) ) ;
#21648=AXIS2_PLACEMENT_3D ( 'NONE', #73267, #35265, #65762 ) ;
#21654=EDGE_CURVE ( 'NONE', #11855, #60629, #64912, .T. ) ;
#21664=AXIS2_PLACEMENT_3D ( 'NONE', #81051, #11571, #65044 ) ;
#21668=ORIENTED_EDGE ( 'NONE', *, *, #93405, .F. ) ;
#21669=( NAMED_UNIT ( * ) PLANE_ANGLE_UNIT ( ) SI_UNIT ( $, .RADIAN. ) );
#21676=( NAMED_UNIT ( * ) PLANE_ANGLE_UNIT ( ) SI_UNIT ( $, .RADIAN. ) );
#21680=CIRCLE ( 'NONE', #52002, 0.2499999999999980294 ) ;
#21686=ORIENTED_EDGE ( 'NONE', *, *, #78131, .F. ) ;
#21688=VERTEX_POINT ( 'NONE', #24992 ) ;
#21698=AXIS2_PLACEMENT_3D ( 'NONE', #43621, #65623, #49633 ) ;
#21701=EDGE_LOOP ( 'NONE', ( #24655, #72686, #91285, #51016 ) ) ;
#21704=ORIENTED_EDGE ( 'NONE', *, *, #41262, .F. ) ;
#21709=LINE ( 'NONE', #52682, #81849 ) ;
#21710=EDGE_CURVE ( 'NONE', #82533, #70499, #57636, .T. ) ;
#21711=CARTESIAN_POINT ( 'NONE',  ( -4.000000000000000000, 37.00000000000000000, 2.750000000000000000 ) ) ;
#21714=VECTOR ( 'NONE', #81243, 1000.000000000000000 ) ;
#21720=( NAMED_UNIT ( * ) PLANE_ANGLE_UNIT ( ) SI_UNIT ( $, .RADIAN. ) );
#21721=( NAMED_UNIT ( * ) SI_UNIT ( $, .STERADIAN. ) SOLID_ANGLE_UNIT ( ) );
#21724=ADVANCED_FACE ( 'NONE', ( #32870 ), #19113, .T. ) ;
#21726=ORIENTED_EDGE ( 'NONE', *, *, #57443, .F. ) ;
#21728=DIRECTION ( 'NONE',  ( -0.000000000000000000, -0.000000000000000000, -1.000000000000000000 ) ) ;
#21742=AXIS2_PLACEMENT_3D ( 'NONE', #38173, #44670, #83165 ) ;
#21754=CARTESIAN_POINT ( 'NONE',  ( 4.630000000000003446, 1.019547802438464545, 4.000000000000000000 ) ) ;
#21762=PRESENTATION_STYLE_ASSIGNMENT (( #59735 ) ) ;
#21772=SURFACE_STYLE_USAGE ( .BOTH. , #7757 ) ;
#21778=CARTESIAN_POINT ( 'NONE',  ( 10.88670032936942711, -94.01435490392699990, -4.000000000000000000 ) ) ;
#21793=CARTESIAN_POINT ( 'NONE',  ( -8.000000000000000000, 79.82179676972448590, 4.250000000000000000 ) ) ;
#21803=DIRECTION ( 'NONE',  ( 0.000000000000000000, -0.000000000000000000, -1.000000000000000000 ) ) ;
#21814=VECTOR ( 'NONE', #42766, 1000.000000000000114 ) ;
#21819=CIRCLE ( 'NONE', #82463, 1.249999999999987121 ) ;
#21832=CIRCLE ( 'NONE', #55370, 0.2499999999999997224 ) ;
#21833=ORIENTED_EDGE ( 'NONE', *, *, #64637, .T. ) ;
#21834=AXIS2_PLACEMENT_3D ( 'NONE', #32544, #31064, #61563 ) ;
#21836=DIRECTION ( 'NONE',  ( -0.000000000000000000, -0.000000000000000000, -1.000000000000000000 ) ) ;
#21840=EDGE_CURVE ( 'NONE', #45159, #17988, #83004, .T. ) ;
#21846=FILL_AREA_STYLE ('',( #14340 ) ) ;
#21860=CARTESIAN_POINT ( 'NONE',  ( 6.829574850505124139, -88.00372650098202598, -2.500000000000001776 ) ) ;
#21871=LINE ( 'NONE', #45340, #47823 ) ;
#21876=CARTESIAN_POINT ( 'NONE',  ( -3.250000000000000444, 1.019547802438465656, 2.500000000000000000 ) ) ;
#21885=CARTESIAN_POINT ( 'NONE',  ( -7.121341127240343738, -73.24353698637879972, -2.500000000000000000 ) ) ;
#21892=ORIENTED_EDGE ( 'NONE', *, *, #56016, .F. ) ;
#21894=LINE ( 'NONE', #55327, #82950 ) ;
#21911=TOROIDAL_SURFACE ( 'NONE', #64969, 0.5000000000000000000, 0.2500000000000000000 ) ;
#21930=ORIENTED_EDGE ( 'NONE', *, *, #45398, .T. ) ;
#21933=ADVANCED_FACE ( 'NONE', ( #41874 ), #79852, .T. ) ;
#21934=( NAMED_UNIT ( * ) PLANE_ANGLE_UNIT ( ) SI_UNIT ( $, .RADIAN. ) );
#21935=DIRECTION ( 'NONE',  ( 0.000000000000000000, 0.000000000000000000, -1.000000000000000000 ) ) ;
#21963=EDGE_CURVE ( 'NONE', #10040, #2203, #57831, .T. ) ;
#21979=MECHANICAL_DESIGN_GEOMETRIC_PRESENTATION_REPRESENTATION('',(#65045),#77841);
#21985=CARTESIAN_POINT ( 'NONE',  ( -8.223478179881292149, 85.80780507572754345, 3.936430718245549354 ) ) ;
#21991=CARTESIAN_POINT ( 'NONE',  ( -4.000000000000000000, 10.25000000000000000, -3.750000000000000000 ) ) ;
#22014=CIRCLE ( 'NONE', #77875, 0.2500000000000002220 ) ;
#22022=( LENGTH_UNIT ( ) NAMED_UNIT ( * ) SI_UNIT ( .MILLI., .METRE. ) );
#22023=ORIENTED_EDGE ( 'NONE', *, *, #22063, .F. ) ;
#22033=CARTESIAN_POINT ( 'NONE',  ( -6.732636091893171582, -88.11213685669366669, -2.750000000000000444 ) ) ;
#22049=CIRCLE ( 'NONE', #63499, 6.349999999999995204 ) ;
#22050=CARTESIAN_POINT ( 'NONE',  ( -6.607869636406716651, -50.96183896326274265, -3.750000000003224976 ) ) ;
#22051=COLOUR_RGB ( '', 0.09019608, 0.27058824, 0.51372549) ;
#22058=CARTESIAN_POINT ( 'NONE',  ( -8.004782461319722486, 84.51756810411900744, -3.749999999999998668 ) ) ;
#22063=EDGE_CURVE ( 'NONE', #54112, #93500, #5351, .T. ) ;
#22071=ORIENTED_EDGE ( 'NONE', *, *, #80768, .F. ) ;
#22083=ORIENTED_EDGE ( 'NONE', *, *, #22207, .T. ) ;
#22085=VERTEX_POINT ( 'NONE', #4853 ) ;
#22096=DIRECTION ( 'NONE',  ( 0.000000000000000000, 0.000000000000000000, 1.000000000000000000 ) ) ;
#22102=VERTEX_POINT ( 'NONE', #65822 ) ;
#22112=SURFACE_STYLE_USAGE ( .BOTH. , #30080 ) ;
#22120=CARTESIAN_POINT ( 'NONE',  ( -3.990799379706100325, -9.967613007074422882, -3.750000000000000000 ) ) ;
#22123=DIRECTION ( 'NONE',  ( -0.000000000000000000, 0.000000000000000000, 1.000000000000000000 ) ) ;
#22141=VERTEX_POINT ( 'NONE', #43324 ) ;
#22143=CARTESIAN_POINT ( 'NONE',  ( 12.30000000000000249, 99.99999999999998579, 8.000000000000000000 ) ) ;
#22165=CARTESIAN_POINT ( 'NONE',  ( -8.000000000000000000, -0.01653120532836994255, 3.750000000000000000 ) ) ;
#22173=STYLED_ITEM ( 'NONE', ( #50408 ), #14065 ) ;
#22176=EDGE_LOOP ( 'NONE', ( #79729, #27986, #41228, #56796 ) ) ;
#22178=ORIENTED_EDGE ( 'NONE', *, *, #55004, .T. ) ;
#22181=ORIENTED_EDGE ( 'NONE', *, *, #74263, .T. ) ;
#22187=CARTESIAN_POINT ( 'NONE',  ( 12.14357320772536575, 54.02013147999952736, 2.900000000000000355 ) ) ;
#22194=EDGE_LOOP ( 'NONE', ( #51470, #46718, #67561, #94648 ) ) ;
#22197=ORIENTED_EDGE ( 'NONE', *, *, #86392, .F. ) ;
#22207=EDGE_CURVE ( 'NONE', #91180, #92042, #55886, .T. ) ;
#22208=AXIS2_PLACEMENT_3D ( 'NONE', #41870, #49346, #33349 ) ;
#22209=DIRECTION ( 'NONE',  ( 0.000000000000000000, 0.000000000000000000, 1.000000000000000000 ) ) ;
#22213=DIRECTION ( 'NONE',  ( -1.000000000000000000, -0.000000000000000000, -0.000000000000000000 ) ) ;
#22217=DIRECTION ( 'NONE',  ( -1.000000000000000000, 0.000000000000000000, 0.000000000000000000 ) ) ;
#22219=LINE ( 'NONE', #93151, #91474 ) ;
#22228=CARTESIAN_POINT ( 'NONE',  ( -15.00000000000000000, 83.99999999999998579, 4.000000000000000000 ) ) ;
#22241=PRESENTATION_STYLE_ASSIGNMENT (( #250 ) ) ;
#22242=TOROIDAL_SURFACE ( 'NONE', #81245, 0.5000000000000000000, 0.2500000000000000000 ) ;
#22244=LINE ( 'NONE', #75224, #94215 ) ;
#22247=DIRECTION ( 'NONE',  ( 1.000000000000000000, -0.000000000000000000, -0.000000000000000000 ) ) ;
#22261=EDGE_CURVE ( 'NONE', #63379, #23275, #97340, .T. ) ;
#22269=ORIENTED_EDGE ( 'NONE', *, *, #80502, .F. ) ;
#22271=CARTESIAN_POINT ( 'NONE',  ( 10.72174155805500995, -40.27583460507576518, -3.749999999996413536 ) ) ;
#22278=( NAMED_UNIT ( * ) PLANE_ANGLE_UNIT ( ) SI_UNIT ( $, .RADIAN. ) );
#22281=FILL_AREA_STYLE ('',( #15280 ) ) ;
#22301=MECHANICAL_DESIGN_GEOMETRIC_PRESENTATION_REPRESENTATION('',(#89220),#55765);
#22302=DIRECTION ( 'NONE',  ( 1.000000000000000000, 0.000000000000000000, 0.000000000000000000 ) ) ;
#22313=EDGE_LOOP ( 'NONE', ( #7387, #79572, #13659, #8869 ) ) ;
#22317=DIRECTION ( 'NONE',  ( -1.000000000000000000, 0.000000000000000000, 0.000000000000000000 ) ) ;
#22338=CARTESIAN_POINT ( 'NONE',  ( 4.379999999999999893, 0.09082567841931840635, -3.750000000000000000 ) ) ;
#22341=SURFACE_SIDE_STYLE ('',( #7338 ) ) ;
#22346=AXIS2_PLACEMENT_3D ( 'NONE', #53185, #12717, #51213 ) ;
#22352=CARTESIAN_POINT ( 'NONE',  ( 4.380000001225145212, 0.09385850579744531297, -2.500000000000000000 ) ) ;
#22374=ORIENTED_EDGE ( 'NONE', *, *, #57735, .F. ) ;
#22376=EDGE_CURVE ( 'NONE', #32092, #37045, #4777, .T. ) ;
#22387=CARTESIAN_POINT ( 'NONE',  ( 3.969999999999999751, 10.25000000000000000, -2.750000000000000000 ) ) ;
#22393=CARTESIAN_POINT ( 'NONE',  ( 0.000000000000000000, -97.00000000000000000, -2.750000000000000000 ) ) ;
#22401=CIRCLE ( 'NONE', #89469, 0.2500000000000002220 ) ;
#22421=( NAMED_UNIT ( * ) SI_UNIT ( $, .STERADIAN. ) SOLID_ANGLE_UNIT ( ) );
#22426=CARTESIAN_POINT ( 'NONE',  ( 5.365144748710862110, -17.52568678401977920, 4.000000000000000000 ) ) ;
#22427=PRESENTATION_STYLE_ASSIGNMENT (( #90899 ) ) ;
#22428=FACE_OUTER_BOUND ( 'NONE', #6283, .T. ) ;
#22446=VECTOR ( 'NONE', #98234, 1000.000000000000000 ) ;
#22453=ORIENTED_EDGE ( 'NONE', *, *, #68187, .F. ) ;
#22458=CARTESIAN_POINT ( 'NONE',  ( -6.982525766850296023, -88.11956318484570261, 2.500000000000000888 ) ) ;
#22462=CARTESIAN_POINT ( 'NONE',  ( 4.906773990575424627, -8.256880746075378141, -4.000000000000000000 ) ) ;
#22464=ORIENTED_EDGE ( 'NONE', *, *, #59715, .T. ) ;
#22465=LINE ( 'NONE', #37969, #13449 ) ;
#22469=AXIS2_PLACEMENT_3D ( 'NONE', #33416, #33904, #88410 ) ;
#22470=UNCERTAINTY_MEASURE_WITH_UNIT (LENGTH_MEASURE( 1.000000000000000082E-05 ), #95002, 'distance_accuracy_value', 'NONE');
#22471=CARTESIAN_POINT ( 'NONE',  ( -10.03950393934412411, 88.95408272062866217, 5.473102654073078277 ) ) ;
#22473=CIRCLE ( 'NONE', #27227, 0.2500000000000000000 ) ;
#22477=CARTESIAN_POINT ( 'NONE',  ( -13.11254139118232231, 91.00000000000000000, -8.000000000000000000 ) ) ;
#22479=CARTESIAN_POINT ( 'NONE',  ( 5.510795456469524289, -25.29786701974074603, -2.750000000000000000 ) ) ;
#22494=ADVANCED_FACE ( 'NONE', ( #81808 ), #90981, .T. ) ;
#22496=EDGE_LOOP ( 'NONE', ( #32964, #24980, #57810, #90047 ) ) ;
#22517=DIRECTION ( 'NONE',  ( 1.000000000000000000, 0.000000000000000000, 0.000000000000000000 ) ) ;
#22541=CARTESIAN_POINT ( 'NONE',  ( -4.787219229845119273, -17.54708441700886468, -3.999999999999998224 ) ) ;
#22544=EDGE_LOOP ( 'NONE', ( #50191, #91783, #19622, #66090 ) ) ;
#22549=DIRECTION ( 'NONE',  ( 0.000000000000000000, 0.000000000000000000, -1.000000000000000000 ) ) ;
#22557=( GEOMETRIC_REPRESENTATION_CONTEXT ( 3 ) GLOBAL_UNCERTAINTY_ASSIGNED_CONTEXT ( ( #97417 ) ) GLOBAL_UNIT_ASSIGNED_CONTEXT ( ( #23265, #45756, #18088 ) ) REPRESENTATION_CONTEXT ( 'NONE', 'WORKASPACE' ) );
#22560=ORIENTED_EDGE ( 'NONE', *, *, #73061, .T. ) ;
#22561=ORIENTED_EDGE ( 'NONE', *, *, #73026, .F. ) ;
#22574=ORIENTED_EDGE ( 'NONE', *, *, #98608, .T. ) ;
#22576=ORIENTED_EDGE ( 'NONE', *, *, #52334, .T. ) ;
#22580=EDGE_CURVE ( 'NONE', #9323, #18983, #63849, .T. ) ;
#22583=DIRECTION ( 'NONE',  ( 0.08715574274765139351, 0.9961946980917461003, -0.000000000000000000 ) ) ;
#22585=CARTESIAN_POINT ( 'NONE',  ( 10.88666287821217082, -94.01511732729316861, 4.000000000000000000 ) ) ;
#22589=VERTEX_POINT ( 'NONE', #70778 ) ;
#22591=CARTESIAN_POINT ( 'NONE',  ( -4.250000000000000000, 36.75000000000000000, -3.750000000000000000 ) ) ;
#22600=COLOUR_RGB ( '', 0.09019608, 0.27058824, 0.51372549) ;
#22606=SURFACE_STYLE_FILL_AREA ( #123 ) ;
#22608=EDGE_CURVE ( 'NONE', #20984, #35180, #77267, .T. ) ;
#22610=VERTEX_POINT ( 'NONE', #55259 ) ;
#22618=DIRECTION ( 'NONE',  ( -0.000000000000000000, -0.000000000000000000, -1.000000000000000000 ) ) ;
#22625=FILL_AREA_STYLE ('',( #60101 ) ) ;
#22626=COLOUR_RGB ( '', 0.08235294, 0.09019608, 0.10196078) ;
#22643=ADVANCED_FACE ( 'NONE', ( #8778 ), #20837, .F. ) ;
#22651=STYLED_ITEM ( 'NONE', ( #49761 ), #39648 ) ;
#22657=AXIS2_PLACEMENT_3D ( 'NONE', #39847, #94804, #21280 ) ;
#22664=CARTESIAN_POINT ( 'NONE',  ( -10.54702889487960071, -44.61188042012589960, 4.000000000000000000 ) ) ;
#22673=ORIENTED_EDGE ( 'NONE', *, *, #1785, .T. ) ;
#22675=DIRECTION ( 'NONE',  ( 0.000000000000000000, -1.000000000000000000, 0.000000000000000000 ) ) ;
#22697=STYLED_ITEM ( 'NONE', ( #66601 ), #74641 ) ;
#22702=EDGE_CURVE ( 'NONE', #71617, #9146, #35158, .T. ) ;
#22744=DIRECTION ( 'NONE',  ( -0.02177529129954165754, -0.9997628902338895340, -2.778676860659971196E-13 ) ) ;
#22753=FILL_AREA_STYLE_COLOUR ( '', #59928 ) ;
#22754=DIRECTION ( 'NONE',  ( 0.08715574274765139351, 0.9961946980917461003, 0.000000000000000000 ) ) ;
#22762=CARTESIAN_POINT ( 'NONE',  ( 11.15633344613943123, -69.21805206906502406, -4.000000000000000000 ) ) ;
#22766=SURFACE_SIDE_STYLE ('',( #56086 ) ) ;
#22789=FACE_OUTER_BOUND ( 'NONE', #51953, .T. ) ;
#22792=CIRCLE ( 'NONE', #69099, 0.5000000000000004441 ) ;
#22806=DIRECTION ( 'NONE',  ( 0.000000000000000000, 0.000000000000000000, 1.000000000000000000 ) ) ;
#22823=AXIS2_PLACEMENT_3D ( 'NONE', #36723, #30674, #68211 ) ;
#22832=AXIS2_PLACEMENT_3D ( 'NONE', #35762, #35262, #66757 ) ;
#22834=FACE_OUTER_BOUND ( 'NONE', #39284, .T. ) ;
#22842=ORIENTED_EDGE ( 'NONE', *, *, #79791, .T. ) ;
#22846=CARTESIAN_POINT ( 'NONE',  ( 6.933985542754713904, -73.15302115696529484, -2.499999999998392397 ) ) ;
#22854=VECTOR ( 'NONE', #89429, 1000.000000000000000 ) ;
#22856=CYLINDRICAL_SURFACE ( 'NONE', #79802, 3.000000000000002665 ) ;
#22862=AXIS2_PLACEMENT_3D ( 'NONE', #1978, #16969, #23498 ) ;
#22864=CARTESIAN_POINT ( 'NONE',  ( -18.89999999999999147, 99.99999999999998579, -7.750000000000000000 ) ) ;
#22865=CARTESIAN_POINT ( 'NONE',  ( -11.05192081855196662, -57.06859629173521853, -4.000000000000000000 ) ) ;
#22870=ORIENTED_EDGE ( 'NONE', *, *, #8291, .F. ) ;
#22882=CARTESIAN_POINT ( 'NONE',  ( -15.00000000000004974, 91.00000000000000000, 4.000000000000000000 ) ) ;
#22883=CARTESIAN_POINT ( 'NONE',  ( -7.858204384948651366, -3.138042374739517193, -4.000000000000000000 ) ) ;
#22888=DIRECTION ( 'NONE',  ( 0.06975647374412534407, 0.9975640502598241977, -0.000000000000000000 ) ) ;
#22896=ADVANCED_FACE ( 'NONE', ( #72707 ), #11256, .T. ) ;
#22901=CARTESIAN_POINT ( 'NONE',  ( 8.879999999999999005, 20.99999999999999645, 1.249999999999987121 ) ) ;
#22902=AXIS2_PLACEMENT_3D ( 'NONE', #57113, #11618, #79133 ) ;
#22910=( GEOMETRIC_REPRESENTATION_CONTEXT ( 3 ) GLOBAL_UNCERTAINTY_ASSIGNED_CONTEXT ( ( #21480 ) ) GLOBAL_UNIT_ASSIGNED_CONTEXT ( ( #65012, #57036, #20528 ) ) REPRESENTATION_CONTEXT ( 'NONE', 'WORKASPACE' ) );
#22922=CARTESIAN_POINT ( 'NONE',  ( 4.823529266124356063, -6.402884419280910677, 4.000000000000000000 ) ) ;
#22929=CARTESIAN_POINT ( 'NONE',  ( -3.750000000000001776, 0.08806741915675847521, -4.000000000000000000 ) ) ;
#22946=EDGE_CURVE ( 'NONE', #89322, #86711, #18753, .T. ) ;
#22948=ADVANCED_FACE ( 'NONE', ( #34713 ), #95728, .T. ) ;
#22969=MECHANICAL_DESIGN_GEOMETRIC_PRESENTATION_REPRESENTATION('',(#96403),#94812);
#22972=CARTESIAN_POINT ( 'NONE',  ( -13.38735934609733036, 90.81479509783585513, 7.611013694203884405 ) ) ;
#22997=DIRECTION ( 'NONE',  ( -0.000000000000000000, -0.000000000000000000, 1.000000000000000000 ) ) ;
#23021=CARTESIAN_POINT ( 'NONE',  ( 4.629999999999991900, 76.07179676972444327, 4.000000000000000000 ) ) ;
#23043=VECTOR ( 'NONE', #86889, 1000.000000000000000 ) ;
#23049=DIRECTION ( 'NONE',  ( 0.000000000000000000, 1.000000000000000000, 0.000000000000000000 ) ) ;
#23064=EDGE_CURVE ( 'NONE', #70379, #7185, #94237, .T. ) ;
#23068=EDGE_CURVE ( 'NONE', #1670, #98319, #43700, .T. ) ;
#23081=AXIS2_PLACEMENT_3D ( 'NONE', #77846, #9355, #31357 ) ;
#23087=CARTESIAN_POINT ( 'NONE',  ( 4.380000000000002558, 1.019547802438462547, -3.750000000000000000 ) ) ;
#23088=FILL_AREA_STYLE ('',( #109 ) ) ;
#23092=CARTESIAN_POINT ( 'NONE',  ( 3.969999999999999751, 36.75000000000000000, 2.750000000000000000 ) ) ;
#23096=ORIENTED_EDGE ( 'NONE', *, *, #46328, .T. ) ;
#23106=ORIENTED_EDGE ( 'NONE', *, *, #56544, .T. ) ;
#23115=MECHANICAL_DESIGN_GEOMETRIC_PRESENTATION_REPRESENTATION('',(#66187),#90104);
#23121=CIRCLE ( 'NONE', #19879, 2.899999999999999911 ) ;
#23130=UNCERTAINTY_MEASURE_WITH_UNIT (LENGTH_MEASURE( 1.000000000000000082E-05 ), #20942, 'distance_accuracy_value', 'NONE');
#23145=SURFACE_SIDE_STYLE ('',( #40105 ) ) ;
#23147=( GEOMETRIC_REPRESENTATION_CONTEXT ( 3 ) GLOBAL_UNCERTAINTY_ASSIGNED_CONTEXT ( ( #94316 ) ) GLOBAL_UNIT_ASSIGNED_CONTEXT ( ( #69164, #70148, #31139 ) ) REPRESENTATION_CONTEXT ( 'NONE', 'WORKASPACE' ) );
#23158=CARTESIAN_POINT ( 'NONE',  ( -11.62541523590571657, -75.76371818141868175, 3.750000000000000000 ) ) ;
#23179=DIRECTION ( 'NONE',  ( 1.049065152435176504E-16, -1.000000000000000000, 0.000000000000000000 ) ) ;
#23194=CARTESIAN_POINT ( 'NONE',  ( -5.780262629516634831, -39.80185923444031459, 2.499999999999999556 ) ) ;
#23208=DIRECTION ( 'NONE',  ( -1.000000000000000000, 0.000000000000000000, 0.000000000000000000 ) ) ;
#23224=AXIS2_PLACEMENT_3D ( 'NONE', #1739, #48186, #70714 ) ;
#23233=( NAMED_UNIT ( * ) PLANE_ANGLE_UNIT ( ) SI_UNIT ( $, .RADIAN. ) );
#23235=LINE ( 'NONE', #59727, #74333 ) ;
#23243=PLANE ( 'NONE',  #45260 ) ;
#23255=FILL_AREA_STYLE ('',( #22753 ) ) ;
#23256=PLANE ( 'NONE',  #34389 ) ;
#23262=CARTESIAN_POINT ( 'NONE',  ( 10.34945593949844600, -32.01313548011462018, -4.000000000000000000 ) ) ;
#23265=( LENGTH_UNIT ( ) NAMED_UNIT ( * ) SI_UNIT ( .MILLI., .METRE. ) );
#23273=UNCERTAINTY_MEASURE_WITH_UNIT (LENGTH_MEASURE( 1.000000000000000082E-05 ), #6774, 'distance_accuracy_value', 'NONE');
#23275=VERTEX_POINT ( 'NONE', #59190 ) ;
#23278=DIRECTION ( 'NONE',  ( 0.000000000000000000, -0.000000000000000000, -1.000000000000000000 ) ) ;
#23290=SURFACE_SIDE_STYLE ('',( #7296 ) ) ;
#23300=LINE ( 'NONE', #68302, #34550 ) ;
#23301=ORIENTED_EDGE ( 'NONE', *, *, #15078, .T. ) ;
#23305=ADVANCED_FACE ( 'NONE', ( #68196 ), #98717, .F. ) ;
#23316=AXIS2_PLACEMENT_3D ( 'NONE', #87333, #11335, #41854 ) ;
#23332=PRESENTATION_STYLE_ASSIGNMENT (( #82820 ) ) ;
#23333=CARTESIAN_POINT ( 'NONE',  ( -3.521970974752482331, -0.8418515890118015710, -2.749999999999999556 ) ) ;
#23342=CARTESIAN_POINT ( 'NONE',  ( 6.324684870375198109, -50.88968658555813818, -2.499999999999999112 ) ) ;
#23345=CARTESIAN_POINT ( 'NONE',  ( 6.574847571011208203, -50.89175608700130482, 2.750000000000000444 ) ) ;
#23359=CARTESIAN_POINT ( 'NONE',  ( -9.823941624412537266, -32.16601312909467225, -4.000000000000000000 ) ) ;
#23362=FILL_AREA_STYLE_COLOUR ( '', #44816 ) ;
#23366=CARTESIAN_POINT ( 'NONE',  ( 4.219999999999999751, 10.00000000000000000, 3.750000000000000000 ) ) ;
#23374=( NAMED_UNIT ( * ) SI_UNIT ( $, .STERADIAN. ) SOLID_ANGLE_UNIT ( ) );
#23382=CARTESIAN_POINT ( 'NONE',  ( 3.969999999999999751, 10.25000000000000000, 4.000000000000000000 ) ) ;
#23387=DIRECTION ( 'NONE',  ( 0.000000000000000000, 0.000000000000000000, -1.000000000000000000 ) ) ;
#23398=CIRCLE ( 'NONE', #29783, 0.2500000000000002220 ) ;
#23411=AXIS2_PLACEMENT_3D ( 'NONE', #85680, #26159, #56654 ) ;
#23414=COLOUR_RGB ( '', 0.31764706, 0.68627451, 0.89019608) ;
#23417=AXIS2_PLACEMENT_3D ( 'NONE', #85561, #17072, #47555 ) ;
#23418=ADVANCED_FACE ( 'NONE', ( #66197 ), #96729, .F. ) ;
#23419=( NAMED_UNIT ( * ) PLANE_ANGLE_UNIT ( ) SI_UNIT ( $, .RADIAN. ) );
#23442=VECTOR ( 'NONE', #75027, 1000.000000000000000 ) ;
#23444=ORIENTED_EDGE ( 'NONE', *, *, #18847, .F. ) ;
#23468=DIRECTION ( 'NONE',  ( 0.06975647374412567714, 0.9975640502598243087, 0.000000000000000000 ) ) ;
#23470=EDGE_CURVE ( 'NONE', #93321, #14585, #6406, .T. ) ;
#23475=CARTESIAN_POINT ( 'NONE',  ( 4.722628015970558479, -9.822377395415374579, -3.750000000000000888 ) ) ;
#23476=CARTESIAN_POINT ( 'NONE',  ( 5.678900477199343655, -28.62996443930155266, 2.750000000000000000 ) ) ;
#23479=VERTEX_POINT ( 'NONE', #39672 ) ;
#23497=CARTESIAN_POINT ( 'NONE',  ( 4.441537491530695547, -2.700695904843435802, -4.000000000000000000 ) ) ;
#23498=DIRECTION ( 'NONE',  ( 1.000000000000000000, 0.000000000000000000, 0.000000000000000000 ) ) ;
#23521=ORIENTED_EDGE ( 'NONE', *, *, #78131, .T. ) ;
#23529=DIRECTION ( 'NONE',  ( -1.000000000000000000, 0.000000000000000000, 0.000000000000000000 ) ) ;
#23534=VERTEX_POINT ( 'NONE', #91675 ) ;
#23541=CARTESIAN_POINT ( 'NONE',  ( -18.00000000000000355, 75.73428692542562146, 2.900000000000000355 ) ) ;
#23547=CYLINDRICAL_SURFACE ( 'NONE', #18896, 1.249999999999987121 ) ;
#23549=EDGE_CURVE ( 'NONE', #39290, #61288, #10898, .T. ) ;
#23555=ORIENTED_EDGE ( 'NONE', *, *, #69909, .T. ) ;
#23563=CIRCLE ( 'NONE', #82624, 3.690000000000000391 ) ;
#23565=ORIENTED_EDGE ( 'NONE', *, *, #96580, .T. ) ;
#23570=EDGE_LOOP ( 'NONE', ( #10616, #97753, #81261 ) ) ;
#23577=ADVANCED_FACE ( 'NONE', ( #35465 ), #39966, .T. ) ;
#23585=( GEOMETRIC_REPRESENTATION_CONTEXT ( 3 ) GLOBAL_UNCERTAINTY_ASSIGNED_CONTEXT ( ( #3458 ) ) GLOBAL_UNIT_ASSIGNED_CONTEXT ( ( #32392, #95873, #41412 ) ) REPRESENTATION_CONTEXT ( 'NONE', 'WORKASPACE' ) );
#23593=CARTESIAN_POINT ( 'NONE',  ( 0.000000000000000000, -97.00000000000000000, 4.000000000000000000 ) ) ;
#23594=VERTEX_POINT ( 'NONE', #58960 ) ;
#23599=( LENGTH_UNIT ( ) NAMED_UNIT ( * ) SI_UNIT ( .MILLI., .METRE. ) );
#23603=ORIENTED_EDGE ( 'NONE', *, *, #92151, .T. ) ;
#23611=PLANE ( 'NONE',  #33607 ) ;
#23620=SURFACE_SIDE_STYLE ('',( #3080 ) ) ;
#23626=FILL_AREA_STYLE_COLOUR ( '', #47998 ) ;
#23632=EDGE_CURVE ( 'NONE', #27600, #6181, #59143, .T. ) ;
#23657=CARTESIAN_POINT ( 'NONE',  ( -10.07339213347369444, -32.14942050451527678, 4.000000000000000000 ) ) ;
#23665=EDGE_CURVE ( 'NONE', #78252, #72885, #9632, .T. ) ;
#23677=CARTESIAN_POINT ( 'NONE',  ( 4.629999999999999893, 4.857171655774867594E-16, -4.000000000000000000 ) ) ;
#23684=EDGE_LOOP ( 'NONE', ( #21599, #66305, #64836, #54068 ) ) ;
#23690=CARTESIAN_POINT ( 'NONE',  ( -4.818654718866499209, -24.96058166501294906, 2.499999999999999112 ) ) ;
#23695=AXIS2_PLACEMENT_3D ( 'NONE', #97577, #29038, #53025 ) ;
#23698=LINE ( 'NONE', #54158, #74513 ) ;
#23700=CARTESIAN_POINT ( 'NONE',  ( -18.89999999999999147, 91.25000000000000000, -8.000000000000000000 ) ) ;
#23702=FILL_AREA_STYLE_COLOUR ( '', #56928 ) ;
#23705=( NAMED_UNIT ( * ) PLANE_ANGLE_UNIT ( ) SI_UNIT ( $, .RADIAN. ) );
#23706=LINE ( 'NONE', #33133, #34716 ) ;
#23709=CARTESIAN_POINT ( 'NONE',  ( 15.00000000000000000, 77.07179676972447169, 6.500000000000000888 ) ) ;
#23721=CARTESIAN_POINT ( 'NONE',  ( 6.905552584539410788, -69.44516986207491982, -2.750000000000000444 ) ) ;
#23722=ORIENTED_EDGE ( 'NONE', *, *, #54271, .T. ) ;
#23731=DIRECTION ( 'NONE',  ( -1.000000000000000000, 0.000000000000000000, 0.000000000000000000 ) ) ;
#23738=SURFACE_SIDE_STYLE ('',( #7245 ) ) ;
#23750=CARTESIAN_POINT ( 'NONE',  ( 8.879999999999991900, 27.04366094290857347, 3.000000000000000000 ) ) ;
#23757=DIRECTION ( 'NONE',  ( -4.205390244792255888E-16, 1.000000000000000000, 8.410780489584511775E-16 ) ) ;
#23771=CARTESIAN_POINT ( 'NONE',  ( 4.600000000000003197, 98.49999999999998579, -8.525133428036873795 ) ) ;
#23772=( NAMED_UNIT ( * ) PLANE_ANGLE_UNIT ( ) SI_UNIT ( $, .RADIAN. ) );
#23781=CARTESIAN_POINT ( 'NONE',  ( 18.00000000000000000, 78.80384757729336798, 4.000000000000000000 ) ) ;
#23785=CARTESIAN_POINT ( 'NONE',  ( -6.607869636366940469, -50.96183896326462559, 4.000000000003224088 ) ) ;
#23788=LINE ( 'NONE', #54253, #57116 ) ;
#23810=ORIENTED_EDGE ( 'NONE', *, *, #25889, .T. ) ;
#23811=DIRECTION ( 'NONE',  ( 2.107602052970794797E-16, -1.000000000000000000, 0.000000000000000000 ) ) ;
#23829=FILL_AREA_STYLE ('',( #54292 ) ) ;
#23838=FILL_AREA_STYLE ('',( #92801 ) ) ;
#23840=DIRECTION ( 'NONE',  ( 1.000000000000000000, 0.000000000000000000, 0.000000000000000000 ) ) ;
#23847=CARTESIAN_POINT ( 'NONE',  ( 17.99999999999999645, 78.06028276952159217, -3.869891141068608320 ) ) ;
#23850=DIRECTION ( 'NONE',  ( -1.000000000000000000, 0.000000000000000000, -0.000000000000000000 ) ) ;
#23865=ORIENTED_EDGE ( 'NONE', *, *, #16980, .T. ) ;
#23870=CARTESIAN_POINT ( 'NONE',  ( -7.750000000000000000, 1.019547802438458550, -4.000000000000000000 ) ) ;
#23875=DIRECTION ( 'NONE',  ( 0.000000000000000000, 0.000000000000000000, -1.000000000000000000 ) ) ;
#23877=CARTESIAN_POINT ( 'NONE',  ( -18.00000000000000355, 75.73428692542562146, -3.000000000000000000 ) ) ;
#23900=ORIENTED_EDGE ( 'NONE', *, *, #30772, .T. ) ;
#23905=CARTESIAN_POINT ( 'NONE',  ( 6.905642986259637794, -69.45547628558860254, 3.750000000000000000 ) ) ;
#23918=DIRECTION ( 'NONE',  ( -1.000000000000000000, 0.000000000000000000, 0.000000000000000000 ) ) ;
#23931=EDGE_CURVE ( 'NONE', #40303, #5283, #30297, .T. ) ;
#23943=CARTESIAN_POINT ( 'NONE',  ( -8.000000000000000000, 80.32179676972448590, -4.250000000000000000 ) ) ;
#23950=CARTESIAN_POINT ( 'NONE',  ( 9.879999999999991900, 20.99999999999999645, -1.249999999999987121 ) ) ;
#23956=CARTESIAN_POINT ( 'NONE',  ( 4.441081520791478887, -2.684960557648791823, 2.750000000000000000 ) ) ;
#23959=LINE ( 'NONE', #79286, #27527 ) ;
#23960=DIRECTION ( 'NONE',  ( -2.569960705150826877E-16, 1.000000000000000000, 0.000000000000000000 ) ) ;
#23977=CARTESIAN_POINT ( 'NONE',  ( 8.979999999999991545, 27.03929484861773958, 3.000000000000000000 ) ) ;
#23979=CARTESIAN_POINT ( 'NONE',  ( -6.000000000000009770, 40.99999999999999289, -6.500000000000000888 ) ) ;
#24002=ORIENTED_EDGE ( 'NONE', *, *, #35382, .T. ) ;
#24003=DIRECTION ( 'NONE',  ( 1.000000000000000000, -0.000000000000000000, 0.000000000000000000 ) ) ;
#24049=AXIS2_PLACEMENT_3D ( 'NONE', #5423, #35893, #14898 ) ;
#24062=ORIENTED_EDGE ( 'NONE', *, *, #85350, .F. ) ;
#24067=( LENGTH_UNIT ( ) NAMED_UNIT ( * ) SI_UNIT ( .MILLI., .METRE. ) );
#24075=SURFACE_STYLE_FILL_AREA ( #30561 ) ;
#24081=CARTESIAN_POINT ( 'NONE',  ( -16.60833333333333073, 99.74999999999998579, 8.000000000000000000 ) ) ;
#24083=DIRECTION ( 'NONE',  ( 0.000000000000000000, 0.000000000000000000, 1.000000000000000000 ) ) ;
#24084=VECTOR ( 'NONE', #6716, 1000.000000000000000 ) ;
#24096=LINE ( 'NONE', #25089, #67792 ) ;
#24104=CARTESIAN_POINT ( 'NONE',  ( -7.750000000000000000, 0.000000000000000000, -3.750000000000000000 ) ) ;
#24107=CIRCLE ( 'NONE', #84773, 0.7500000000000006661 ) ;
#24115=COLOUR_RGB ( '', 0.31764706, 0.68627451, 0.89019608) ;
#24117=ORIENTED_EDGE ( 'NONE', *, *, #36990, .F. ) ;
#24120=DIRECTION ( 'NONE',  ( 0.000000000000000000, 0.000000000000000000, -1.000000000000000000 ) ) ;
#24122=CIRCLE ( 'NONE', #75198, 2.999999999999997335 ) ;
#24130=UNCERTAINTY_MEASURE_WITH_UNIT (LENGTH_MEASURE( 1.000000000000000082E-05 ), #91066, 'distance_accuracy_value', 'NONE');
#24132=ORIENTED_EDGE ( 'NONE', *, *, #60401, .T. ) ;
#24138=CARTESIAN_POINT ( 'NONE',  ( -8.028887233259784040, -1.053223610215041184, 3.750000000000000000 ) ) ;
#24147=FACE_OUTER_BOUND ( 'NONE', #5234, .T. ) ;
#24148=EDGE_LOOP ( 'NONE', ( #22464, #70646, #41249 ) ) ;
#24149=TOROIDAL_SURFACE ( 'NONE', #1819, 0.5000000000000000000, 0.2500000000000000000 ) ;
#24156=AXIS2_PLACEMENT_3D ( 'NONE', #97887, #13873, #88880 ) ;
#24166=FACE_OUTER_BOUND ( 'NONE', #14891, .T. ) ;
#24177=ORIENTED_EDGE ( 'NONE', *, *, #94487, .F. ) ;
#24178=CARTESIAN_POINT ( 'NONE',  ( -3.335599319945092844, -2.700684445899034447, 2.500000000000000888 ) ) ;
#24180=CARTESIAN_POINT ( 'NONE',  ( 8.862917521832709866, -7.247543382048746707, 4.000000000000000000 ) ) ;
#24184=( GEOMETRIC_REPRESENTATION_CONTEXT ( 3 ) GLOBAL_UNCERTAINTY_ASSIGNED_CONTEXT ( ( #60375 ) ) GLOBAL_UNIT_ASSIGNED_CONTEXT ( ( #15029, #67524, #37528 ) ) REPRESENTATION_CONTEXT ( 'NONE', 'WORKASPACE' ) );
#24185=CARTESIAN_POINT ( 'NONE',  ( 4.879999999999991900, 76.07179676972444327, -6.500000000000000888 ) ) ;
#24186=CARTESIAN_POINT ( 'NONE',  ( 4.630000000000003446, 1.019547802438464545, 3.750000000000000000 ) ) ;
#24193=AXIS2_PLACEMENT_3D ( 'NONE', #18103, #26092, #56588 ) ;
#24213=DIRECTION ( 'NONE',  ( -1.000000000000000000, 1.761140584748027129E-15, 0.000000000000000000 ) ) ;
#24234=UNCERTAINTY_MEASURE_WITH_UNIT (LENGTH_MEASURE( 1.000000000000000082E-05 ), #60767, 'distance_accuracy_value', 'NONE');
#24240=CARTESIAN_POINT ( 'NONE',  ( 8.705944879585906904, -3.115743166039381951, -4.000000000000000000 ) ) ;
#24241=CARTESIAN_POINT ( 'NONE',  ( -9.000000000000000000, 75.76920769491746910, 2.900000000000000355 ) ) ;
#24251=EDGE_CURVE ( 'NONE', #88687, #44437, #6756, .T. ) ;
#24254=ORIENTED_EDGE ( 'NONE', *, *, #76203, .F. ) ;
#24255=AXIS2_PLACEMENT_3D ( 'NONE', #14341, #44813, #45320 ) ;
#24256=ORIENTED_EDGE ( 'NONE', *, *, #27789, .F. ) ;
#24267=CARTESIAN_POINT ( 'NONE',  ( 17.90558034491757056, 78.11737700066547063, 4.059948642090509985 ) ) ;
#24270=CARTESIAN_POINT ( 'NONE',  ( -7.374934931933696092, -78.83424294380051833, 4.000000000000000888 ) ) ;
#24271=ORIENTED_EDGE ( 'NONE', *, *, #10327, .T. ) ;
#24276=ORIENTED_EDGE ( 'NONE', *, *, #4812, .F. ) ;
#24289=PRESENTATION_STYLE_ASSIGNMENT (( #37326 ) ) ;
#24293=DIRECTION ( 'NONE',  ( -0.000000000000000000, 0.000000000000000000, 1.000000000000000000 ) ) ;
#24296=ORIENTED_EDGE ( 'NONE', *, *, #17533, .T. ) ;
#24297=EDGE_CURVE ( 'NONE', #70269, #48471, #10768, .T. ) ;
#24304=DIRECTION ( 'NONE',  ( 1.000000000000000000, 0.000000000000000000, 0.000000000000000000 ) ) ;
#24318=( NAMED_UNIT ( * ) PLANE_ANGLE_UNIT ( ) SI_UNIT ( $, .RADIAN. ) );
#24332=EDGE_CURVE ( 'NONE', #2137, #55638, #81819, .T. ) ;
#24342=ADVANCED_FACE ( 'NONE', ( #89216 ), #95743, .F. ) ;
#24343=CARTESIAN_POINT ( 'NONE',  ( -8.107947183002034208, -3.126532598414448749, -4.000000000000000000 ) ) ;
#24358=EDGE_LOOP ( 'NONE', ( #65572, #40880, #31745, #69449 ) ) ;
#24359=DIRECTION ( 'NONE',  ( -1.000000000000000000, 0.000000000000000000, 0.000000000000000000 ) ) ;
#24366=DIRECTION ( 'NONE',  ( 1.000000000000000000, 0.000000000000000000, 0.000000000000000000 ) ) ;
#24377=FACE_OUTER_BOUND ( 'NONE', #98835, .T. ) ;
#24394=EDGE_LOOP ( 'NONE', ( #70260, #82942, #17749, #4602 ) ) ;
#24402=CIRCLE ( 'NONE', #32364, 0.2500000000000002220 ) ;
#24410=VECTOR ( 'NONE', #91346, 1000.000000000000000 ) ;
#24424=ORIENTED_EDGE ( 'NONE', *, *, #92675, .T. ) ;
#24430=CARTESIAN_POINT ( 'NONE',  ( -9.795238246328622722, -28.02849944208173127, 3.750000000000001332 ) ) ;
#24438=VECTOR ( 'NONE', #22213, 1000.000000000000000 ) ;
#24444=CARTESIAN_POINT ( 'NONE',  ( -13.80105244023572197, 90.89655890636302615, 7.750000000000543565 ) ) ;
#24451=CARTESIAN_POINT ( 'NONE',  ( 6.673414917871782315, -55.62670566514463388, -3.750000000000000888 ) ) ;
#24452=CARTESIAN_POINT ( 'NONE',  ( 6.757497259964397429, -58.30388498758440363, 2.500000000003219203 ) ) ;
#24454=VERTEX_POINT ( 'NONE', #88224 ) ;
#24461=STYLED_ITEM ( 'NONE', ( #32820 ), #66015 ) ;
#24464=VERTEX_POINT ( 'NONE', #11742 ) ;
#24472=VECTOR ( 'NONE', #89262, 1000.000000000000000 ) ;
#24473=FACE_OUTER_BOUND ( 'NONE', #76135, .T. ) ;
#24475=CIRCLE ( 'NONE', #85132, 0.2500000000000002220 ) ;
#24476=FACE_OUTER_BOUND ( 'NONE', #75742, .T. ) ;
#24513=CIRCLE ( 'NONE', #16512, 0.2500000000000002220 ) ;
#24514=EDGE_CURVE ( 'NONE', #77456, #25656, #96241, .T. ) ;
#24533=DIRECTION ( 'NONE',  ( 0.000000000000000000, -0.000000000000000000, -1.000000000000000000 ) ) ;
#24536=FACE_OUTER_BOUND ( 'NONE', #67092, .T. ) ;
#24548=AXIS2_PLACEMENT_3D ( 'NONE', #58090, #6098, #13594 ) ;
#24554=ORIENTED_EDGE ( 'NONE', *, *, #16542, .T. ) ;
#24562=ORIENTED_EDGE ( 'NONE', *, *, #37855, .T. ) ;
#24564=EDGE_LOOP ( 'NONE', ( #31463, #68136 ) ) ;
#24572=SURFACE_SIDE_STYLE ('',( #86047 ) ) ;
#24576=LINE ( 'NONE', #76071, #72199 ) ;
#24577=VERTEX_POINT ( 'NONE', #59202 ) ;
#24586=ORIENTED_EDGE ( 'NONE', *, *, #42772, .T. ) ;
#24592=CARTESIAN_POINT ( 'NONE',  ( 9.050000000000002487, 99.99999999999998579, -8.000000000000000000 ) ) ;
#24598=DIRECTION ( 'NONE',  ( 0.000000000000000000, -0.000000000000000000, 1.000000000000000000 ) ) ;
#24600=DIRECTION ( 'NONE',  ( -2.569960705150826877E-16, 1.000000000000000000, 0.000000000000000000 ) ) ;
#24606=VECTOR ( 'NONE', #94199, 1000.000000000000000 ) ;
#24610=DIRECTION ( 'NONE',  ( -0.000000000000000000, 0.000000000000000000, -1.000000000000000000 ) ) ;
#24614=CIRCLE ( 'NONE', #15063, 1.750000000000000666 ) ;
#24627=ORIENTED_EDGE ( 'NONE', *, *, #54530, .T. ) ;
#24632=DIRECTION ( 'NONE',  ( -0.000000000000000000, -0.000000000000000000, 1.000000000000000000 ) ) ;
#24641=DIRECTION ( 'NONE',  ( -1.000000000000000000, 0.000000000000000000, 0.000000000000000000 ) ) ;
#24642=FILL_AREA_STYLE_COLOUR ( '', #46083 ) ;
#24649=DIRECTION ( 'NONE',  ( 1.000000000000000000, 2.569960705150834273E-16, 0.000000000000000000 ) ) ;
#24655=ORIENTED_EDGE ( 'NONE', *, *, #7958, .T. ) ;
#24668=AXIS2_PLACEMENT_3D ( 'NONE', #47406, #79392, #32403 ) ;
#24670=DIRECTION ( 'NONE',  ( 0.000000000000000000, 0.000000000000000000, -1.000000000000000000 ) ) ;
#24684=CARTESIAN_POINT ( 'NONE',  ( 6.880000000000011440, 40.74999999999999289, 4.250000000000000000 ) ) ;
#24698=EDGE_CURVE ( 'NONE', #36015, #15178, #24402, .T. ) ;
#24716=ORIENTED_EDGE ( 'NONE', *, *, #96222, .T. ) ;
#24734=EDGE_CURVE ( 'NONE', #19346, #67870, #27581, .T. ) ;
#24737=ORIENTED_EDGE ( 'NONE', *, *, #95076, .T. ) ;
#24738=EDGE_LOOP ( 'NONE', ( #4412, #11525, #52571, #10358 ) ) ;
#24741=( NAMED_UNIT ( * ) SI_UNIT ( $, .STERADIAN. ) SOLID_ANGLE_UNIT ( ) );
#24751=AXIS2_PLACEMENT_3D ( 'NONE', #55736, #9736, #64674 ) ;
#24753=CARTESIAN_POINT ( 'NONE',  ( -18.89999999999999147, 99.74999999999998579, -7.750000000000000000 ) ) ;
#24754=CARTESIAN_POINT ( 'NONE',  ( 17.81748129626868504, 78.53842255729946942, 4.009548935143046222 ) ) ;
#24757=CARTESIAN_POINT ( 'NONE',  ( -7.371446924914479837, -73.25787537890647627, 4.000000000000000888 ) ) ;
#24763=EDGE_LOOP ( 'NONE', ( #29788, #38942 ) ) ;
#24768=VERTEX_POINT ( 'NONE', #14220 ) ;
#24771=CIRCLE ( 'NONE', #90187, 0.2500000000000002220 ) ;
#24777=EDGE_CURVE ( 'NONE', #89183, #89322, #78701, .T. ) ;
#24778=ORIENTED_EDGE ( 'NONE', *, *, #10327, .F. ) ;
#24784=CARTESIAN_POINT ( 'NONE',  ( -8.900000000000000355, 75.73428692542562146, -3.000000000000000000 ) ) ;
#24787=AXIS2_PLACEMENT_3D ( 'NONE', #40801, #93296, #2330 ) ;
#24798=FACE_OUTER_BOUND ( 'NONE', #37428, .T. ) ;
#24802=CIRCLE ( 'NONE', #19999, 0.2500000000000002220 ) ;
#24817=SURFACE_STYLE_USAGE ( .BOTH. , #84817 ) ;
#24823=FILL_AREA_STYLE_COLOUR ( '', #9572 ) ;
#24826=DIRECTION ( 'NONE',  ( 0.06975647374412512203, 0.9975640502598241977, 0.000000000000000000 ) ) ;
#24835=CARTESIAN_POINT ( 'NONE',  ( -8.211425130294045971, 85.75922772022539675, -4.168580035010579721 ) ) ;
#24844=DIRECTION ( 'NONE',  ( -2.569960705150826877E-16, 1.000000000000000000, 0.000000000000000000 ) ) ;
#24851=DIRECTION ( 'NONE',  ( -1.000000000000000000, -0.000000000000000000, -0.000000000000000000 ) ) ;
#24859=STYLED_ITEM ( 'NONE', ( #30696 ), #53984 ) ;
#24862=AXIS2_PLACEMENT_3D ( 'NONE', #43263, #12273, #27766 ) ;
#24866=PLANE ( 'NONE',  #51975 ) ;
#24868=EDGE_CURVE ( 'NONE', #7152, #21334, #85126, .T. ) ;
#24885=ORIENTED_EDGE ( 'NONE', *, *, #33522, .T. ) ;
#24888=VECTOR ( 'NONE', #11885, 1000.000000000000000 ) ;
#24890=DIRECTION ( 'NONE',  ( 0.7808688094430307203, -0.6246950475544238435, 0.000000000000000000 ) ) ;
#24898=ORIENTED_EDGE ( 'NONE', *, *, #32433, .F. ) ;
#24901=DIRECTION ( 'NONE',  ( 1.000000000000000000, 0.000000000000000000, 0.000000000000000000 ) ) ;
#24911=ORIENTED_EDGE ( 'NONE', *, *, #45781, .F. ) ;
#24914=EDGE_LOOP ( 'NONE', ( #88920, #5817, #96087, #17148 ) ) ;
#24920=CARTESIAN_POINT ( 'NONE',  ( -11.26270400852059872, -93.44583868494822809, 3.750000000000001776 ) ) ;
#24928=( NAMED_UNIT ( * ) PLANE_ANGLE_UNIT ( ) SI_UNIT ( $, .RADIAN. ) );
#24933=LINE ( 'NONE', #86413, #98416 ) ;
#24944=CARTESIAN_POINT ( 'NONE',  ( 6.574584770571507697, -50.88238473864101508, 2.750000000000000444 ) ) ;
#24949=EDGE_CURVE ( 'NONE', #46764, #97225, #22219, .T. ) ;
#24952=CARTESIAN_POINT ( 'NONE',  ( -1.899999999999997247, 98.49999999999998579, -8.525133428036873795 ) ) ;
#24961=DIRECTION ( 'NONE',  ( -0.000000000000000000, -0.000000000000000000, 1.000000000000000000 ) ) ;
#24962=SURFACE_SIDE_STYLE ('',( #83974 ) ) ;
#24968=( NAMED_UNIT ( * ) PLANE_ANGLE_UNIT ( ) SI_UNIT ( $, .RADIAN. ) );
#24980=ORIENTED_EDGE ( 'NONE', *, *, #40812, .F. ) ;
#24983=AXIS2_PLACEMENT_3D ( 'NONE', #68234, #14743, #62170 ) ;
#24985=EDGE_CURVE ( 'NONE', #15093, #96102, #9167, .T. ) ;
#24988=ADVANCED_FACE ( 'NONE', ( #17179 ), #88244, .T. ) ;
#24992=CARTESIAN_POINT ( 'NONE',  ( -3.499999999999998668, 1.019547802438465434, -2.750000000000000444 ) ) ;
#24996=( NAMED_UNIT ( * ) PLANE_ANGLE_UNIT ( ) SI_UNIT ( $, .RADIAN. ) );
#24997=FACE_OUTER_BOUND ( 'NONE', #77601, .T. ) ;
#25004=VERTEX_POINT ( 'NONE', #69676 ) ;
#25019=FACE_OUTER_BOUND ( 'NONE', #20317, .T. ) ;
#25031=COLOUR_RGB ( '', 0.66274510, 0.83137255, 0.94901961) ;
#25033=AXIS2_PLACEMENT_3D ( 'NONE', #97766, #22247, #61214 ) ;
#25037=ORIENTED_EDGE ( 'NONE', *, *, #96097, .T. ) ;
#25058=DIRECTION ( 'NONE',  ( -0.9997628902338809853, 0.02177529129993028070, 1.734723475976807292E-15 ) ) ;
#25063=DIRECTION ( 'NONE',  ( 0.000000000000000000, 0.000000000000000000, 1.000000000000000000 ) ) ;
#25075=CARTESIAN_POINT ( 'NONE',  ( -6.732636091893173358, -88.11213685669363826, -2.500000000000000000 ) ) ;
#25089=CARTESIAN_POINT ( 'NONE',  ( -3.750000000000000000, 37.00000000000000000, -4.000000000000000000 ) ) ;
#25098=CARTESIAN_POINT ( 'NONE',  ( -10.54702889484795669, -44.61188042013009891, 4.000000000000000888 ) ) ;
#25110=DIRECTION ( 'NONE',  ( -0.000000000000000000, -0.000000000000000000, -1.000000000000000000 ) ) ;
#25111=LINE ( 'NONE', #79064, #49627 ) ;
#25126=APPLICATION_CONTEXT ( 'automotive_design' ) ;
#25127=AXIS2_PLACEMENT_3D ( 'NONE', #48514, #2069, #25058 ) ;
#25128=CARTESIAN_POINT ( 'NONE',  ( -4.000000000000000000, 36.75000000000000000, 2.500000000000000000 ) ) ;
#25130=TOROIDAL_SURFACE ( 'NONE', #50650, 1.750000000000000888, 0.2500000000000000000 ) ;
#25132=ORIENTED_EDGE ( 'NONE', *, *, #50128, .F. ) ;
#25138=CARTESIAN_POINT ( 'NONE',  ( -10.09048698379360687, 46.92328126389585208, 0.000000000000000000 ) ) ;
#25144=DIRECTION ( 'NONE',  ( 0.000000000000000000, 0.000000000000000000, -1.000000000000000000 ) ) ;
#25163=VERTEX_POINT ( 'NONE', #48995 ) ;
#25187=DIRECTION ( 'NONE',  ( -1.000000000000000000, -6.938893903907221278E-15, 6.938893903907221278E-15 ) ) ;
#25194=AXIS2_PLACEMENT_3D ( 'NONE', #24186, #25662, #70174 ) ;
#25227=EDGE_CURVE ( 'NONE', #28519, #37810, #77182, .T. ) ;
#25228=UNCERTAINTY_MEASURE_WITH_UNIT (LENGTH_MEASURE( 1.000000000000000082E-05 ), #77653, 'distance_accuracy_value', 'NONE');
#25233=CARTESIAN_POINT ( 'NONE',  ( 18.00000000000000000, 84.07179676972448590, -12.00000000000000000 ) ) ;
#25262=CARTESIAN_POINT ( 'NONE',  ( -4.537879770909789556, -17.56524742836196040, 4.000000000004837908 ) ) ;
#25313=ORIENTED_EDGE ( 'NONE', *, *, #31695, .F. ) ;
#25326=DIRECTION ( 'NONE',  ( -0.000000000000000000, -0.000000000000000000, 1.000000000000000000 ) ) ;
#25336=DIRECTION ( 'NONE',  ( -0.000000000000000000, -0.000000000000000000, -1.000000000000000000 ) ) ;
#25337=CARTESIAN_POINT ( 'NONE',  ( -7.982674952684395642, 85.82256618331770426, -4.181766378585055399 ) ) ;
#25346=( LENGTH_UNIT ( ) NAMED_UNIT ( * ) SI_UNIT ( .MILLI., .METRE. ) );
#25352=CARTESIAN_POINT ( 'NONE',  ( 6.879999999999995453, 79.82179676972448590, 6.250000000000000000 ) ) ;
#25353=CARTESIAN_POINT ( 'NONE',  ( 11.18665108205495962, -81.61837458712054172, -3.999999999999999112 ) ) ;
#25364=FACE_OUTER_BOUND ( 'NONE', #30400, .T. ) ;
#25402=AXIS2_PLACEMENT_3D ( 'NONE', #98694, #4838, #42829 ) ;
#25417=CARTESIAN_POINT ( 'NONE',  ( -11.51441085139681597, -65.40266849241702118, 3.750000000000001332 ) ) ;
#25435=CARTESIAN_POINT ( 'NONE',  ( -4.250000000000000000, 10.00000000000000000, 3.750000000000000000 ) ) ;
#25442=CIRCLE ( 'NONE', #82943, 2.000000000000001776 ) ;
#25443=CARTESIAN_POINT ( 'NONE',  ( 4.655929185144718652, -8.243906417217084837, 2.500000000000000000 ) ) ;
#25454=ORIENTED_EDGE ( 'NONE', *, *, #75562, .F. ) ;
#25455=EDGE_CURVE ( 'NONE', #40665, #97363, #30180, .T. ) ;
#25458=CARTESIAN_POINT ( 'NONE',  ( -3.627483523066867388, -3.617667194782701934, -2.749999999999798383 ) ) ;
#25462=FILL_AREA_STYLE ('',( #54936 ) ) ;
#25466=( GEOMETRIC_REPRESENTATION_CONTEXT ( 3 ) GLOBAL_UNCERTAINTY_ASSIGNED_CONTEXT ( ( #34154 ) ) GLOBAL_UNIT_ASSIGNED_CONTEXT ( ( #53786, #82428, #38790 ) ) REPRESENTATION_CONTEXT ( 'NONE', 'WORKASPACE' ) );
#25495=ORIENTED_EDGE ( 'NONE', *, *, #97966, .F. ) ;
#25497=TOROIDAL_SURFACE ( 'NONE', #4724, 0.5000000000000000000, 0.2500000000000000000 ) ;
#25511=( NAMED_UNIT ( * ) PLANE_ANGLE_UNIT ( ) SI_UNIT ( $, .RADIAN. ) );
#25516=ORIENTED_EDGE ( 'NONE', *, *, #26997, .T. ) ;
#25517=CARTESIAN_POINT ( 'NONE',  ( 12.14357320772536575, 54.02013147999952736, -2.899999999999999467 ) ) ;
#25529=ORIENTED_EDGE ( 'NONE', *, *, #39416, .T. ) ;
#25541=ADVANCED_FACE ( 'NONE', ( #47150 ), #31167, .T. ) ;
#25551=FACE_OUTER_BOUND ( 'NONE', #81371, .T. ) ;
#25573=CARTESIAN_POINT ( 'NONE',  ( -10.17570567488967725, 89.26421072723884720, 5.905278573613795601 ) ) ;
#25582=DIRECTION ( 'NONE',  ( 1.000000000000000000, 0.000000000000000000, 0.000000000000000000 ) ) ;
#25593=CARTESIAN_POINT ( 'NONE',  ( -7.121364490415374782, -73.24716305332424326, -3.750000000000000000 ) ) ;
#25594=FILL_AREA_STYLE ('',( #10093 ) ) ;
#25600=CARTESIAN_POINT ( 'NONE',  ( -18.00000000000000355, 75.73428692542562146, -2.900000000000000799 ) ) ;
#25606=DIRECTION ( 'NONE',  ( -1.000000000000000000, 6.938893903907221278E-15, -6.938893903907221278E-15 ) ) ;
#25608=CARTESIAN_POINT ( 'NONE',  ( -3.750000000000000000, 9.750000000000000000, 3.750000000000000000 ) ) ;
#25610=CIRCLE ( 'NONE', #52785, 0.2500000000000002220 ) ;
#25621=( LENGTH_UNIT ( ) NAMED_UNIT ( * ) SI_UNIT ( .MILLI., .METRE. ) );
#25626=VERTEX_POINT ( 'NONE', #46191 ) ;
#25630=DIRECTION ( 'NONE',  ( 0.8070303256584298035, -0.5905099943842175847, 0.000000000000000000 ) ) ;
#25652=EDGE_LOOP ( 'NONE', ( #7297, #29430 ) ) ;
#25654=VECTOR ( 'NONE', #74088, 1000.000000000000114 ) ;
#25656=VERTEX_POINT ( 'NONE', #9165 ) ;
#25657=CARTESIAN_POINT ( 'NONE',  ( 11.10658183848185487, -52.67641232763428150, 3.750000000000000000 ) ) ;
#25662=DIRECTION ( 'NONE',  ( 0.000000000000000000, -1.000000000000000000, 0.000000000000000000 ) ) ;
#25666=PLANE ( 'NONE',  #70580 ) ;
#25669=VERTEX_POINT ( 'NONE', #84677 ) ;
#25670=FILL_AREA_STYLE ('',( #92666 ) ) ;
#25686=EDGE_CURVE ( 'NONE', #5283, #9418, #46667, .T. ) ;
#25697=CARTESIAN_POINT ( 'NONE',  ( 0.000000000000000000, 0.000000000000000000, 4.000000000000000000 ) ) ;
#25713=ORIENTED_EDGE ( 'NONE', *, *, #18543, .T. ) ;
#25714=CARTESIAN_POINT ( 'NONE',  ( 9.112669734029088531, -7.236323975083732485, -3.750000000000000000 ) ) ;
#25728=AXIS2_PLACEMENT_3D ( 'NONE', #42413, #87412, #48918 ) ;
#25743=CARTESIAN_POINT ( 'NONE',  ( 18.00000000000000000, 77.62863618568174218, 4.012044701512652800 ) ) ;
#25746=CARTESIAN_POINT ( 'NONE',  ( -7.072388532740516709, -84.40601219567591329, 3.750000000000806022 ) ) ;
#25755=EDGE_CURVE ( 'NONE', #6552, #59059, #14910, .T. ) ;
#25762=EDGE_LOOP ( 'NONE', ( #31146, #37046, #92747, #7863 ) ) ;
#25768=CARTESIAN_POINT ( 'NONE',  ( 6.879999999999995453, 41.24999999999999289, -6.500000000000000888 ) ) ;
#25774=CARTESIAN_POINT ( 'NONE',  ( 14.49999999999999822, 75.00000000000000000, 6.500000000000000888 ) ) ;
#25778=DIRECTION ( 'NONE',  ( -0.7971177707001962931, -0.6038238647436433570, 0.000000000000000000 ) ) ;
#25791=CARTESIAN_POINT ( 'NONE',  ( -7.803778109523453743, 84.96281847254653030, 4.037836297607493741 ) ) ;
#25804=CARTESIAN_POINT ( 'NONE',  ( 6.880000000000009663, 40.99999999999999289, -6.250000000000000000 ) ) ;
#25830=CARTESIAN_POINT ( 'NONE',  ( 10.95672020364514054, -56.81584260457095326, -4.000000000000000000 ) ) ;
#25832=FILL_AREA_STYLE_COLOUR ( '', #83308 ) ;
#25857=ORIENTED_EDGE ( 'NONE', *, *, #44829, .T. ) ;
#25861=EDGE_LOOP ( 'NONE', ( #97564, #77387, #20070, #92593 ) ) ;
#25872=VERTEX_POINT ( 'NONE', #49602 ) ;
#25882=CIRCLE ( 'NONE', #14761, 0.2500000000000002220 ) ;
#25886=ORIENTED_EDGE ( 'NONE', *, *, #59183, .T. ) ;
#25889=EDGE_CURVE ( 'NONE', #80133, #11363, #96344, .T. ) ;
#25895=CARTESIAN_POINT ( 'NONE',  ( -10.94537820540292117, -97.33546231743453347, 3.750000000000000444 ) ) ;
#25917=CARTESIAN_POINT ( 'NONE',  ( 6.829574850505125028, -88.00372650098201177, 2.500000000000000888 ) ) ;
#25921=CARTESIAN_POINT ( 'NONE',  ( 9.730292033379889460, -19.64198355330689338, 3.750000000000001332 ) ) ;
#25928=AXIS2_PLACEMENT_3D ( 'NONE', #65455, #6441, #52438 ) ;
#25932=FACE_OUTER_BOUND ( 'NONE', #24914, .T. ) ;
#25958=MECHANICAL_DESIGN_GEOMETRIC_PRESENTATION_REPRESENTATION('',(#86627),#38739);
#25986=ADVANCED_FACE ( 'NONE', ( #63141 ), #17666, .F. ) ;
#25988=CARTESIAN_POINT ( 'NONE',  ( -8.160079337347118766, -4.177753580735825700, -3.750000000000000444 ) ) ;
#25990=DIRECTION ( 'NONE',  ( 0.000000000000000000, -1.000000000000000000, 0.000000000000000000 ) ) ;
#26021=( GEOMETRIC_REPRESENTATION_CONTEXT ( 3 ) GLOBAL_UNCERTAINTY_ASSIGNED_CONTEXT ( ( #293 ) ) GLOBAL_UNIT_ASSIGNED_CONTEXT ( ( #85346, #84860, #93826 ) ) REPRESENTATION_CONTEXT ( 'NONE', 'WORKASPACE' ) );
#26022=ORIENTED_EDGE ( 'NONE', *, *, #18669, .F. ) ;
#26026=ORIENTED_EDGE ( 'NONE', *, *, #27106, .F. ) ;
#26027=DIRECTION ( 'NONE',  ( 1.000000000000000000, 0.000000000000000000, 0.000000000000000000 ) ) ;
#26028=CIRCLE ( 'NONE', #77123, 6.599999999999995204 ) ;
#26044=DIRECTION ( 'NONE',  ( 0.000000000000000000, -0.000000000000000000, -1.000000000000000000 ) ) ;
#26059=DIRECTION ( 'NONE',  ( -0.000000000000000000, 0.000000000000000000, 1.000000000000000000 ) ) ;
#26066=CIRCLE ( 'NONE', #81938, 9.999999999999998224 ) ;
#26067=CARTESIAN_POINT ( 'NONE',  ( -8.081444665946364125, -7.288330178564340400, 4.000000000000000000 ) ) ;
#26070=AXIS2_PLACEMENT_3D ( 'NONE', #77401, #75939, #53426 ) ;
#26072=DIRECTION ( 'NONE',  ( 0.000000000000000000, 1.000000000000000000, 0.000000000000000000 ) ) ;
#26079=DIRECTION ( 'NONE',  ( 1.000000000000000000, 0.000000000000000000, 0.000000000000000000 ) ) ;
#26092=DIRECTION ( 'NONE',  ( -0.000000000000000000, 0.000000000000000000, 1.000000000000000000 ) ) ;
#26100=AXIS2_PLACEMENT_3D ( 'NONE', #13389, #24844, #24359 ) ;
#26101=DIRECTION ( 'NONE',  ( -0.000000000000000000, 0.000000000000000000, 1.000000000000000000 ) ) ;
#26113=SURFACE_STYLE_FILL_AREA ( #79103 ) ;
#26121=DIRECTION ( 'NONE',  ( -0.000000000000000000, 0.000000000000000000, 1.000000000000000000 ) ) ;
#26127=ADVANCED_FACE ( 'NONE', ( #81098 ), #67089, .T. ) ;
#26129=EDGE_LOOP ( 'NONE', ( #96139, #33402, #48277, #31825 ) ) ;
#26137=CARTESIAN_POINT ( 'NONE',  ( 11.43665280331135392, -81.62088987012758423, 4.000000000000000000 ) ) ;
#26141=CARTESIAN_POINT ( 'NONE',  ( -7.118731320094870973, -71.92838106472885329, 3.750000000000000444 ) ) ;
#26159=DIRECTION ( 'NONE',  ( 0.000000000000000000, -0.000000000000000000, -1.000000000000000000 ) ) ;
#26171=CARTESIAN_POINT ( 'NONE',  ( -7.858204384621390481, -3.138042374757826991, -4.000000000000000000 ) ) ;
#26187=UNCERTAINTY_MEASURE_WITH_UNIT (LENGTH_MEASURE( 1.000000000000000082E-05 ), #59311, 'distance_accuracy_value', 'NONE');
#26193=CARTESIAN_POINT ( 'NONE',  ( 6.673414917871782315, -55.62670566514463388, 2.750000000000000000 ) ) ;
#26205=ORIENTED_EDGE ( 'NONE', *, *, #67589, .T. ) ;
#26222=CARTESIAN_POINT ( 'NONE',  ( 8.629999999999991900, 70.25000000000000000, -6.500000000000000888 ) ) ;
#26243=CARTESIAN_POINT ( 'NONE',  ( -18.89999999999999503, 98.99999999999998579, 7.750000000000000000 ) ) ;
#26246=SURFACE_STYLE_USAGE ( .BOTH. , #40768 ) ;
#26247=DIRECTION ( 'NONE',  ( 1.257402221000611116E-16, -1.000000000000000000, -0.000000000000000000 ) ) ;
#26260=AXIS2_PLACEMENT_3D ( 'NONE', #54842, #71350, #94324 ) ;
#26268=CARTESIAN_POINT ( 'NONE',  ( 6.935117329331543345, -80.58074665962956828, 2.750000000000000888 ) ) ;
#26282=CARTESIAN_POINT ( 'NONE',  ( -3.521924834447247132, -0.8399927508087468020, 2.750000000000001776 ) ) ;
#26287=CARTESIAN_POINT ( 'NONE',  ( -8.443706647342963834, 87.03308080853030049, -4.556631258847860799 ) ) ;
#26289=CARTESIAN_POINT ( 'NONE',  ( 11.34661744925197802, 54.08985607419764818, 3.000000000000000000 ) ) ;
#26290=TOROIDAL_SURFACE ( 'NONE', #51852, 10.09999999999999787, 0.1000000000000000056 ) ;
#26304=CARTESIAN_POINT ( 'NONE',  ( 10.09973302574091569, -32.02492402197682253, -4.000000000000000888 ) ) ;
#26313=EDGE_CURVE ( 'NONE', #94118, #87018, #21099, .T. ) ;
#26320=DIRECTION ( 'NONE',  ( 0.000000000000000000, 0.000000000000000000, 1.000000000000000000 ) ) ;
#26321=CARTESIAN_POINT ( 'NONE',  ( -9.000000000000000000, 75.76920769491746910, 3.000000000000000000 ) ) ;
#26330=VERTEX_POINT ( 'NONE', #82083 ) ;
#26349=ORIENTED_EDGE ( 'NONE', *, *, #41970, .T. ) ;
#26370=CARTESIAN_POINT ( 'NONE',  ( -10.79673003881345217, -98.50248976943588275, 3.750000000000000888 ) ) ;
#26379=FILL_AREA_STYLE_COLOUR ( '', #83764 ) ;
#26397=EDGE_CURVE ( 'NONE', #87849, #77456, #62846, .T. ) ;
#26405=LINE ( 'NONE', #3921, #5545 ) ;
#26406=CARTESIAN_POINT ( 'NONE',  ( -3.521047174886991815, -6.414748048905294375, -2.500000000000000000 ) ) ;
#26412=CARTESIAN_POINT ( 'NONE',  ( 6.910361961229144256, -84.29457034759302303, -3.999999999998390177 ) ) ;
#26422=CARTESIAN_POINT ( 'NONE',  ( 0.000000000000000000, -97.00000000000000000, -4.000000000000000000 ) ) ;
#26433=CIRCLE ( 'NONE', #96701, 0.2500000000000002220 ) ;
#26454=CARTESIAN_POINT ( 'NONE',  ( 4.879999999999991900, 76.07179676972444327, -4.250000000000000000 ) ) ;
#26463=FACE_OUTER_BOUND ( 'NONE', #5722, .T. ) ;
#26467=EDGE_CURVE ( 'NONE', #54753, #91690, #75620, .T. ) ;
#26476=AXIS2_PLACEMENT_3D ( 'NONE', #5266, #11765, #58225 ) ;
#26478=CARTESIAN_POINT ( 'NONE',  ( 9.879999999999988347, 26.99999999999999645, -2.900000000000000799 ) ) ;
#26484=LINE ( 'NONE', #72472, #47360 ) ;
#26485=EDGE_CURVE ( 'NONE', #70379, #79717, #58949, .T. ) ;
#26486=VERTEX_POINT ( 'NONE', #52575 ) ;
#26488=CARTESIAN_POINT ( 'NONE',  ( -5.078940136053647691, -28.66985681914853501, 2.499999999999999556 ) ) ;
#26498=CIRCLE ( 'NONE', #82386, 4.190000000000001279 ) ;
#26502=VERTEX_POINT ( 'NONE', #92537 ) ;
#26504=VECTOR ( 'NONE', #21211, 1000.000000000000000 ) ;
#26506=UNCERTAINTY_MEASURE_WITH_UNIT (LENGTH_MEASURE( 1.000000000000000082E-05 ), #91207, 'distance_accuracy_value', 'NONE');
#26507=CARTESIAN_POINT ( 'NONE',  ( -3.999999999999994671, 43.00000000000000711, -4.250000000000000000 ) ) ;
#26510=CARTESIAN_POINT ( 'NONE',  ( 6.880000000000009663, 40.99999999999999289, -6.250000000000000000 ) ) ;
#26513=ORIENTED_EDGE ( 'NONE', *, *, #92438, .F. ) ;
#26525=EDGE_LOOP ( 'NONE', ( #78739, #66967, #18864, #91131 ) ) ;
#26526=ADVANCED_FACE ( 'NONE', ( #31050 ), #90840, .T. ) ;
#26543=CARTESIAN_POINT ( 'NONE',  ( -8.647950603703787209, -15.58161425315404180, 4.000000000000000000 ) ) ;
#26565=DIRECTION ( 'NONE',  ( -1.000000000000000000, 3.035766082959409891E-14, 0.000000000000000000 ) ) ;
#26568=( BOUNDED_SURFACE ( )  B_SPLINE_SURFACE ( 3, 2, ( 
 ( #16942, #77421, #31427 ),
 ( #17445, #92921, #38955 ),
 ( #84939, #61931, #92432 ),
 ( #23956, #78417, #93916 ),
 ( #54430, #69447, #1956 ),
 ( #967, #54918, #62921 ),
 ( #8935, #25443, #70938 ),
 ( #39452, #32420, #77925 ),
 ( #69944, #93422, #76455 ),
 ( #23476, #7970, #15482 ),
 ( #493, #91945, #85433 ),
 ( #24944, #1464, #31916 ),
 ( #62417, #24452, #9934 ),
 ( #63411, #32911, #55926 ),
 ( #71896, #72382, #29225 ),
 ( #87878, #57872, #79412 ),
 ( #4410, #42397, #26892 ),
 ( #56419, #25917, #80393 ) ),
 .UNSPECIFIED., .F., .F., .T. ) 
 B_SPLINE_SURFACE_WITH_KNOTS ( ( 4, 2, 2, 2, 2, 2, 2, 2, 4 ),
 ( 3, 3 ),
 ( 0.000000000000000000, 0.002783459421197213672, 0.005566918842394427344, 0.01113383768478885469, 0.02226767536957770938, 0.04453535073915541875, 0.06680302610873312119, 0.07793686379352197935, 0.08907070147831083751 ),
 ( 0.000000000000000000, 1.000000000000000000 ),
 .UNSPECIFIED. ) 
 GEOMETRIC_REPRESENTATION_ITEM ( )  RATIONAL_B_SPLINE_SURFACE ( (
 ( 1.000000000000000000, 0.7071067811865482389, 1.000000000000000000),
 ( 1.000000000000000000, 0.7071067811865482389, 1.000000000000000000),
 ( 1.000000000000000000, 0.7071067811865482389, 1.000000000000000000),
 ( 1.000000000000000000, 0.7071067811865482389, 1.000000000000000000),
 ( 1.000000000000000000, 0.7071067811865482389, 1.000000000000000000),
 ( 1.000000000000000000, 0.7071067811865482389, 1.000000000000000000),
 ( 1.000000000000000000, 0.7071067811865482389, 1.000000000000000000),
 ( 1.000000000000000000, 0.7071067811865482389, 1.000000000000000000),
 ( 1.000000000000000000, 0.7071067811865482389, 1.000000000000000000),
 ( 1.000000000000000000, 0.7071067811865482389, 1.000000000000000000),
 ( 1.000000000000000000, 0.7071067811865465735, 1.000000000000000000),
 ( 1.000000000000000000, 0.7071067811865465735, 1.000000000000000000),
 ( 1.000000000000000000, 0.7071067811865482389, 1.000000000000000000),
 ( 1.000000000000000000, 0.7071067811865482389, 1.000000000000000000),
 ( 1.000000000000000000, 0.7071067811865482389, 1.000000000000000000),
 ( 1.000000000000000000, 0.7071067811865482389, 1.000000000000000000),
 ( 1.000000000000000000, 0.7071067811865476838, 1.000000000000000000),
 ( 1.000000000000000000, 0.7071067811865476838, 1.000000000000000000) ) ) 
 REPRESENTATION_ITEM ( '' )  SURFACE ( )  );
#26574=DIRECTION ( 'NONE',  ( -1.000000000000000000, 0.000000000000000000, 0.000000000000000000 ) ) ;
#26582=FILL_AREA_STYLE ('',( #10608 ) ) ;
#26587=EDGE_LOOP ( 'NONE', ( #94848, #28938, #40719, #72100 ) ) ;
#26593=CARTESIAN_POINT ( 'NONE',  ( 9.879999999999968807, 26.99999999999954170, -2.958578643762691307 ) ) ;
#26596=AXIS2_PLACEMENT_3D ( 'NONE', #23943, #14970, #14468 ) ;
#26609=FILL_AREA_STYLE ('',( #58085 ) ) ;
#26613=ORIENTED_EDGE ( 'NONE', *, *, #10850, .F. ) ;
#26619=EDGE_CURVE ( 'NONE', #80133, #70674, #14210, .T. ) ;
#26620=CARTESIAN_POINT ( 'NONE',  ( -6.757332319902496387, -55.97232334539076959, 2.750000000000000000 ) ) ;
#26626=PLANE ( 'NONE',  #89521 ) ;
#26647=CARTESIAN_POINT ( 'NONE',  ( -18.00000000000000355, 75.73428692542562146, 2.900000000000000355 ) ) ;
#26671=EDGE_CURVE ( 'NONE', #81788, #23479, #33372, .T. ) ;
#26673=CARTESIAN_POINT ( 'NONE',  ( 6.930493939446634499, -71.55570417525920845, 3.750000000000001776 ) ) ;
#26692=FILL_AREA_STYLE ('',( #85738 ) ) ;
#26703=SURFACE_STYLE_FILL_AREA ( #80200 ) ;
#26704=ORIENTED_EDGE ( 'NONE', *, *, #80880, .F. ) ;
#26706=VERTEX_POINT ( 'NONE', #10869 ) ;
#26721=VECTOR ( 'NONE', #27595, 1000.000000000000000 ) ;
#26729=AXIS2_PLACEMENT_3D ( 'NONE', #86649, #65594, #20105 ) ;
#26732=EDGE_LOOP ( 'NONE', ( #49622, #83528, #80584, #58308 ) ) ;
#26733=CYLINDRICAL_SURFACE ( 'NONE', #22346, 10.90000000000000036 ) ;
#26758=EDGE_CURVE ( 'NONE', #94992, #20984, #65280, .T. ) ;
#26764=CARTESIAN_POINT ( 'NONE',  ( -3.999999999999999112, 78.07179676972445748, -6.500000000000000888 ) ) ;
#26775=CARTESIAN_POINT ( 'NONE',  ( -4.536162600130072775, -17.54167793721155633, 2.750000000000002220 ) ) ;
#26780=CARTESIAN_POINT ( 'NONE',  ( -9.297374403301716939, 88.08016496434417775, -4.860721439949188039 ) ) ;
#26788=FILL_AREA_STYLE_COLOUR ( '', #88461 ) ;
#26790=DIRECTION ( 'NONE',  ( 0.000000000000000000, 0.000000000000000000, 1.000000000000000000 ) ) ;
#26800=DIRECTION ( 'NONE',  ( -0.000000000000000000, 0.000000000000000000, 1.000000000000000000 ) ) ;
#26822=ORIENTED_EDGE ( 'NONE', *, *, #40124, .F. ) ;
#26828=ORIENTED_EDGE ( 'NONE', *, *, #88988, .F. ) ;
#26831=LINE ( 'NONE', #95332, #5296 ) ;
#26841=ADVANCED_FACE ( 'NONE', ( #93868 ), #48363, .T. ) ;
#26850=VECTOR ( 'NONE', #56955, 1000.000000000000000 ) ;
#26866=LINE ( 'NONE', #40907, #83597 ) ;
#26870=DIRECTION ( 'NONE',  ( 1.000000000000000000, 1.257402221000611116E-16, -0.000000000000000000 ) ) ;
#26872=VERTEX_POINT ( 'NONE', #75795 ) ;
#26892=CARTESIAN_POINT ( 'NONE',  ( 6.660444548071449589, -84.28805632662712810, 2.500000000000001332 ) ) ;
#26894=VERTEX_POINT ( 'NONE', #2291 ) ;
#26903=CARTESIAN_POINT ( 'NONE',  ( -5.328486666255608739, -28.65465727419771724, -2.750000000000806466 ) ) ;
#26909=ORIENTED_EDGE ( 'NONE', *, *, #97966, .T. ) ;
#26910=CARTESIAN_POINT ( 'NONE',  ( 7.160361147697994255, -84.29732993326337009, -4.000000000000000000 ) ) ;
#26925=VECTOR ( 'NONE', #33820, 1000.000000000000000 ) ;
#26934=DIRECTION ( 'NONE',  ( 0.000000000000000000, 0.000000000000000000, 1.000000000000000000 ) ) ;
#26950=FACE_OUTER_BOUND ( 'NONE', #85639, .T. ) ;
#26952=DIRECTION ( 'NONE',  ( -1.000000000000000000, -1.927470528863119542E-16, 0.000000000000000000 ) ) ;
#26970=AXIS2_PLACEMENT_3D ( 'NONE', #46553, #31541, #62037 ) ;
#26976=CARTESIAN_POINT ( 'NONE',  ( -5.999999999999994671, 43.00000000000000000, 4.250000000000000000 ) ) ;
#26997=EDGE_CURVE ( 'NONE', #14094, #16059, #540, .T. ) ;
#27001=AXIS2_PLACEMENT_3D ( 'NONE', #56239, #78736, #10244 ) ;
#27018=DIRECTION ( 'NONE',  ( 1.000000000000000000, -0.000000000000000000, -0.000000000000000000 ) ) ;
#27025=CARTESIAN_POINT ( 'NONE',  ( -6.617298650316658204, -58.37178459782693096, -2.500000000000000000 ) ) ;
#27032=EDGE_CURVE ( 'NONE', #97225, #92281, #16501, .T. ) ;
#27036=CARTESIAN_POINT ( 'NONE',  ( 17.75000000000000355, 78.80384757729335377, -4.000000000000000000 ) ) ;
#27047=FACE_OUTER_BOUND ( 'NONE', #73306, .T. ) ;
#27054=FACE_OUTER_BOUND ( 'NONE', #35910, .T. ) ;
#27056=CIRCLE ( 'NONE', #19075, 0.09999999999999982514 ) ;
#27059=ORIENTED_EDGE ( 'NONE', *, *, #77550, .T. ) ;
#27064=CARTESIAN_POINT ( 'NONE',  ( -8.900000000000002132, 83.99999999999994316, -2.900000000000000799 ) ) ;
#27066=DIRECTION ( 'NONE',  ( 1.000000000000000000, 4.683753385137374737E-14, 0.000000000000000000 ) ) ;
#27075=DIRECTION ( 'NONE',  ( 1.000000000000000000, 0.000000000000000000, 0.000000000000000000 ) ) ;
#27084=ORIENTED_EDGE ( 'NONE', *, *, #29003, .T. ) ;
#27092=CARTESIAN_POINT ( 'NONE',  ( 0.000000000000000000, -97.00000000000000000, -4.000000000000000000 ) ) ;
#27102=CARTESIAN_POINT ( 'NONE',  ( 11.29389914963937969, -89.89072489379410058, 4.000000000000002665 ) ) ;
#27106=EDGE_CURVE ( 'NONE', #55108, #91827, #11125, .T. ) ;
#27111=SURFACE_SIDE_STYLE ('',( #64606 ) ) ;
#27114=DIRECTION ( 'NONE',  ( 1.000000000000000000, 0.000000000000000000, 0.000000000000000000 ) ) ;
#27123=CARTESIAN_POINT ( 'NONE',  ( 9.779999999999990479, 20.99999999999999645, 2.900000000000000355 ) ) ;
#27138=DIRECTION ( 'NONE',  ( 1.000000000000000000, 6.938893903907221278E-15, 0.000000000000000000 ) ) ;
#27153=UNCERTAINTY_MEASURE_WITH_UNIT (LENGTH_MEASURE( 1.000000000000000082E-05 ), #5641, 'distance_accuracy_value', 'NONE');
#27157=ORIENTED_EDGE ( 'NONE', *, *, #60667, .F. ) ;
#27159=CARTESIAN_POINT ( 'NONE',  ( 6.004190426492125532, -34.81345361117713111, 2.750000000000000000 ) ) ;
#27167=DIRECTION ( 'NONE',  ( 0.8070303256584298035, -0.5905099943842175847, 0.000000000000000000 ) ) ;
#27170=CARTESIAN_POINT ( 'NONE',  ( 6.685141491970859384, -80.57575624202263498, 2.500000000000000444 ) ) ;
#27173=DIRECTION ( 'NONE',  ( 1.000000000000000000, -0.000000000000000000, -0.000000000000000000 ) ) ;
#27189=ORIENTED_EDGE ( 'NONE', *, *, #54530, .F. ) ;
#27190=( NAMED_UNIT ( * ) SI_UNIT ( $, .STERADIAN. ) SOLID_ANGLE_UNIT ( ) );
#27198=ADVANCED_FACE ( 'NONE', ( #24997 ), #72426, .T. ) ;
#27201=EDGE_CURVE ( 'NONE', #81929, #60398, #62220, .T. ) ;
#27204=ORIENTED_EDGE ( 'NONE', *, *, #90290, .F. ) ;
#27216=AXIS2_PLACEMENT_3D ( 'NONE', #16246, #63200, #70234 ) ;
#27221=CARTESIAN_POINT ( 'NONE',  ( 4.879999999999994564, 43.00000000000000711, 6.250000000000000000 ) ) ;
#27227=AXIS2_PLACEMENT_3D ( 'NONE', #22033, #61482, #68511 ) ;
#27237=DIRECTION ( 'NONE',  ( 0.9961946980917462113, -0.08715574274765140739, 0.000000000000000000 ) ) ;
#27245=ORIENTED_EDGE ( 'NONE', *, *, #23632, .T. ) ;
#27249=FACE_OUTER_BOUND ( 'NONE', #95612, .T. ) ;
#27256=CARTESIAN_POINT ( 'NONE',  ( 6.934008441971972303, -73.15902683813038720, 3.750000000000000888 ) ) ;
#27263=CARTESIAN_POINT ( 'NONE',  ( -7.037775659072364576, -86.26045094518553924, 2.750000000000000444 ) ) ;
#27264=ORIENTED_EDGE ( 'NONE', *, *, #16116, .T. ) ;
#27270=FACE_OUTER_BOUND ( 'NONE', #70382, .T. ) ;
#27274=EDGE_LOOP ( 'NONE', ( #85761, #42296, #21686, #7278 ) ) ;
#27276=CARTESIAN_POINT ( 'NONE',  ( -8.000000000000000000, 80.32179676972448590, 4.250000000000000000 ) ) ;
#27285=( NAMED_UNIT ( * ) SI_UNIT ( $, .STERADIAN. ) SOLID_ANGLE_UNIT ( ) );
#27290=STYLED_ITEM ( 'NONE', ( #54576 ), #61971 ) ;
#27291=VERTEX_POINT ( 'NONE', #54963 ) ;
#27293=DIRECTION ( 'NONE',  ( 1.000000000000000000, -0.000000000000000000, -0.000000000000000000 ) ) ;
#27303=CARTESIAN_POINT ( 'NONE',  ( 4.130000000000000782, 0.09092508112526098696, -2.499999999999999556 ) ) ;
#27306=DIRECTION ( 'NONE',  ( -1.000000000000000000, 0.000000000000000000, 0.000000000000000000 ) ) ;
#27309=ADVANCED_FACE ( 'NONE', ( #3468 ), #25497, .T. ) ;
#27325=ADVANCED_FACE ( 'NONE', ( #77973 ), #18460, .F. ) ;
#27328=ORIENTED_EDGE ( 'NONE', *, *, #22702, .T. ) ;
#27344=CARTESIAN_POINT ( 'NONE',  ( -8.000000000000000000, 40.74999999999999289, 3.750000000000000000 ) ) ;
#27356=CARTESIAN_POINT ( 'NONE',  ( 6.880000000000009663, 40.99999999999999289, -6.500000000000000888 ) ) ;
#27362=ORIENTED_EDGE ( 'NONE', *, *, #942, .F. ) ;
#27363=EDGE_CURVE ( 'NONE', #50168, #30576, #35912, .T. ) ;
#27371=DIRECTION ( 'NONE',  ( 0.000000000000000000, 0.000000000000000000, 1.000000000000000000 ) ) ;
#27391=SURFACE_SIDE_STYLE ('',( #87889 ) ) ;
#27399=CARTESIAN_POINT ( 'NONE',  ( 6.825238882348372726, -50.90120388559804354, -4.000000000000000000 ) ) ;
#27403=CARTESIAN_POINT ( 'NONE',  ( -5.320211218918609930, -24.96484130673367474, 4.000000000000000888 ) ) ;
#27412=DIRECTION ( 'NONE',  ( 1.000000000000000000, 0.000000000000000000, 0.000000000000000000 ) ) ;
#27423=DIRECTION ( 'NONE',  ( -0.000000000000000000, -0.000000000000000000, -1.000000000000000000 ) ) ;
#27424=DIRECTION ( 'NONE',  ( 0.000000000000000000, 0.000000000000000000, 1.000000000000000000 ) ) ;
#27439=CARTESIAN_POINT ( 'NONE',  ( 4.441537491767904022, -2.700695904837609351, 3.750000000000000000 ) ) ;
#27451=DIRECTION ( 'NONE',  ( 0.000000000000000000, -0.000000000000000000, -1.000000000000000000 ) ) ;
#27468=DIRECTION ( 'NONE',  ( 0.000000000000000000, -1.000000000000000000, 0.000000000000000000 ) ) ;
#27469=EDGE_CURVE ( 'NONE', #94718, #13092, #82934, .T. ) ;
#27476=CARTESIAN_POINT ( 'NONE',  ( -4.285674571761296292, -17.54407107685944212, 2.500000000000000888 ) ) ;
#27483=CARTESIAN_POINT ( 'NONE',  ( 4.630000000000003446, 1.019547802438464545, 4.000000000000000000 ) ) ;
#27495=CARTESIAN_POINT ( 'NONE',  ( 6.930493939446634499, -71.55570417525920845, -2.750000000000000000 ) ) ;
#27508=FACE_OUTER_BOUND ( 'NONE', #3137, .T. ) ;
#27517=VECTOR ( 'NONE', #12677, 1000.000000000000114 ) ;
#27521=CIRCLE ( 'NONE', #92980, 0.2500000000000000000 ) ;
#27527=VECTOR ( 'NONE', #33758, 999.9999999999998863 ) ;
#27538=ORIENTED_EDGE ( 'NONE', *, *, #90990, .T. ) ;
#27541=DIRECTION ( 'NONE',  ( -0.000000000000000000, -0.000000000000000000, -1.000000000000000000 ) ) ;
#27549=CARTESIAN_POINT ( 'NONE',  ( 10.35038117927457968, -32.03264712071879927, -3.750000000000000888 ) ) ;
#27550=CARTESIAN_POINT ( 'NONE',  ( -3.772435417270373570, -6.430908609833668521, -3.750000000000000000 ) ) ;
#27556=EDGE_CURVE ( 'NONE', #56519, #70269, #44397, .T. ) ;
#27558=DIRECTION ( 'NONE',  ( -1.000000000000000000, 0.000000000000000000, 0.000000000000000000 ) ) ;
#27563=DIRECTION ( 'NONE',  ( -0.000000000000000000, 0.000000000000000000, 1.000000000000000000 ) ) ;
#27580=VERTEX_POINT ( 'NONE', #42442 ) ;
#27581=CIRCLE ( 'NONE', #22823, 0.2500000000000002220 ) ;
#27583=CIRCLE ( 'NONE', #56368, 0.2500000000000002220 ) ;
#27586=AXIS2_PLACEMENT_3D ( 'NONE', #31876, #16412, #23918 ) ;
#27593=CYLINDRICAL_SURFACE ( 'NONE', #42609, 0.2500000000000002220 ) ;
#27595=DIRECTION ( 'NONE',  ( -1.483861936729427615E-16, 1.000000000000000000, 0.000000000000000000 ) ) ;
#27600=VERTEX_POINT ( 'NONE', #17735 ) ;
#27603=COLOUR_RGB ( '', 0.31764706, 0.68627451, 0.89019608) ;
#27604=CARTESIAN_POINT ( 'NONE',  ( -6.982525766139713319, -88.11956320875633253, 3.750000000000000444 ) ) ;
#27606=DIRECTION ( 'NONE',  ( -1.000000000000000000, 4.510281037539694659E-14, 0.000000000000000000 ) ) ;
#27611=FACE_OUTER_BOUND ( 'NONE', #94102, .T. ) ;
#27616=FILL_AREA_STYLE ('',( #2695 ) ) ;
#27631=FILL_AREA_STYLE_COLOUR ( '', #5705 ) ;
#27637=CARTESIAN_POINT ( 'NONE',  ( -11.63911236830571916, -77.84336773400802656, -3.750000000000000000 ) ) ;
#27641=EDGE_CURVE ( 'NONE', #5883, #23594, #87840, .T. ) ;
#27642=SURFACE_SIDE_STYLE ('',( #96158 ) ) ;
#27652=VERTEX_POINT ( 'NONE', #70244 ) ;
#27664=ORIENTED_EDGE ( 'NONE', *, *, #72416, .F. ) ;
#27673=ADVANCED_FACE ( 'NONE', ( #45384 ), #78720, .F. ) ;
#27678=SURFACE_STYLE_FILL_AREA ( #4709 ) ;
#27695=MECHANICAL_DESIGN_GEOMETRIC_PRESENTATION_REPRESENTATION('',(#14950),#10152);
#27700=ORIENTED_EDGE ( 'NONE', *, *, #80581, .T. ) ;
#27721=DIRECTION ( 'NONE',  ( -0.000000000000000000, -0.000000000000000000, -1.000000000000000000 ) ) ;
#27722=EDGE_LOOP ( 'NONE', ( #11217, #26349, #6161, #78355, #21378 ) ) ;
#27724=FACE_OUTER_BOUND ( 'NONE', #15768, .T. ) ;
#27749=LINE ( 'NONE', #88255, #58540 ) ;
#27752=CARTESIAN_POINT ( 'NONE',  ( 4.573290919439518376, -6.402485759401510101, 3.750000000000000444 ) ) ;
#27753=( LENGTH_UNIT ( ) NAMED_UNIT ( * ) SI_UNIT ( .MILLI., .METRE. ) );
#27758=CARTESIAN_POINT ( 'NONE',  ( -6.867514901617631118, -58.37540207706140194, 2.749999999999999556 ) ) ;
#27764=CARTESIAN_POINT ( 'NONE',  ( -12.29167862325965821, 90.46743899975646741, -7.079701151216127641 ) ) ;
#27766=DIRECTION ( 'NONE',  ( 0.000000000000000000, 0.000000000000000000, -1.000000000000000000 ) ) ;
#27771=DIRECTION ( 'NONE',  ( 1.000000000000000000, 0.000000000000000000, 0.000000000000000000 ) ) ;
#27772=DIRECTION ( 'NONE',  ( 1.927470528863119542E-16, -1.000000000000000000, -0.000000000000000000 ) ) ;
#27789=EDGE_CURVE ( 'NONE', #75926, #89237, #78220, .T. ) ;
#27790=VECTOR ( 'NONE', #1760, 1000.000000000000000 ) ;
#27799=CARTESIAN_POINT ( 'NONE',  ( 18.00000000000000000, 78.80384757729336798, 3.750000000000000000 ) ) ;
#27802=AXIS2_PLACEMENT_3D ( 'NONE', #89619, #50635, #89124 ) ;
#27804=CYLINDRICAL_SURFACE ( 'NONE', #62113, 0.2500000000000002220 ) ;
#27805=ORIENTED_EDGE ( 'NONE', *, *, #44993, .T. ) ;
#27814=CYLINDRICAL_SURFACE ( 'NONE', #25402, 0.2500000000000002220 ) ;
#27820=EDGE_LOOP ( 'NONE', ( #66502, #96209, #91892, #68307 ) ) ;
#27822=EDGE_LOOP ( 'NONE', ( #67173, #44455, #28322, #83049 ) ) ;
#27842=CARTESIAN_POINT ( 'NONE',  ( -13.79715839871649763, 90.89647188945875200, -7.777600768747879201 ) ) ;
#27846=CARTESIAN_POINT ( 'NONE',  ( -3.750000000000000000, 36.75000000000000000, 2.500000000000000000 ) ) ;
#27847=DIRECTION ( 'NONE',  ( 0.000000000000000000, 0.000000000000000000, -1.000000000000000000 ) ) ;
#27874=SURFACE_STYLE_USAGE ( .BOTH. , #20880 ) ;
#27876=DIRECTION ( 'NONE',  ( 1.000000000000000000, -0.000000000000000000, -0.000000000000000000 ) ) ;
#27890=CARTESIAN_POINT ( 'NONE',  ( 6.935087012919454175, -80.58470470491536730, -4.000000000001609379 ) ) ;
#27891=LINE ( 'NONE', #58887, #86169 ) ;
#27893=CARTESIAN_POINT ( 'NONE',  ( -4.511864039100093926, -13.83704418182128038, 3.999999999999999112 ) ) ;
#27909=ORIENTED_EDGE ( 'NONE', *, *, #50128, .T. ) ;
#27930=LINE ( 'NONE', #96960, #87590 ) ;
#27931=AXIS2_PLACEMENT_3D ( 'NONE', #67341, #59335, #50356 ) ;
#27936=AXIS2_PLACEMENT_3D ( 'NONE', #98854, #30308, #52818 ) ;
#27972=CARTESIAN_POINT ( 'NONE',  ( 5.170517050971797701, -13.81852248048419263, 4.000000000000000000 ) ) ;
#27986=ORIENTED_EDGE ( 'NONE', *, *, #35113, .F. ) ;
#27994=DIRECTION ( 'NONE',  ( 1.000000000000000000, 1.257402221000612102E-16, 0.000000000000000000 ) ) ;
#28001=PRESENTATION_STYLE_ASSIGNMENT (( #66000 ) ) ;
#28017=SURFACE_SIDE_STYLE ('',( #51519 ) ) ;
#28044=AXIS2_PLACEMENT_3D ( 'NONE', #72627, #57634, #34133 ) ;
#28047=ORIENTED_EDGE ( 'NONE', *, *, #87534, .T. ) ;
#28053=CARTESIAN_POINT ( 'NONE',  ( -15.00000000000000000, 83.99999999999998579, -4.000000000000000000 ) ) ;
#28063=CARTESIAN_POINT ( 'NONE',  ( -3.750000000000000000, 10.25000000000000000, -2.750000000000000000 ) ) ;
#28064=ORIENTED_EDGE ( 'NONE', *, *, #92560, .F. ) ;
#28097=CARTESIAN_POINT ( 'NONE',  ( -3.521970993462044230, -0.8418523783473399469, 3.750000000000000444 ) ) ;
#28104=CARTESIAN_POINT ( 'NONE',  ( 8.880000000000000782, 1.019547802438459216, 3.750000000000000000 ) ) ;
#28109=CARTESIAN_POINT ( 'NONE',  ( 3.969999999999999751, 0.000000000000000000, 2.750000000000000000 ) ) ;
#28115=ADVANCED_FACE ( 'NONE', ( #17519 ), #68175, .F. ) ;
#28121=SURFACE_SIDE_STYLE ('',( #6124 ) ) ;
#28122=CARTESIAN_POINT ( 'NONE',  ( -16.94999999999999574, 99.99999999999998579, -7.750000000000000000 ) ) ;
#28126=ADVANCED_FACE ( 'NONE', ( #26463 ), #95967, .T. ) ;
#28132=CARTESIAN_POINT ( 'NONE',  ( -11.38910604374480506, -77.84323126540351723, -4.000000000000000000 ) ) ;
#28137=DIRECTION ( 'NONE',  ( -0.06975647374410356982, -0.9975640502598257520, 0.000000000000000000 ) ) ;
#28140=STYLED_ITEM ( 'NONE', ( #8814 ), #42728 ) ;
#28161=AXIS2_PLACEMENT_3D ( 'NONE', #98751, #76695, #82719 ) ;
#28168=CARTESIAN_POINT ( 'NONE',  ( 8.880000000000020322, 80.07179676972448590, -4.250000000000000000 ) ) ;
#28171=CIRCLE ( 'NONE', #79275, 0.2500000000000002220 ) ;
#28175=CARTESIAN_POINT ( 'NONE',  ( -16.94999999999999574, 99.99999999999998579, 7.750000000000000000 ) ) ;
#28185=ORIENTED_EDGE ( 'NONE', *, *, #37407, .F. ) ;
#28186=PRESENTATION_STYLE_ASSIGNMENT (( #88685 ) ) ;
#28187=ORIENTED_EDGE ( 'NONE', *, *, #32045, .F. ) ;
#28192=DIRECTION ( 'NONE',  ( 1.000000000000000000, 0.000000000000000000, 0.000000000000000000 ) ) ;
#28199=ORIENTED_EDGE ( 'NONE', *, *, #72493, .T. ) ;
#28205=CARTESIAN_POINT ( 'NONE',  ( -11.64999999999999680, 98.49999999999998579, -8.525133428036873795 ) ) ;
#28211=PLANE ( 'NONE',  #81862 ) ;
#28219=DIRECTION ( 'NONE',  ( 0.000000000000000000, -1.000000000000000000, 0.000000000000000000 ) ) ;
#28233=CARTESIAN_POINT ( 'NONE',  ( -13.87912815710419068, 90.90967772850538609, 7.772688653987089857 ) ) ;
#28238=PLANE ( 'NONE',  #34575 ) ;
#28242=CARTESIAN_POINT ( 'NONE',  ( 6.880000000000009663, 40.99999999999999289, 6.500000000000000888 ) ) ;
#28248=FACE_OUTER_BOUND ( 'NONE', #71439, .T. ) ;
#28262=( NAMED_UNIT ( * ) PLANE_ANGLE_UNIT ( ) SI_UNIT ( $, .RADIAN. ) );
#28269=SURFACE_STYLE_FILL_AREA ( #66765 ) ;
#28281=CARTESIAN_POINT ( 'NONE',  ( 8.630000000000000782, 1.085138116723527427E-15, -6.250000000000000000 ) ) ;
#28301=STYLED_ITEM ( 'NONE', ( #18022 ), #11513 ) ;
#28305=ORIENTED_EDGE ( 'NONE', *, *, #34448, .F. ) ;
#28310=AXIS2_PLACEMENT_3D ( 'NONE', #79871, #49369, #11375 ) ;
#28312=ORIENTED_EDGE ( 'NONE', *, *, #2682, .F. ) ;
#28313=AXIS2_PLACEMENT_3D ( 'NONE', #53008, #7542, #92484 ) ;
#28322=ORIENTED_EDGE ( 'NONE', *, *, #4085, .T. ) ;
#28327=DIRECTION ( 'NONE',  ( -1.927470528863119542E-16, 1.000000000000000000, 0.000000000000000000 ) ) ;
#28334=DIRECTION ( 'NONE',  ( 0.000000000000000000, -0.000000000000000000, -1.000000000000000000 ) ) ;
#28355=DIRECTION ( 'NONE',  ( -1.000000000000000000, -1.927470528863119542E-16, 0.000000000000000000 ) ) ;
#28362=CARTESIAN_POINT ( 'NONE',  ( 1.350000000000004086, 98.49999999999998579, 8.000000000000000000 ) ) ;
#28365=CARTESIAN_POINT ( 'NONE',  ( -10.17570567488968081, 89.26421072723886141, -5.905278573613798265 ) ) ;
#28374=VERTEX_POINT ( 'NONE', #79481 ) ;
#28378=FACE_OUTER_BOUND ( 'NONE', #398, .T. ) ;
#28379=AXIS2_PLACEMENT_3D ( 'NONE', #53147, #66679, #60149 ) ;
#28380=FACE_OUTER_BOUND ( 'NONE', #61405, .T. ) ;
#28385=CARTESIAN_POINT ( 'NONE',  ( -6.617417514236028531, -58.37570470593282579, -2.500000000000000000 ) ) ;
#28392=DIRECTION ( 'NONE',  ( -0.000000000000000000, -0.000000000000000000, -1.000000000000000000 ) ) ;
#28393=CARTESIAN_POINT ( 'NONE',  ( -10.53011945866294852, -98.59345040283277228, -4.000000000000000000 ) ) ;
#28429=CARTESIAN_POINT ( 'NONE',  ( 4.380000000000001670, 1.019547802438464768, 4.000000000000000000 ) ) ;
#28430=FILL_AREA_STYLE ('',( #36432 ) ) ;
#28439=ADVANCED_FACE ( 'NONE', ( #46535 ), #83563, .T. ) ;
#28444=VECTOR ( 'NONE', #65099, 1000.000000000000000 ) ;
#28452=MECHANICAL_DESIGN_GEOMETRIC_PRESENTATION_REPRESENTATION('',(#15696),#78052);
#28454=AXIS2_PLACEMENT_3D ( 'NONE', #88562, #87091, #11099 ) ;
#28465=DIRECTION ( 'NONE',  ( 1.000000000000000000, 0.000000000000000000, 0.000000000000000000 ) ) ;
#28474=VERTEX_POINT ( 'NONE', #79743 ) ;
#28475=CARTESIAN_POINT ( 'NONE',  ( 7.185089000015947747, -80.58569572050201657, 3.999999999999999112 ) ) ;
#28482=ADVANCED_FACE ( 'NONE', ( #18759 ), #26733, .T. ) ;
#28487=CARTESIAN_POINT ( 'NONE',  ( 3.969999999999999751, 10.25000000000000000, -3.750000000000000000 ) ) ;
#28489=FACE_OUTER_BOUND ( 'NONE', #29284, .T. ) ;
#28512=CARTESIAN_POINT ( 'NONE',  ( -6.871316085749034741, -73.24163895400424451, -2.500000000000000000 ) ) ;
#28518=FACE_OUTER_BOUND ( 'NONE', #65681, .T. ) ;
#28519=VERTEX_POINT ( 'NONE', #97235 ) ;
#28522=AXIS2_PLACEMENT_3D ( 'NONE', #71274, #55774, #24304 ) ;
#28530=ORIENTED_EDGE ( 'NONE', *, *, #44833, .F. ) ;
#28544=( BOUNDED_SURFACE ( )  B_SPLINE_SURFACE ( 3, 2, ( 
 ( #15299, #60278, #38286 ),
 ( #52774, #76275, #13799 ),
 ( #794, #46272, #76757 ),
 ( #8275, #59780, #31247 ),
 ( #51796, #74789, #36800 ),
 ( #67294, #97821, #63712 ),
 ( #32231, #85749, #85255 ),
 ( #17261, #55746, #64199 ),
 ( #16270, #25262, #70259 ),
 ( #71724, #2764, #18235 ),
 ( #3233, #62732, #9746 ),
 ( #32726, #31744, #1291 ),
 ( #47736, #40737, #62240 ),
 ( #93232, #23785, #54250 ),
 ( #33219, #8755, #16763 ),
 ( #92746, #86733, #78233 ),
 ( #24757, #55235, #48716 ),
 ( #24270, #40248, #41248 ),
 ( #33699, #70756, #94216 ),
 ( #2270, #84762, #25746 ),
 ( #93729, #54736, #63224 ),
 ( #46752, #47236, #86237 ) ),
 .UNSPECIFIED., .F., .F., .T. ) 
 B_SPLINE_SURFACE_WITH_KNOTS ( ( 4, 2, 2, 2, 2, 2, 2, 2, 2, 2, 4 ),
 ( 3, 3 ),
 ( -1.040834085586084257E-17, 0.002789288213736764842, 0.005578576427473540093, 0.01115715285494709059, 0.02231430570989419160, 0.03347145856484129434, 0.04462861141978839707, 0.06694291712968260255, 0.07810006998462970529, 0.08367864641210326360, 0.08925722283957680803 ),
 ( 0.000000000000000000, 1.000000000000000000 ),
 .UNSPECIFIED. ) 
 GEOMETRIC_REPRESENTATION_ITEM ( )  RATIONAL_B_SPLINE_SURFACE ( (
 ( 1.000000000000000000, 0.7071067811865482389, 1.000000000000000000),
 ( 1.000000000000000000, 0.7071067811865482389, 1.000000000000000000),
 ( 1.000000000000000000, 0.7071067811865493491, 1.000000000000000000),
 ( 1.000000000000000000, 0.7071067811865493491, 1.000000000000000000),
 ( 1.000000000000000000, 0.7071067811865475727, 1.000000000000000000),
 ( 1.000000000000000000, 0.7071067811865475727, 1.000000000000000000),
 ( 1.000000000000000000, 0.7071067811865475727, 1.000000000000000000),
 ( 1.000000000000000000, 0.7071067811865475727, 1.000000000000000000),
 ( 1.000000000000000000, 0.7071067811865487940, 1.000000000000000000),
 ( 1.000000000000000000, 0.7071067811865487940, 1.000000000000000000),
 ( 1.000000000000000000, 0.7071067811865475727, 1.000000000000000000),
 ( 1.000000000000000000, 0.7071067811865475727, 1.000000000000000000),
 ( 1.000000000000000000, 0.7071067811865487940, 1.000000000000000000),
 ( 1.000000000000000000, 0.7071067811865487940, 1.000000000000000000),
 ( 1.000000000000000000, 0.7071067811865463515, 1.000000000000000000),
 ( 1.000000000000000000, 0.7071067811865463515, 1.000000000000000000),
 ( 1.000000000000000000, 0.7071067811865456854, 1.000000000000000000),
 ( 1.000000000000000000, 0.7071067811865456854, 1.000000000000000000),
 ( 1.000000000000000000, 0.7071067811865475727, 1.000000000000000000),
 ( 1.000000000000000000, 0.7071067811865475727, 1.000000000000000000),
 ( 1.000000000000000000, 0.7071067811865475727, 1.000000000000000000),
 ( 1.000000000000000000, 0.7071067811865475727, 1.000000000000000000) ) ) 
 REPRESENTATION_ITEM ( '' )  SURFACE ( )  );
#28546=CARTESIAN_POINT ( 'NONE',  ( 11.27041535450084631, -90.94092909150046466, -3.750000000000000000 ) ) ;
#28562=EDGE_LOOP ( 'NONE', ( #6185, #77661, #54555, #98607 ) ) ;
#28598=CARTESIAN_POINT ( 'NONE',  ( -3.888850863501575716, -8.270211729787575905, 3.750000000000000888 ) ) ;
#28602=ORIENTED_EDGE ( 'NONE', *, *, #15726, .T. ) ;
#28620=CARTESIAN_POINT ( 'NONE',  ( -3.530007528296587704, -1.230351260576522110, -3.750000000000000000 ) ) ;
#28640=ORIENTED_EDGE ( 'NONE', *, *, #68773, .T. ) ;
#28642=CYLINDRICAL_SURFACE ( 'NONE', #58962, 0.2500000000000002220 ) ;
#28646=EDGE_CURVE ( 'NONE', #58305, #2418, #89209, .T. ) ;
#28665=PRESENTATION_STYLE_ASSIGNMENT (( #20182 ) ) ;
#28677=VERTEX_POINT ( 'NONE', #29679 ) ;
#28694=MECHANICAL_DESIGN_GEOMETRIC_PRESENTATION_REPRESENTATION('',(#76585),#52750);
#28702=AXIS2_PLACEMENT_3D ( 'NONE', #2086, #63533, #93049 ) ;
#28705=CARTESIAN_POINT ( 'NONE',  ( 8.629999999999995453, 41.24999999999999289, 6.250000000000000000 ) ) ;
#28710=DIRECTION ( 'NONE',  ( -0.000000000000000000, 1.000000000000000000, 0.000000000000000000 ) ) ;
#28712=ORIENTED_EDGE ( 'NONE', *, *, #60792, .T. ) ;
#28714=DIRECTION ( 'NONE',  ( 0.000000000000000000, -0.000000000000000000, -1.000000000000000000 ) ) ;
#28718=DIRECTION ( 'NONE',  ( 0.000000000000000000, 1.000000000000000000, 0.000000000000000000 ) ) ;
#28719=CARTESIAN_POINT ( 'NONE',  ( -15.00000000000000000, 83.99999999999998579, 4.000000000000000000 ) ) ;
#28726=CARTESIAN_POINT ( 'NONE',  ( -10.09048698379360687, 46.92328126389585208, 0.000000000000000000 ) ) ;
#28743=AXIS2_PLACEMENT_3D ( 'NONE', #72338, #28327, #3870 ) ;
#28755=CARTESIAN_POINT ( 'NONE',  ( -13.45431060380788502, 90.84076481352336430, -7.653071044409292867 ) ) ;
#28756=SURFACE_STYLE_USAGE ( .BOTH. , #51263 ) ;
#28762=SURFACE_SIDE_STYLE ('',( #28269 ) ) ;
#28774=EDGE_LOOP ( 'NONE', ( #89573, #87379, #51668, #14811 ) ) ;
#28776=( LENGTH_UNIT ( ) NAMED_UNIT ( * ) SI_UNIT ( .MILLI., .METRE. ) );
#28786=DIRECTION ( 'NONE',  ( -0.08715574274765415519, -0.9961946980917458783, 0.000000000000000000 ) ) ;
#28789=SURFACE_STYLE_FILL_AREA ( #19328 ) ;
#28803=CIRCLE ( 'NONE', #51149, 0.2500000000000002220 ) ;
#28814=VECTOR ( 'NONE', #87720, 1000.000000000000000 ) ;
#28833=AXIS2_PLACEMENT_3D ( 'NONE', #24684, #25187, #9673 ) ;
#28839=DIRECTION ( 'NONE',  ( 0.000000000000000000, 0.000000000000000000, -1.000000000000000000 ) ) ;
#28841=CARTESIAN_POINT ( 'NONE',  ( -10.79772875661416087, 89.74400587740484525, -6.349085400557793690 ) ) ;
#28845=CARTESIAN_POINT ( 'NONE',  ( -18.00000000000000355, 75.73428692542562146, -3.000000000000000000 ) ) ;
#28853=CARTESIAN_POINT ( 'NONE',  ( 14.99999999999998046, 69.99999999999998579, 6.250000000000000000 ) ) ;
#28866=COLOUR_RGB ( '', 0.40784314, 0.44705882, 0.49803922) ;
#28870=CYLINDRICAL_SURFACE ( 'NONE', #581, 0.2500000000000002220 ) ;
#28871=DIRECTION ( 'NONE',  ( -0.000000000000000000, -1.000000000000000000, -0.000000000000000000 ) ) ;
#28885=CARTESIAN_POINT ( 'NONE',  ( 6.579634127946654587, -87.99828267815715321, 3.750000000000000000 ) ) ;
#28899=CIRCLE ( 'NONE', #52890, 0.4999999999999995559 ) ;
#28905=ORIENTED_EDGE ( 'NONE', *, *, #14389, .T. ) ;
#28909=SURFACE_STYLE_FILL_AREA ( #97445 ) ;
#28919=EDGE_CURVE ( 'NONE', #28474, #13062, #23698, .T. ) ;
#28938=ORIENTED_EDGE ( 'NONE', *, *, #58216, .T. ) ;
#28948=EDGE_CURVE ( 'NONE', #51986, #26486, #95281, .T. ) ;
#28951=CARTESIAN_POINT ( 'NONE',  ( 10.93736952761193670, -97.13260119835408091, 4.000000000000000000 ) ) ;
#28967=CARTESIAN_POINT ( 'NONE',  ( -18.89999999999999503, 98.99999999999998579, -8.000000000000000000 ) ) ;
#28999=CARTESIAN_POINT ( 'NONE',  ( 6.579634127946654587, -87.99828267815715321, 2.750000000000000888 ) ) ;
#29001=VECTOR ( 'NONE', #15132, 1000.000000000000000 ) ;
#29003=EDGE_CURVE ( 'NONE', #21081, #76760, #74033, .T. ) ;
#29008=DIRECTION ( 'NONE',  ( -1.000000000000000000, 0.000000000000000000, 0.000000000000000000 ) ) ;
#29025=CARTESIAN_POINT ( 'NONE',  ( 10.86470958188973768, -97.91370008131707436, -3.750000000016808333 ) ) ;
#29026=CARTESIAN_POINT ( 'NONE',  ( -7.037696230105376927, -86.26312365675100580, -3.750000000000000000 ) ) ;
#29032=DIRECTION ( 'NONE',  ( -0.000000000000000000, 0.000000000000000000, 1.000000000000000000 ) ) ;
#29038=DIRECTION ( 'NONE',  ( -0.000000000000000000, 0.000000000000000000, 1.000000000000000000 ) ) ;
#29040=EDGE_CURVE ( 'NONE', #35385, #8055, #53506, .T. ) ;
#29044=ORIENTED_EDGE ( 'NONE', *, *, #96550, .F. ) ;
#29063=ORIENTED_EDGE ( 'NONE', *, *, #71677, .T. ) ;
#29071=CARTESIAN_POINT ( 'NONE',  ( 11.19532980485324103, -77.48602862270493574, 4.000000000000000000 ) ) ;
#29086=DIRECTION ( 'NONE',  ( 0.000000000000000000, 0.000000000000000000, -1.000000000000000000 ) ) ;
#29097=DIRECTION ( 'NONE',  ( 0.000000000000000000, 0.000000000000000000, 1.000000000000000000 ) ) ;
#29104=FACE_OUTER_BOUND ( 'NONE', #2353, .T. ) ;
#29106=CARTESIAN_POINT ( 'NONE',  ( 5.800000000000003375, 99.99999999999998579, -8.525133428036873795 ) ) ;
#29115=FACE_OUTER_BOUND ( 'NONE', #86617, .T. ) ;
#29138=ORIENTED_EDGE ( 'NONE', *, *, #21641, .T. ) ;
#29156=DIRECTION ( 'NONE',  ( 0.000000000000000000, 0.000000000000000000, 1.000000000000000000 ) ) ;
#29162=CARTESIAN_POINT ( 'NONE',  ( 8.879999999999991900, 76.07179676972447169, -4.000000000000000000 ) ) ;
#29163=AXIS2_PLACEMENT_3D ( 'NONE', #19286, #72761, #41326 ) ;
#29192=( GEOMETRIC_REPRESENTATION_CONTEXT ( 3 ) GLOBAL_UNCERTAINTY_ASSIGNED_CONTEXT ( ( #49495 ) ) GLOBAL_UNIT_ASSIGNED_CONTEXT ( ( #75690, #21720, #7706 ) ) REPRESENTATION_CONTEXT ( 'NONE', 'WORKASPACE' ) );
#29194=DIRECTION ( 'NONE',  ( -1.049065152435176504E-16, 1.000000000000000000, -0.000000000000000000 ) ) ;
#29196=PLANE ( 'NONE',  #62126 ) ;
#29202=DIRECTION ( 'NONE',  ( -1.000000000000000000, -0.000000000000000000, -0.000000000000000000 ) ) ;
#29208=DIRECTION ( 'NONE',  ( -1.000000000000000000, 0.000000000000000000, 0.000000000000000000 ) ) ;
#29225=CARTESIAN_POINT ( 'NONE',  ( 6.683985746567200792, -73.15435785430807414, 2.500000000000000888 ) ) ;
#29231=MECHANICAL_DESIGN_GEOMETRIC_PRESENTATION_REPRESENTATION('',(#16482),#54778);
#29237=FACE_OUTER_BOUND ( 'NONE', #58482, .T. ) ;
#29242=EDGE_LOOP ( 'NONE', ( #70038, #21086, #46632 ) ) ;
#29248=CARTESIAN_POINT ( 'NONE',  ( 4.219999999999999751, 36.75000000000000000, -3.750000000000000000 ) ) ;
#29254=CARTESIAN_POINT ( 'NONE',  ( 11.40632470798694342, -69.21560994247114706, -3.750000000000000000 ) ) ;
#29268=CIRCLE ( 'NONE', #50038, 2.899999999999999023 ) ;
#29271=CARTESIAN_POINT ( 'NONE',  ( 0.2510757737844357407, 80.99999999999994316, 0.000000000000000000 ) ) ;
#29280=CARTESIAN_POINT ( 'NONE',  ( -7.750000000000000000, 80.32179676972448590, -4.250000000000000000 ) ) ;
#29284=EDGE_LOOP ( 'NONE', ( #65613, #85369, #29296, #28047 ) ) ;
#29290=LINE ( 'NONE', #74288, #15327 ) ;
#29295=EDGE_CURVE ( 'NONE', #62733, #25669, #8994, .T. ) ;
#29296=ORIENTED_EDGE ( 'NONE', *, *, #9727, .T. ) ;
#29299=EDGE_LOOP ( 'NONE', ( #35072, #77263, #84584, #41938 ) ) ;
#29301=STYLED_ITEM ( 'NONE', ( #33260 ), #77673 ) ;
#29318=SURFACE_SIDE_STYLE ('',( #54287 ) ) ;
#29327=SURFACE_STYLE_FILL_AREA ( #95883 ) ;
#29331=CARTESIAN_POINT ( 'NONE',  ( 6.910443788714468738, -84.29081344360214700, -2.749999999994367617 ) ) ;
#29334=ORIENTED_EDGE ( 'NONE', *, *, #22608, .T. ) ;
#29347=EDGE_LOOP ( 'NONE', ( #90257, #21204, #72433, #4998 ) ) ;
#29364=ORIENTED_EDGE ( 'NONE', *, *, #24514, .T. ) ;
#29365=VECTOR ( 'NONE', #37741, 1000.000000000000114 ) ;
#29366=CARTESIAN_POINT ( 'NONE',  ( 17.75000000000001776, 4.561680251642722724E-15, -3.750000000000000000 ) ) ;
#29367=CARTESIAN_POINT ( 'NONE',  ( -10.09048698379360864, 46.92328126389585208, -3.000000000000000000 ) ) ;
#29375=CARTESIAN_POINT ( 'NONE',  ( -15.00000000000004974, 91.25000000000000000, 7.750000000000000000 ) ) ;
#29388=DIRECTION ( 'NONE',  ( 0.000000000000000000, 1.000000000000000000, 0.000000000000000000 ) ) ;
#29394=ORIENTED_EDGE ( 'NONE', *, *, #40916, .F. ) ;
#29399=DIRECTION ( 'NONE',  ( -0.000000000000000000, 0.000000000000000000, 1.000000000000000000 ) ) ;
#29404=FACE_OUTER_BOUND ( 'NONE', #73995, .T. ) ;
#29408=CARTESIAN_POINT ( 'NONE',  ( -3.999999999999994671, 43.00000000000000711, -6.500000000000000888 ) ) ;
#29423=CIRCLE ( 'NONE', #24668, 0.09999999999999939493 ) ;
#29430=ORIENTED_EDGE ( 'NONE', *, *, #76753, .T. ) ;
#29435=CARTESIAN_POINT ( 'NONE',  ( -6.822528426060553208, -84.39592987140930802, 2.500000000000000000 ) ) ;
#29440=CARTESIAN_POINT ( 'NONE',  ( 6.825220758711188829, -50.90060425938847288, -4.000000000000000000 ) ) ;
#29454=DIRECTION ( 'NONE',  ( 1.483861936729427615E-16, -1.000000000000000000, -0.000000000000000000 ) ) ;
#29462=SURFACE_SIDE_STYLE ('',( #66989 ) ) ;
#29484=SURFACE_STYLE_USAGE ( .BOTH. , #14022 ) ;
#29488=DIRECTION ( 'NONE',  ( -0.000000000000000000, 0.000000000000000000, 1.000000000000000000 ) ) ;
#29495=DIRECTION ( 'NONE',  ( 0.000000000000000000, 0.000000000000000000, -1.000000000000000000 ) ) ;
#29497=PRESENTATION_STYLE_ASSIGNMENT (( #61483 ) ) ;
#29513=CARTESIAN_POINT ( 'NONE',  ( -5.811454672277545974, -36.11427488547636955, -3.999999999998387956 ) ) ;
#29532=VERTEX_POINT ( 'NONE', #71930 ) ;
#29534=DIRECTION ( 'NONE',  ( -0.000000000000000000, 0.000000000000000000, 1.000000000000000000 ) ) ;
#29547=VERTEX_POINT ( 'NONE', #32939 ) ;
#29570=LINE ( 'NONE', #35610, #67429 ) ;
#29579=DIRECTION ( 'NONE',  ( 0.000000000000000000, -0.000000000000000000, -1.000000000000000000 ) ) ;
#29599=CARTESIAN_POINT ( 'NONE',  ( 3.969999999999999751, 10.25000000000000000, -2.500000000000000000 ) ) ;
#29603=CARTESIAN_POINT ( 'NONE',  ( 4.629999999999999893, 4.857171655774867594E-16, 4.000000000000000000 ) ) ;
#29609=MECHANICAL_DESIGN_GEOMETRIC_PRESENTATION_REPRESENTATION('',(#64713),#47166);
#29615=SURFACE_SIDE_STYLE ('',( #75627 ) ) ;
#29628=VECTOR ( 'NONE', #40431, 1000.000000000000000 ) ;
#29635=CARTESIAN_POINT ( 'NONE',  ( -11.16005593728303324, -52.90553718812902417, 4.000000000003606004 ) ) ;
#29640=AXIS2_PLACEMENT_3D ( 'NONE', #1495, #46961, #8969 ) ;
#29642=SURFACE_STYLE_USAGE ( .BOTH. , #98185 ) ;
#29648=SURFACE_STYLE_FILL_AREA ( #67682 ) ;
#29657=LINE ( 'NONE', #69651, #12904 ) ;
#29671=DIRECTION ( 'NONE',  ( -0.000000000000000000, -0.000000000000000000, -1.000000000000000000 ) ) ;
#29677=CARTESIAN_POINT ( 'NONE',  ( 12.99999999999999822, 75.00000000000000000, 6.500000000000000888 ) ) ;
#29678=ORIENTED_EDGE ( 'NONE', *, *, #17411, .F. ) ;
#29679=CARTESIAN_POINT ( 'NONE',  ( 4.469999999999999751, 36.75000000000000000, 4.000000000000000000 ) ) ;
#29682=EDGE_CURVE ( 'NONE', #75564, #55756, #37403, .T. ) ;
#29690=FACE_OUTER_BOUND ( 'NONE', #93029, .T. ) ;
#29696=FILL_AREA_STYLE ('',( #51731 ) ) ;
#29701=COLOUR_RGB ( '', 0.08235294, 0.09019608, 0.10196078) ;
#29714=ADVANCED_FACE ( 'NONE', ( #59878 ), #42916, .F. ) ;
#29715=DIRECTION ( 'NONE',  ( -1.000000000000000000, -0.000000000000000000, -0.000000000000000000 ) ) ;
#29734=CARTESIAN_POINT ( 'NONE',  ( -7.750000000000000000, 79.82179676972448590, 4.250000000000000000 ) ) ;
#29740=CARTESIAN_POINT ( 'NONE',  ( 9.511402282543471642, -15.49422404099329498, -3.750000000000000000 ) ) ;
#29746=( NAMED_UNIT ( * ) SI_UNIT ( $, .STERADIAN. ) SOLID_ANGLE_UNIT ( ) );
#29750=( NAMED_UNIT ( * ) PLANE_ANGLE_UNIT ( ) SI_UNIT ( $, .RADIAN. ) );
#29762=DIRECTION ( 'NONE',  ( 0.000000000000000000, 1.000000000000000000, 0.000000000000000000 ) ) ;
#29766=PRESENTATION_STYLE_ASSIGNMENT (( #7292 ) ) ;
#29769=ORIENTED_EDGE ( 'NONE', *, *, #86431, .T. ) ;
#29774=ORIENTED_EDGE ( 'NONE', *, *, #31392, .T. ) ;
#29779=EDGE_LOOP ( 'NONE', ( #82081, #69671, #60038, #26613 ) ) ;
#29783=AXIS2_PLACEMENT_3D ( 'NONE', #12596, #34102, #66590 ) ;
#29788=ORIENTED_EDGE ( 'NONE', *, *, #3169, .F. ) ;
#29794=DIRECTION ( 'NONE',  ( 0.000000000000000000, 1.000000000000000000, 0.000000000000000000 ) ) ;
#29797=VECTOR ( 'NONE', #93897, 1000.000000000000000 ) ;
#29817=( LENGTH_UNIT ( ) NAMED_UNIT ( * ) SI_UNIT ( .MILLI., .METRE. ) );
#29823=CARTESIAN_POINT ( 'NONE',  ( 6.033511671519392827, -36.04540650267304613, -2.499999999999998224 ) ) ;
#29839=( LENGTH_UNIT ( ) NAMED_UNIT ( * ) SI_UNIT ( .MILLI., .METRE. ) );
#29843=DIRECTION ( 'NONE',  ( 0.000000000000000000, 0.000000000000000000, 1.000000000000000000 ) ) ;
#29847=ORIENTED_EDGE ( 'NONE', *, *, #6565, .F. ) ;
#29851=DIRECTION ( 'NONE',  ( 0.9995586998285053149, 0.02970531260815256758, 0.000000000000000000 ) ) ;
#29862=( GEOMETRIC_REPRESENTATION_CONTEXT ( 3 ) GLOBAL_UNCERTAINTY_ASSIGNED_CONTEXT ( ( #35142 ) ) GLOBAL_UNIT_ASSIGNED_CONTEXT ( ( #48010, #71031, #17048 ) ) REPRESENTATION_CONTEXT ( 'NONE', 'WORKASPACE' ) );
#29864=DIRECTION ( 'NONE',  ( 0.000000000000000000, 1.000000000000000000, 0.000000000000000000 ) ) ;
#29903=CARTESIAN_POINT ( 'NONE',  ( -3.750000000000000888, 1.019547802438465212, -4.000000000000000000 ) ) ;
#29913=CARTESIAN_POINT ( 'NONE',  ( 8.879999999999991900, 27.04366094290857347, -2.900000000000000799 ) ) ;
#29924=DIRECTION ( 'NONE',  ( 0.000000000000000000, -0.000000000000000000, -1.000000000000000000 ) ) ;
#29932=CARTESIAN_POINT ( 'NONE',  ( -6.030006457149878152, -39.79017371238850842, 2.750000000000000000 ) ) ;
#29937=CARTESIAN_POINT ( 'NONE',  ( 5.170517050971795037, -13.81852248048418375, -3.999999999999999112 ) ) ;
#29940=VECTOR ( 'NONE', #83280, 1000.000000000000000 ) ;
#29946=CARTESIAN_POINT ( 'NONE',  ( -9.286179496273216927, 88.06418697516217264, 4.851265792411716404 ) ) ;
#29968=ORIENTED_EDGE ( 'NONE', *, *, #68437, .T. ) ;
#29977=DIRECTION ( 'NONE',  ( -0.000000000000000000, -0.000000000000000000, 1.000000000000000000 ) ) ;
#29978=DIRECTION ( 'NONE',  ( 0.000000000000000000, 0.000000000000000000, -1.000000000000000000 ) ) ;
#29986=DIRECTION ( 'NONE',  ( 0.000000000000000000, 0.000000000000000000, 1.000000000000000000 ) ) ;
#30011=ADVANCED_FACE ( 'NONE', ( #77341 ), #7887, .T. ) ;
#30012=VECTOR ( 'NONE', #53603, 1000.000000000000000 ) ;
#30014=CARTESIAN_POINT ( 'NONE',  ( -7.117921737451715636, -58.38558715620306572, -3.999999999999999112 ) ) ;
#30015=AXIS2_PLACEMENT_3D ( 'NONE', #86729, #18231, #10727 ) ;
#30058=ORIENTED_EDGE ( 'NONE', *, *, #15576, .T. ) ;
#30063=TOROIDAL_SURFACE ( 'NONE', #52427, 2.899999999999999911, 0.1000000000000000056 ) ;
#30066=LINE ( 'NONE', #36608, #3497 ) ;
#30068=DIRECTION ( 'NONE',  ( -0.000000000000000000, 0.000000000000000000, 1.000000000000000000 ) ) ;
#30073=CARTESIAN_POINT ( 'NONE',  ( 8.880000000000000782, -7.313785530894214126, -3.750000000000001776 ) ) ;
#30076=ADVANCED_FACE ( 'NONE', ( #33788 ), #47827, .T. ) ;
#30078=DIRECTION ( 'NONE',  ( 0.000000000000000000, -1.000000000000000000, 0.000000000000000000 ) ) ;
#30080=SURFACE_SIDE_STYLE ('',( #22606 ) ) ;
#30082=ORIENTED_EDGE ( 'NONE', *, *, #3545, .T. ) ;
#30104=LINE ( 'NONE', #76112, #30012 ) ;
#30111=ORIENTED_EDGE ( 'NONE', *, *, #35698, .F. ) ;
#30118=MECHANICAL_DESIGN_GEOMETRIC_PRESENTATION_REPRESENTATION('',(#73151),#42911);
#30131=CARTESIAN_POINT ( 'NONE',  ( -11.48887051628074829, -88.22984412037166635, 4.000000000000000000 ) ) ;
#30142=CARTESIAN_POINT ( 'NONE',  ( 17.75000000000000355, 77.07179676972445748, -6.250000000000000000 ) ) ;
#30145=CARTESIAN_POINT ( 'NONE',  ( -7.750000000000000000, 0.000000000000000000, 4.000000000000000000 ) ) ;
#30150=FACE_OUTER_BOUND ( 'NONE', #15652, .T. ) ;
#30153=( GEOMETRIC_REPRESENTATION_CONTEXT ( 3 ) GLOBAL_UNCERTAINTY_ASSIGNED_CONTEXT ( ( #93212 ) ) GLOBAL_UNIT_ASSIGNED_CONTEXT ( ( #69301, #31281, #92291 ) ) REPRESENTATION_CONTEXT ( 'NONE', 'WORKASPACE' ) );
#30160=EDGE_CURVE ( 'NONE', #37917, #22102, #55839, .T. ) ;
#30162=ORIENTED_EDGE ( 'NONE', *, *, #87136, .T. ) ;
#30168=CARTESIAN_POINT ( 'NONE',  ( -8.000000000000000000, 40.99999999999999289, 6.500000000000000888 ) ) ;
#30171=( GEOMETRIC_REPRESENTATION_CONTEXT ( 3 ) GLOBAL_UNCERTAINTY_ASSIGNED_CONTEXT ( ( #87169 ) ) GLOBAL_UNIT_ASSIGNED_CONTEXT ( ( #814, #67816, #7808 ) ) REPRESENTATION_CONTEXT ( 'NONE', 'WORKASPACE' ) );
#30172=DIRECTION ( 'NONE',  ( 0.000000000000000000, 0.000000000000000000, 1.000000000000000000 ) ) ;
#30173=ORIENTED_EDGE ( 'NONE', *, *, #56016, .T. ) ;
#30177=ORIENTED_EDGE ( 'NONE', *, *, #85707, .F. ) ;
#30180=LINE ( 'NONE', #69189, #62771 ) ;
#30185=CIRCLE ( 'NONE', #84533, 0.2500000000000002220 ) ;
#30198=DIRECTION ( 'NONE',  ( -1.000000000000000000, 0.000000000000000000, 0.000000000000000000 ) ) ;
#30207=MECHANICAL_DESIGN_GEOMETRIC_PRESENTATION_REPRESENTATION('',(#9454),#4689);
#30226=UNCERTAINTY_MEASURE_WITH_UNIT (LENGTH_MEASURE( 1.000000000000000082E-05 ), #63751, 'distance_accuracy_value', 'NONE');
#30232=CARTESIAN_POINT ( 'NONE',  ( 11.40632470801588028, -69.21560994247100496, -4.000000000000000000 ) ) ;
#30237=SURFACE_STYLE_USAGE ( .BOTH. , #15276 ) ;
#30247=ORIENTED_EDGE ( 'NONE', *, *, #92595, .F. ) ;
#30249=DIRECTION ( 'NONE',  ( -0.08715574274765112983, -0.9961946980917461003, 0.000000000000000000 ) ) ;
#30260=CARTESIAN_POINT ( 'NONE',  ( 6.683977931330435496, -73.15273079452120442, -2.499999999999999556 ) ) ;
#30267=ORIENTED_EDGE ( 'NONE', *, *, #91561, .T. ) ;
#30270=ORIENTED_EDGE ( 'NONE', *, *, #84933, .T. ) ;
#30274=VECTOR ( 'NONE', #28871, 1000.000000000000000 ) ;
#30275=CARTESIAN_POINT ( 'NONE',  ( 4.469999999999999751, 10.00000000000000000, 3.750000000000000000 ) ) ;
#30280=ORIENTED_EDGE ( 'NONE', *, *, #21359, .F. ) ;
#30289=ORIENTED_EDGE ( 'NONE', *, *, #71498, .T. ) ;
#30297=LINE ( 'NONE', #83316, #70643 ) ;
#30298=AXIS2_PLACEMENT_3D ( 'NONE', #39656, #78628, #10139 ) ;
#30308=DIRECTION ( 'NONE',  ( -0.000000000000000000, 0.000000000000000000, 1.000000000000000000 ) ) ;
#30317=CARTESIAN_POINT ( 'NONE',  ( 5.113979357103554335, -17.50950876244569443, -2.750000000000804246 ) ) ;
#30327=DIRECTION ( 'NONE',  ( 0.000000000000000000, 1.000000000000000000, 0.000000000000000000 ) ) ;
#30333=( LENGTH_UNIT ( ) NAMED_UNIT ( * ) SI_UNIT ( .MILLI., .METRE. ) );
#30336=DIRECTION ( 'NONE',  ( 1.000000000000000000, 0.000000000000000000, 0.000000000000000000 ) ) ;
#30337=ORIENTED_EDGE ( 'NONE', *, *, #50212, .F. ) ;
#30340=LINE ( 'NONE', #92820, #61069 ) ;
#30350=CARTESIAN_POINT ( 'NONE',  ( -7.749999999999999112, -0.02153525003578424246, -4.000000000000000000 ) ) ;
#30363=CIRCLE ( 'NONE', #55937, 0.2500000000000002220 ) ;
#30368=EDGE_CURVE ( 'NONE', #89066, #91549, #77398, .T. ) ;
#30369=ADVANCED_FACE ( 'NONE', ( #39912 ), #31542, .T. ) ;
#30375=DIRECTION ( 'NONE',  ( 1.000000000000000000, 2.081668171172167567E-14, 0.000000000000000000 ) ) ;
#30379=CIRCLE ( 'NONE', #9625, 0.09999999999999939493 ) ;
#30383=AXIS2_PLACEMENT_3D ( 'NONE', #1799, #63737, #15807 ) ;
#30392=CARTESIAN_POINT ( 'NONE',  ( -3.750000000000000000, 10.25000000000000000, -2.500000000000000000 ) ) ;
#30398=CARTESIAN_POINT ( 'NONE',  ( -8.000000000000000000, 80.99999999999994316, -1.249999999999987121 ) ) ;
#30400=EDGE_LOOP ( 'NONE', ( #51595, #23096, #4728, #84177 ) ) ;
#30401=EDGE_CURVE ( 'NONE', #22141, #2391, #49110, .T. ) ;
#30416=ORIENTED_EDGE ( 'NONE', *, *, #20390, .F. ) ;
#30421=ORIENTED_EDGE ( 'NONE', *, *, #33005, .F. ) ;
#30437=UNCERTAINTY_MEASURE_WITH_UNIT (LENGTH_MEASURE( 1.000000000000000082E-05 ), #9479, 'distance_accuracy_value', 'NONE');
#30438=CARTESIAN_POINT ( 'NONE',  ( -14.89999999999999680, 98.49999999999998579, -8.525133428036873795 ) ) ;
#30440=VECTOR ( 'NONE', #37026, 1000.000000000000000 ) ;
#30448=AXIS2_PLACEMENT_3D ( 'NONE', #92153, #61152, #196 ) ;
#30463=SURFACE_STYLE_USAGE ( .BOTH. , #24962 ) ;
#30479=AXIS2_PLACEMENT_3D ( 'NONE', #83606, #15614, #46578 ) ;
#30490=DIRECTION ( 'NONE',  ( -0.000000000000000000, -0.000000000000000000, -1.000000000000000000 ) ) ;
#30499=DIRECTION ( 'NONE',  ( -1.000000000000000000, 0.000000000000000000, 0.000000000000000000 ) ) ;
#30522=ADVANCED_FACE ( 'NONE', ( #49858 ), #66425, .T. ) ;
#30523=CARTESIAN_POINT ( 'NONE',  ( -4.250000000000000000, 36.75000000000000000, 4.000000000000000000 ) ) ;
#30525=VERTEX_POINT ( 'NONE', #96958 ) ;
#30527=ORIENTED_EDGE ( 'NONE', *, *, #11281, .T. ) ;
#30534=DIRECTION ( 'NONE',  ( 0.000000000000000000, 0.000000000000000000, 1.000000000000000000 ) ) ;
#30537=VERTEX_POINT ( 'NONE', #5940 ) ;
#30547=( GEOMETRIC_REPRESENTATION_CONTEXT ( 3 ) GLOBAL_UNCERTAINTY_ASSIGNED_CONTEXT ( ( #38134 ) ) GLOBAL_UNIT_ASSIGNED_CONTEXT ( ( #12870, #43369, #21372 ) ) REPRESENTATION_CONTEXT ( 'NONE', 'WORKASPACE' ) );
#30550=CARTESIAN_POINT ( 'NONE',  ( 8.862917522023083805, -7.247543382038870163, 4.000000000000000000 ) ) ;
#30555=CARTESIAN_POINT ( 'NONE',  ( -3.750000000000000000, 10.00000000000000000, -2.750000000000000000 ) ) ;
#30561=FILL_AREA_STYLE ('',( #47044 ) ) ;
#30569=ADVANCED_FACE ( 'NONE', ( #67921 ), #92018, .F. ) ;
#30576=VERTEX_POINT ( 'NONE', #35928 ) ;
#30598=EDGE_CURVE ( 'NONE', #24464, #69208, #94463, .T. ) ;
#30605=ORIENTED_EDGE ( 'NONE', *, *, #20806, .T. ) ;
#30614=CARTESIAN_POINT ( 'NONE',  ( -19.89999999999999858, 98.99999999999998579, 8.000000000000000000 ) ) ;
#30623=CARTESIAN_POINT ( 'NONE',  ( -9.543970587277799567, -28.01866822100916465, 4.000000000000000000 ) ) ;
#30642=CARTESIAN_POINT ( 'NONE',  ( -19.64999999999999858, 0.000000000000000000, -7.750000000000000000 ) ) ;
#30652=CIRCLE ( 'NONE', #32291, 0.1000000000000001166 ) ;
#30659=MECHANICAL_DESIGN_GEOMETRIC_PRESENTATION_REPRESENTATION('',(#61006),#9992);
#30661=CARTESIAN_POINT ( 'NONE',  ( -6.732636091893172470, -88.11213685669366669, 2.750000000000000444 ) ) ;
#30674=DIRECTION ( 'NONE',  ( 0.000000000000000000, 1.000000000000000000, -0.000000000000000000 ) ) ;
#30687=ADVANCED_FACE ( 'NONE', ( #26950 ), #4954, .T. ) ;
#30691=ORIENTED_EDGE ( 'NONE', *, *, #26619, .T. ) ;
#30696=PRESENTATION_STYLE_ASSIGNMENT (( #75220 ) ) ;
#30698=FILL_AREA_STYLE ('',( #69215 ) ) ;
#30722=AXIS2_PLACEMENT_3D ( 'NONE', #4143, #73100, #27114 ) ;
#30728=CARTESIAN_POINT ( 'NONE',  ( 11.44533173451573660, -77.48526441101033413, -3.750000000000000000 ) ) ;
#30732=CARTESIAN_POINT ( 'NONE',  ( 6.879999999999995453, 70.25000000000000000, 6.500000000000000888 ) ) ;
#30742=DIRECTION ( 'NONE',  ( 0.6246950475544237324, 0.7808688094430306093, 0.000000000000000000 ) ) ;
#30754=VECTOR ( 'NONE', #81464, 999.9999999999998863 ) ;
#30756=VERTEX_POINT ( 'NONE', #65929 ) ;
#30764=ADVANCED_FACE ( 'NONE', ( #18478, #41978 ), #96457, .F. ) ;
#30765=( NAMED_UNIT ( * ) SI_UNIT ( $, .STERADIAN. ) SOLID_ANGLE_UNIT ( ) );
#30772=EDGE_CURVE ( 'NONE', #89406, #96102, #72939, .T. ) ;
#30773=SURFACE_SIDE_STYLE ('',( #21446 ) ) ;
#30778=FILL_AREA_STYLE_COLOUR ( '', #68934 ) ;
#30782=COLOUR_RGB ( '', 0.31764706, 0.68627451, 0.89019608) ;
#30790=MECHANICAL_DESIGN_GEOMETRIC_PRESENTATION_REPRESENTATION('',(#16402),#48357);
#30802=( NAMED_UNIT ( * ) SI_UNIT ( $, .STERADIAN. ) SOLID_ANGLE_UNIT ( ) );
#30803=CARTESIAN_POINT ( 'NONE',  ( -6.982525766850298687, -88.11956318484570261, -2.750000000000000444 ) ) ;
#30806=SURFACE_SIDE_STYLE ('',( #9296 ) ) ;
#30813=CARTESIAN_POINT ( 'NONE',  ( 5.429204171141014612, -28.64228857766720537, -2.499999999999999112 ) ) ;
#30818=CARTESIAN_POINT ( 'NONE',  ( 5.114679605280758601, -17.52310038230844924, 2.750000000000000000 ) ) ;
#30822=( GEOMETRIC_REPRESENTATION_CONTEXT ( 3 ) GLOBAL_UNCERTAINTY_ASSIGNED_CONTEXT ( ( #32194 ) ) GLOBAL_UNIT_ASSIGNED_CONTEXT ( ( #66925, #89918, #19943 ) ) REPRESENTATION_CONTEXT ( 'NONE', 'WORKASPACE' ) );
#30824=FACE_OUTER_BOUND ( 'NONE', #56994, .T. ) ;
#30829=CARTESIAN_POINT ( 'NONE',  ( 0.4400000000000020006, 1.019547802438468986, -3.750000000000000000 ) ) ;
#30832=CARTESIAN_POINT ( 'NONE',  ( -8.159336008669392015, -4.163137246823999327, -3.750000000000000000 ) ) ;
#30834=AXIS2_PLACEMENT_3D ( 'NONE', #86403, #41896, #18889 ) ;
#30836=CARTESIAN_POINT ( 'NONE',  ( -6.732636091893168029, -88.11213685669366669, 4.000000000000000000 ) ) ;
#30857=FACE_BOUND ( 'NONE', #91961, .T. ) ;
#30889=CARTESIAN_POINT ( 'NONE',  ( 6.575338752131433040, -50.90849809618014632, 3.750000000000000000 ) ) ;
#30891=FILL_AREA_STYLE ('',( #62867 ) ) ;
#30908=ORIENTED_EDGE ( 'NONE', *, *, #39884, .F. ) ;
#30930=EDGE_CURVE ( 'NONE', #92377, #19902, #94484, .T. ) ;
#30933=VECTOR ( 'NONE', #57916, 1000.000000000000000 ) ;
#30958=FACE_OUTER_BOUND ( 'NONE', #65546, .T. ) ;
#30963=EDGE_CURVE ( 'NONE', #82286, #40665, #41013, .T. ) ;
#30994=DIRECTION ( 'NONE',  ( -1.000000000000000000, 0.000000000000000000, -0.000000000000000000 ) ) ;
#31001=ORIENTED_EDGE ( 'NONE', *, *, #84512, .T. ) ;
#31008=MECHANICAL_DESIGN_GEOMETRIC_PRESENTATION_REPRESENTATION('',(#40649),#80544);
#31009=CARTESIAN_POINT ( 'NONE',  ( 6.879999999999995453, 43.00000000000000000, 4.250000000000000000 ) ) ;
#31050=FACE_OUTER_BOUND ( 'NONE', #15560, .T. ) ;
#31064=DIRECTION ( 'NONE',  ( 1.000000000000000000, 0.000000000000000000, 0.000000000000000000 ) ) ;
#31066=DIRECTION ( 'NONE',  ( 1.000000000000000000, 0.000000000000000000, 0.000000000000000000 ) ) ;
#31070=AXIS2_PLACEMENT_3D ( 'NONE', #19021, #80004, #65983 ) ;
#31078=CIRCLE ( 'NONE', #86973, 1.249999999999987121 ) ;
#31080=DIRECTION ( 'NONE',  ( 0.08715574274765140739, 0.9961946980917462113, 0.000000000000000000 ) ) ;
#31089=( NAMED_UNIT ( * ) PLANE_ANGLE_UNIT ( ) SI_UNIT ( $, .RADIAN. ) );
#31094=AXIS2_PLACEMENT_3D ( 'NONE', #96786, #73756, #81265 ) ;
#31111=UNCERTAINTY_MEASURE_WITH_UNIT (LENGTH_MEASURE( 1.000000000000000082E-05 ), #85113, 'distance_accuracy_value', 'NONE');
#31113=ORIENTED_EDGE ( 'NONE', *, *, #87848, .T. ) ;
#31114=EDGE_LOOP ( 'NONE', ( #63518, #24716, #90287, #43567 ) ) ;
#31119=CARTESIAN_POINT ( 'NONE',  ( -11.62817260217089199, -77.84151128241060746, 4.000000000000001776 ) ) ;
#31128=ADVANCED_FACE ( 'NONE', ( #41442 ), #11901, .F. ) ;
#31139=( NAMED_UNIT ( * ) SI_UNIT ( $, .STERADIAN. ) SOLID_ANGLE_UNIT ( ) );
#31146=ORIENTED_EDGE ( 'NONE', *, *, #26467, .T. ) ;
#31157=LINE ( 'NONE', #46182, #50488 ) ;
#31164=FACE_OUTER_BOUND ( 'NONE', #65184, .T. ) ;
#31167=PLANE ( 'NONE',  #97991 ) ;
#31170=CARTESIAN_POINT ( 'NONE',  ( -3.530007528296587704, -1.230351260576522110, 2.750000000000000000 ) ) ;
#31184=CARTESIAN_POINT ( 'NONE',  ( 5.679566525937524979, -28.64346213795363738, -2.750000000000000888 ) ) ;
#31226=CARTESIAN_POINT ( 'NONE',  ( -5.999999999999994671, 41.24999999999999289, 6.250000000000000000 ) ) ;
#31230=UNCERTAINTY_MEASURE_WITH_UNIT (LENGTH_MEASURE( 1.000000000000000082E-05 ), #91765, 'distance_accuracy_value', 'NONE');
#31234=AXIS2_PLACEMENT_3D ( 'NONE', #26647, #19644, #20636 ) ;
#31244=CARTESIAN_POINT ( 'NONE',  ( 18.00000000000000000, 77.37581971779007972, 4.190584158845563678 ) ) ;
#31247=CARTESIAN_POINT ( 'NONE',  ( -3.586264863366058098, -2.711807932106036212, 3.749999999999797939 ) ) ;
#31250=ORIENTED_EDGE ( 'NONE', *, *, #32879, .T. ) ;
#31258=FILL_AREA_STYLE ('',( #15793 ) ) ;
#31268=SURFACE_STYLE_FILL_AREA ( #76779 ) ;
#31275=VERTEX_POINT ( 'NONE', #94900 ) ;
#31277=LINE ( 'NONE', #61777, #34329 ) ;
#31281=( NAMED_UNIT ( * ) PLANE_ANGLE_UNIT ( ) SI_UNIT ( $, .RADIAN. ) );
#31285=VERTEX_POINT ( 'NONE', #48417 ) ;
#31292=CARTESIAN_POINT ( 'NONE',  ( -7.072466555035560098, -84.40185515922217974, -2.750000000000000000 ) ) ;
#31302=CARTESIAN_POINT ( 'NONE',  ( 4.380000000000000782, 0.09385850580201696158, -2.750000000000000000 ) ) ;
#31305=CARTESIAN_POINT ( 'NONE',  ( 6.757645195922957093, -58.31151720878640532, 2.750000000000000444 ) ) ;
#31315=CARTESIAN_POINT ( 'NONE',  ( 18.00000000000000355, 77.07179676972445748, -4.250000000000000000 ) ) ;
#31320=SURFACE_STYLE_USAGE ( .BOTH. , #83845 ) ;
#31323=CARTESIAN_POINT ( 'NONE',  ( -15.00000000000000000, 83.99999999999998579, 7.750000000000000000 ) ) ;
#31324=ORIENTED_EDGE ( 'NONE', *, *, #88395, .T. ) ;
#31327=SURFACE_STYLE_FILL_AREA ( #77319 ) ;
#31353=STYLED_ITEM ( 'NONE', ( #68790 ), #17764 ) ;
#31357=DIRECTION ( 'NONE',  ( 1.000000000000000000, 0.000000000000000000, 0.000000000000000000 ) ) ;
#31358=MECHANICAL_DESIGN_GEOMETRIC_PRESENTATION_REPRESENTATION('',(#33000),#48912);
#31371=EDGE_CURVE ( 'NONE', #55012, #31523, #39532, .T. ) ;
#31372=VECTOR ( 'NONE', #51958, 1000.000000000000114 ) ;
#31377=( LENGTH_UNIT ( ) NAMED_UNIT ( * ) SI_UNIT ( .MILLI., .METRE. ) );
#31381=CARTESIAN_POINT ( 'NONE',  ( -4.787136363774555647, -17.54594992866424974, -4.000000000000000000 ) ) ;
#31389=CARTESIAN_POINT ( 'NONE',  ( -7.750000000000000000, 40.74999999999999289, 3.750000000000000000 ) ) ;
#31392=EDGE_CURVE ( 'NONE', #33199, #87437, #77837, .T. ) ;
#31405=FILL_AREA_STYLE_COLOUR ( '', #84250 ) ;
#31417=AXIS2_PLACEMENT_3D ( 'NONE', #14222, #21728, #91188 ) ;
#31426=DIRECTION ( 'NONE',  ( 1.000000000000000000, -0.000000000000000000, -0.000000000000000000 ) ) ;
#31427=CARTESIAN_POINT ( 'NONE',  ( 4.130000000000000782, 1.019547802438464545, 2.500000000000000000 ) ) ;
#31443=VECTOR ( 'NONE', #18536, 1000.000000000000000 ) ;
#31460=CLOSED_SHELL ( 'NONE', ( #88095, #35899, #80504, #60408, #92137, #93951, #2542, #16519, #50908, #1544, #41186, #25541, #4539, #44265, #31520, #84439, #20796, #27198, #19319, #43564, #5885, #84507, #45129, #15530, #82972, #48485, #21724, #10088, #31849, #90071 ) ) ;
#31463=ORIENTED_EDGE ( 'NONE', *, *, #69537, .F. ) ;
#31472=CARTESIAN_POINT ( 'NONE',  ( 6.880000000000009663, 40.99999999999999289, -6.500000000000000888 ) ) ;
#31474=ORIENTED_EDGE ( 'NONE', *, *, #50023, .T. ) ;
#31494=CARTESIAN_POINT ( 'NONE',  ( -18.89999999999999503, 92.00000000000000000, 7.750000000000000000 ) ) ;
#31495=CARTESIAN_POINT ( 'NONE',  ( -10.31693093662791405, 89.21683745891327533, -5.695017665641882054 ) ) ;
#31500=EDGE_CURVE ( 'NONE', #43409, #42048, #74860, .T. ) ;
#31502=CARTESIAN_POINT ( 'NONE',  ( 10.58840669699852199, -98.14374106289703548, 4.000000000000000000 ) ) ;
#31518=VECTOR ( 'NONE', #73093, 1000.000000000000000 ) ;
#31520=ADVANCED_FACE ( 'NONE', ( #28378 ), #4899, .T. ) ;
#31523=VERTEX_POINT ( 'NONE', #67362 ) ;
#31528=ORIENTED_EDGE ( 'NONE', *, *, #81256, .F. ) ;
#31530=DIRECTION ( 'NONE',  ( 0.000000000000000000, -1.000000000000000000, -0.000000000000000000 ) ) ;
#31533=FILL_AREA_STYLE_COLOUR ( '', #36299 ) ;
#31541=DIRECTION ( 'NONE',  ( 0.000000000000000000, -1.000000000000000000, 0.000000000000000000 ) ) ;
#31542=TOROIDAL_SURFACE ( 'NONE', #92224, 3.750000000000001776, 0.2500000000000000000 ) ;
#31547=DIRECTION ( 'NONE',  ( 1.000000000000000000, 1.049065152435174162E-16, 0.000000000000000000 ) ) ;
#31568=CARTESIAN_POINT ( 'NONE',  ( -6.841090228438033272, -58.65898919720570603, -2.750000000000000444 ) ) ;
#31570=PRESENTATION_STYLE_ASSIGNMENT (( #92570 ) ) ;
#31576=LINE ( 'NONE', #8595, #77128 ) ;
#31580=DIRECTION ( 'NONE',  ( 1.000000000000000000, 1.257402221000611116E-16, -0.000000000000000000 ) ) ;
#31603=FILL_AREA_STYLE ('',( #93094 ) ) ;
#31605=EDGE_CURVE ( 'NONE', #11363, #95826, #10832, .T. ) ;
#31606=ORIENTED_EDGE ( 'NONE', *, *, #67066, .F. ) ;
#31607=ORIENTED_EDGE ( 'NONE', *, *, #16116, .F. ) ;
#31613=CARTESIAN_POINT ( 'NONE',  ( -9.793382739396090386, -28.00152668697614189, 3.750000000000000000 ) ) ;
#31623=ORIENTED_EDGE ( 'NONE', *, *, #90876, .F. ) ;
#31627=ORIENTED_EDGE ( 'NONE', *, *, #90184, .F. ) ;
#31634=CYLINDRICAL_SURFACE ( 'NONE', #40690, 0.2500000000000002220 ) ;
#31643=VECTOR ( 'NONE', #4598, 1000.000000000000000 ) ;
#31649=DIRECTION ( 'NONE',  ( -1.000000000000000000, 0.000000000000000000, 0.000000000000000000 ) ) ;
#31651=VECTOR ( 'NONE', #20301, 1000.000000000000000 ) ;
#31657=CARTESIAN_POINT ( 'NONE',  ( -4.010449548135202491, -13.83555390988819767, 2.500000000000001332 ) ) ;
#31659=CARTESIAN_POINT ( 'NONE',  ( 8.742110228303776154, -4.148858702909789642, 4.000000000000000000 ) ) ;
#31664=DIRECTION ( 'NONE',  ( 1.000000000000000000, 0.000000000000000000, -0.000000000000000000 ) ) ;
#31669=FACE_OUTER_BOUND ( 'NONE', #11997, .T. ) ;
#31675=DIRECTION ( 'NONE',  ( 1.000000000000000000, 0.000000000000000000, 0.000000000000000000 ) ) ;
#31695=EDGE_CURVE ( 'NONE', #54251, #51712, #61330, .T. ) ;
#31713=CARTESIAN_POINT ( 'NONE',  ( 8.630000000000000782, 1.019547802438459216, -4.000000000000000000 ) ) ;
#31723=VECTOR ( 'NONE', #55867, 1000.000000000000000 ) ;
#31744=CARTESIAN_POINT ( 'NONE',  ( -5.811454672275934819, -36.11427488548928011, 4.000000000000000000 ) ) ;
#31745=ORIENTED_EDGE ( 'NONE', *, *, #24698, .F. ) ;
#31750=VERTEX_POINT ( 'NONE', #85317 ) ;
#31754=DIRECTION ( 'NONE',  ( 0.000000000000000000, 0.000000000000000000, -1.000000000000000000 ) ) ;
#31770=EDGE_LOOP ( 'NONE', ( #31250, #21570, #30058, #28712 ) ) ;
#31771=CARTESIAN_POINT ( 'NONE',  ( 3.969999999999999751, 36.75000000000000000, 3.750000000000000000 ) ) ;
#31779=CARTESIAN_POINT ( 'NONE',  ( 5.679567480639522437, -28.64348288259103725, -3.750000000000000000 ) ) ;
#31790=STYLED_ITEM ( 'NONE', ( #60682 ), #72135 ) ;
#31792=CARTESIAN_POINT ( 'NONE',  ( -10.94840535726592634, 89.72140148746893829, 6.176821657850954495 ) ) ;
#31804=LINE ( 'NONE', #62302, #36126 ) ;
#31805=DIRECTION ( 'NONE',  ( 1.000000000000000000, 0.000000000000000000, 0.000000000000000000 ) ) ;
#31809=CARTESIAN_POINT ( 'NONE',  ( -9.793405416354234561, -28.00185549905096849, -3.750000000000000000 ) ) ;
#31825=ORIENTED_EDGE ( 'NONE', *, *, #13544, .F. ) ;
#31828=DIRECTION ( 'NONE',  ( 1.927470528863119542E-16, -1.000000000000000000, 0.000000000000000000 ) ) ;
#31849=ADVANCED_FACE ( 'NONE', ( #53335 ), #84829, .T. ) ;
#31855=ORIENTED_EDGE ( 'NONE', *, *, #49008, .T. ) ;
#31857=EDGE_LOOP ( 'NONE', ( #84626, #38571, #46009, #82078 ) ) ;
#31860=EDGE_LOOP ( 'NONE', ( #43758, #17158, #32781, #33393 ) ) ;
#31864=( NAMED_UNIT ( * ) SI_UNIT ( $, .STERADIAN. ) SOLID_ANGLE_UNIT ( ) );
#31876=CARTESIAN_POINT ( 'NONE',  ( 15.00000000000000178, 73.00000000000000000, -6.250000000000000000 ) ) ;
#31879=VECTOR ( 'NONE', #12339, 1000.000000000000000 ) ;
#31885=ORIENTED_EDGE ( 'NONE', *, *, #36631, .T. ) ;
#31905=FACE_OUTER_BOUND ( 'NONE', #6571, .T. ) ;
#31914=CARTESIAN_POINT ( 'NONE',  ( 4.526800700887880780, -5.190657137169758073, -3.750000000000000888 ) ) ;
#31916=CARTESIAN_POINT ( 'NONE',  ( 6.324684870385063995, -50.88968658577716297, 2.500000000000000888 ) ) ;
#31919=ORIENTED_EDGE ( 'NONE', *, *, #41296, .F. ) ;
#31929=ORIENTED_EDGE ( 'NONE', *, *, #95318, .T. ) ;
#31931=CARTESIAN_POINT ( 'NONE',  ( 9.779999999999994031, 1.885066177228129719E-15, 3.000000000000000000 ) ) ;
#31937=CARTESIAN_POINT ( 'NONE',  ( 4.721518086276724979, -3.620742741961517019, -4.000000000000000000 ) ) ;
#31947=AXIS2_PLACEMENT_3D ( 'NONE', #87850, #81822, #65340 ) ;
#31951=SPHERICAL_SURFACE ( 'NONE', #52919, 0.2500000000000000000 ) ;
#32001=COLOUR_RGB ( '', 0.72549020, 0.75294118, 0.79215686) ;
#32022=ORIENTED_EDGE ( 'NONE', *, *, #84873, .F. ) ;
#32028=FACE_OUTER_BOUND ( 'NONE', #62522, .T. ) ;
#32042=AXIS2_PLACEMENT_3D ( 'NONE', #22228, #36730, #7720 ) ;
#32045=EDGE_CURVE ( 'NONE', #8279, #23534, #34569, .T. ) ;
#32052=CARTESIAN_POINT ( 'NONE',  ( -7.127794346849581686, -80.93619716733994096, -3.750000000000000000 ) ) ;
#32062=DIRECTION ( 'NONE',  ( 1.000000000000000000, 0.000000000000000000, 0.000000000000000000 ) ) ;
#32063=CARTESIAN_POINT ( 'NONE',  ( -10.53011945866294852, -98.59345040283277228, 4.000000000000000000 ) ) ;
#32066=VECTOR ( 'NONE', #10082, 1000.000000000000000 ) ;
#32079=EDGE_CURVE ( 'NONE', #31750, #60629, #42795, .T. ) ;
#32081=CYLINDRICAL_SURFACE ( 'NONE', #71744, 0.2500000000000002220 ) ;
#32090=UNCERTAINTY_MEASURE_WITH_UNIT (LENGTH_MEASURE( 1.000000000000000082E-05 ), #71913, 'distance_accuracy_value', 'NONE');
#32092=VERTEX_POINT ( 'NONE', #15762 ) ;
#32093=VERTEX_POINT ( 'NONE', #98290 ) ;
#32109=SURFACE_STYLE_USAGE ( .BOTH. , #47626 ) ;
#32136=AXIS2_PLACEMENT_3D ( 'NONE', #74117, #28137, #12150 ) ;
#32137=ORIENTED_EDGE ( 'NONE', *, *, #23470, .T. ) ;
#32139=CARTESIAN_POINT ( 'NONE',  ( -4.259797195126484581, -13.81744876717395876, 2.750000000000000888 ) ) ;
#32141=DIRECTION ( 'NONE',  ( -0.06975647374410356982, -0.9975640502598257520, -0.000000000000000000 ) ) ;
#32145=COLOUR_RGB ( '', 0.66274510, 0.83137255, 0.94901961) ;
#32154=FACE_OUTER_BOUND ( 'NONE', #66799, .T. ) ;
#32164=EDGE_LOOP ( 'NONE', ( #43217, #83434, #50604, #77500 ) ) ;
#32170=CARTESIAN_POINT ( 'NONE',  ( 3.969999999999999751, 37.25000000000000000, 3.750000000000000000 ) ) ;
#32194=UNCERTAINTY_MEASURE_WITH_UNIT (LENGTH_MEASURE( 1.000000000000000082E-05 ), #66925, 'distance_accuracy_value', 'NONE');
#32208=CARTESIAN_POINT ( 'NONE',  ( -3.750000000000000000, 36.75000000000000000, -2.750000000000000000 ) ) ;
#32216=( LENGTH_UNIT ( ) NAMED_UNIT ( * ) SI_UNIT ( .MILLI., .METRE. ) );
#32228=CARTESIAN_POINT ( 'NONE',  ( 18.00000000000000000, 77.35022402048976176, 4.131279366366106487 ) ) ;
#32231=CARTESIAN_POINT ( 'NONE',  ( -4.139459722423826982, -8.271751626981549421, 4.000000000000000000 ) ) ;
#32232=ORIENTED_EDGE ( 'NONE', *, *, #63452, .F. ) ;
#32233=CARTESIAN_POINT ( 'NONE',  ( 10.83696084481538691, -98.17058944465519232, 4.000000000000000000 ) ) ;
#32259=ORIENTED_EDGE ( 'NONE', *, *, #32079, .T. ) ;
#32271=DIRECTION ( 'NONE',  ( -0.000000000000000000, 0.000000000000000000, 1.000000000000000000 ) ) ;
#32274=EDGE_CURVE ( 'NONE', #59804, #717, #47355, .T. ) ;
#32282=CARTESIAN_POINT ( 'NONE',  ( -7.750355510519348456, 84.07179676972448590, 4.000000000000000000 ) ) ;
#32291=AXIS2_PLACEMENT_3D ( 'NONE', #17624, #41610, #64561 ) ;
#32310=CARTESIAN_POINT ( 'NONE',  ( -9.343156623282764528, 88.41679554545851261, -5.273290232418045953 ) ) ;
#32321=DIRECTION ( 'NONE',  ( -0.000000000000000000, 1.000000000000000000, -0.000000000000000000 ) ) ;
#32330=SURFACE_STYLE_FILL_AREA ( #78328 ) ;
#32360=CARTESIAN_POINT ( 'NONE',  ( 1.350000000000004086, 98.49999999999998579, -8.525133428036873795 ) ) ;
#32364=AXIS2_PLACEMENT_3D ( 'NONE', #98226, #75697, #7208 ) ;
#32371=( GEOMETRIC_REPRESENTATION_CONTEXT ( 3 ) GLOBAL_UNCERTAINTY_ASSIGNED_CONTEXT ( ( #17126 ) ) GLOBAL_UNIT_ASSIGNED_CONTEXT ( ( #1365, #71317, #3806 ) ) REPRESENTATION_CONTEXT ( 'NONE', 'WORKASPACE' ) );
#32382=VERTEX_POINT ( 'NONE', #17382 ) ;
#32392=( LENGTH_UNIT ( ) NAMED_UNIT ( * ) SI_UNIT ( .MILLI., .METRE. ) );
#32398=FACE_BOUND ( 'NONE', #16560, .T. ) ;
#32400=ORIENTED_EDGE ( 'NONE', *, *, #32680, .T. ) ;
#32402=AXIS2_PLACEMENT_3D ( 'NONE', #68811, #54275, #62266 ) ;
#32403=DIRECTION ( 'NONE',  ( -1.000000000000000000, 0.000000000000000000, 0.000000000000000000 ) ) ;
#32420=CARTESIAN_POINT ( 'NONE',  ( 4.919406150738182326, -13.80316667506059858, 2.500000000000000000 ) ) ;
#32422=ORIENTED_EDGE ( 'NONE', *, *, #49008, .F. ) ;
#32433=EDGE_CURVE ( 'NONE', #75573, #95619, #86851, .T. ) ;
#32435=FILL_AREA_STYLE_COLOUR ( '', #54640 ) ;
#32440=CARTESIAN_POINT ( 'NONE',  ( 18.00000000000000355, 77.07179676972445748, 4.250000000000000000 ) ) ;
#32442=COLOUR_RGB ( '', 0.09019608, 0.27058824, 0.51372549) ;
#32445=CYLINDRICAL_SURFACE ( 'NONE', #5604, 0.09999999999999939493 ) ;
#32465=DIRECTION ( 'NONE',  ( -0.000000000000000000, -0.000000000000000000, -1.000000000000000000 ) ) ;
#32469=SURFACE_STYLE_USAGE ( .BOTH. , #77972 ) ;
#32530=ORIENTED_EDGE ( 'NONE', *, *, #45564, .F. ) ;
#32544=CARTESIAN_POINT ( 'NONE',  ( -0.000000000000000000, 91.25000000000000000, -7.750000000000000000 ) ) ;
#32556=DIRECTION ( 'NONE',  ( 0.000000000000000000, 0.000000000000000000, 1.000000000000000000 ) ) ;
#32566=DIRECTION ( 'NONE',  ( 0.000000000000000000, 0.000000000000000000, -1.000000000000000000 ) ) ;
#32569=CARTESIAN_POINT ( 'NONE',  ( 0.000000000000000000, 69.99999999999998579, 4.000000000000000000 ) ) ;
#32573=SURFACE_STYLE_FILL_AREA ( #48557 ) ;
#32574=STYLED_ITEM ( 'NONE', ( #81170 ), #97716 ) ;
#32578=CARTESIAN_POINT ( 'NONE',  ( 0.000000000000000000, -97.00000000000000000, -2.500000000000000000 ) ) ;
#32584=STYLED_ITEM ( 'NONE', ( #22241 ), #94194 ) ;
#32592=SURFACE_STYLE_USAGE ( .BOTH. , #23145 ) ;
#32594=DIRECTION ( 'NONE',  ( -0.000000000000000000, -0.000000000000000000, -1.000000000000000000 ) ) ;
#32596=ORIENTED_EDGE ( 'NONE', *, *, #51630, .T. ) ;
#32620=DIRECTION ( 'NONE',  ( 1.000000000000000000, -0.000000000000000000, -0.000000000000000000 ) ) ;
#32637=DIRECTION ( 'NONE',  ( -0.000000000000000000, 1.000000000000000000, 0.000000000000000000 ) ) ;
#32643=FACE_OUTER_BOUND ( 'NONE', #34584, .T. ) ;
#32652=DIRECTION ( 'NONE',  ( 1.000000000000000000, 0.000000000000000000, 0.000000000000000000 ) ) ;
#32680=EDGE_CURVE ( 'NONE', #49491, #6552, #80106, .T. ) ;
#32704=SURFACE_SIDE_STYLE ('',( #77717 ) ) ;
#32721=DIRECTION ( 'NONE',  ( 0.000000000000000000, 0.000000000000000000, -1.000000000000000000 ) ) ;
#32726=CARTESIAN_POINT ( 'NONE',  ( -6.060988839905887993, -36.09899559455953977, 4.000000000000000000 ) ) ;
#32731=VERTEX_POINT ( 'NONE', #66834 ) ;
#32740=MECHANICAL_DESIGN_GEOMETRIC_PRESENTATION_REPRESENTATION('',(#71083),#40750);
#32744=ORIENTED_EDGE ( 'NONE', *, *, #82988, .T. ) ;
#32746=ORIENTED_EDGE ( 'NONE', *, *, #9727, .F. ) ;
#32749=DIRECTION ( 'NONE',  ( 1.000000000000000000, 0.000000000000000000, 0.000000000000000000 ) ) ;
#32751=AXIS2_PLACEMENT_3D ( 'NONE', #4890, #5868, #87872 ) ;
#32758=FILL_AREA_STYLE_COLOUR ( '', #90822 ) ;
#32781=ORIENTED_EDGE ( 'NONE', *, *, #80448, .F. ) ;
#32783=CYLINDRICAL_SURFACE ( 'NONE', #36131, 0.2500000000000002220 ) ;
#32791=CARTESIAN_POINT ( 'NONE',  ( -6.000000000000009770, 40.99999999999999289, 4.250000000000000000 ) ) ;
#32792=CARTESIAN_POINT ( 'NONE',  ( -3.750000000000000000, 10.25000000000000000, -3.750000000000000000 ) ) ;
#32802=CARTESIAN_POINT ( 'NONE',  ( -8.000343251535921851, 84.06932101904432386, -3.750000000000000000 ) ) ;
#32815=DIRECTION ( 'NONE',  ( 0.000000000000000000, 0.000000000000000000, -1.000000000000000000 ) ) ;
#32820=PRESENTATION_STYLE_ASSIGNMENT (( #92843 ) ) ;
#32831=CARTESIAN_POINT ( 'NONE',  ( -8.000000000000000000, 80.07179676972448590, -6.250000000000000000 ) ) ;
#32841=VERTEX_POINT ( 'NONE', #91812 ) ;
#32843=EDGE_CURVE ( 'NONE', #74689, #18880, #64106, .T. ) ;
#32845=ORIENTED_EDGE ( 'NONE', *, *, #7294, .F. ) ;
#32860=EDGE_CURVE ( 'NONE', #21688, #54112, #85445, .T. ) ;
#32870=FACE_OUTER_BOUND ( 'NONE', #60055, .T. ) ;
#32873=TOROIDAL_SURFACE ( 'NONE', #12107, 2.899999999999999467, 0.1000000000000000056 ) ;
#32875=CARTESIAN_POINT ( 'NONE',  ( 9.879999999999990123, 20.99999999999999645, -2.899999999999999911 ) ) ;
#32879=EDGE_CURVE ( 'NONE', #16289, #40665, #9790, .T. ) ;
#32881=ORIENTED_EDGE ( 'NONE', *, *, #47002, .T. ) ;
#32889=DIRECTION ( 'NONE',  ( 0.000000000000000000, 0.000000000000000000, 1.000000000000000000 ) ) ;
#32911=CARTESIAN_POINT ( 'NONE',  ( 6.905507196100984402, -69.44000359832136837, 2.499999999998390621 ) ) ;
#32913=AXIS2_PLACEMENT_3D ( 'NONE', #16824, #70325, #24826 ) ;
#32923=CIRCLE ( 'NONE', #10595, 0.2500000000000002220 ) ;
#32924=COLOUR_RGB ( '', 0.08235294, 0.09019608, 0.10196078) ;
#32927=AXIS2_PLACEMENT_3D ( 'NONE', #29677, #22209, #52686 ) ;
#32939=CARTESIAN_POINT ( 'NONE',  ( -8.000000000000000000, 79.82179676972448590, -6.250000000000000000 ) ) ;
#32942=ORIENTED_EDGE ( 'NONE', *, *, #21654, .T. ) ;
#32947=DIRECTION ( 'NONE',  ( -0.000000000000000000, -0.000000000000000000, 1.000000000000000000 ) ) ;
#32964=ORIENTED_EDGE ( 'NONE', *, *, #12999, .T. ) ;
#32968=DIRECTION ( 'NONE',  ( 1.000000000000000000, 0.000000000000000000, -0.000000000000000000 ) ) ;
#32982=AXIS2_PLACEMENT_3D ( 'NONE', #49951, #80455, #95958 ) ;
#32983=CARTESIAN_POINT ( 'NONE',  ( -9.795294835246881604, -28.02932231004771069, -3.750000000000001332 ) ) ;
#33000=STYLED_ITEM ( 'NONE', ( #35595 ), #87902 ) ;
#33005=EDGE_CURVE ( 'NONE', #69773, #55108, #33261, .T. ) ;
#33011=PLANE ( 'NONE',  #2785 ) ;
#33016=AXIS2_PLACEMENT_3D ( 'NONE', #51541, #81047, #51041 ) ;
#33035=DIRECTION ( 'NONE',  ( 0.000000000000000000, 4.683753385137383573E-14, -1.000000000000000000 ) ) ;
#33041=VECTOR ( 'NONE', #53011, 1000.000000000000000 ) ;
#33053=DIRECTION ( 'NONE',  ( 0.8070303256584298035, -0.5905099943842175847, 0.000000000000000000 ) ) ;
#33057=CARTESIAN_POINT ( 'NONE',  ( -10.32520421619553197, -40.46224970676419019, 4.000000000000000888 ) ) ;
#33062=CARTESIAN_POINT ( 'NONE',  ( -8.124115902427741176, 75.04369783535875627, -3.000000000000000000 ) ) ;
#33063=FACE_OUTER_BOUND ( 'NONE', #64213, .T. ) ;
#33083=AXIS2_PLACEMENT_3D ( 'NONE', #68212, #72849, #45199 ) ;
#33102=ORIENTED_EDGE ( 'NONE', *, *, #92517, .T. ) ;
#33110=DIRECTION ( 'NONE',  ( 2.569960705150826877E-16, -1.000000000000000000, 0.000000000000000000 ) ) ;
#33118=ORIENTED_EDGE ( 'NONE', *, *, #17170, .F. ) ;
#33127=VECTOR ( 'NONE', #37769, 999.9999999999998863 ) ;
#33129=VERTEX_POINT ( 'NONE', #33737 ) ;
#33133=CARTESIAN_POINT ( 'NONE',  ( -8.000000000000000000, 79.82179676972448590, 4.000000000000000000 ) ) ;
#33134=AXIS2_PLACEMENT_3D ( 'NONE', #59169, #45154, #37673 ) ;
#33142=VECTOR ( 'NONE', #27876, 1000.000000000000000 ) ;
#33143=CARTESIAN_POINT ( 'NONE',  ( 4.219999999999999751, 10.00000000000000000, -2.500000000000000000 ) ) ;
#33147=DIRECTION ( 'NONE',  ( 0.000000000000000000, 0.000000000000000000, -1.000000000000000000 ) ) ;
#33150=CARTESIAN_POINT ( 'NONE',  ( 4.395797040798766098, -0.8371465525189527579, -2.750000000000000444 ) ) ;
#33156=DIRECTION ( 'NONE',  ( 1.000000000000000000, -0.000000000000000000, -0.000000000000000000 ) ) ;
#33176=ORIENTED_EDGE ( 'NONE', *, *, #43035, .F. ) ;
#33181=DIRECTION ( 'NONE',  ( 1.000000000000000000, 0.000000000000000000, 0.000000000000000000 ) ) ;
#33183=UNCERTAINTY_MEASURE_WITH_UNIT (LENGTH_MEASURE( 1.000000000000000082E-05 ), #3816, 'distance_accuracy_value', 'NONE');
#33197=AXIS2_PLACEMENT_3D ( 'NONE', #7046, #8520, #77993 ) ;
#33199=VERTEX_POINT ( 'NONE', #64239 ) ;
#33200=ORIENTED_EDGE ( 'NONE', *, *, #47745, .T. ) ;
#33208=FACE_OUTER_BOUND ( 'NONE', #83051, .T. ) ;
#33214=CARTESIAN_POINT ( 'NONE',  ( 17.75000000000000000, 78.80384757729336798, 4.000000000000000000 ) ) ;
#33219=CARTESIAN_POINT ( 'NONE',  ( -7.117921737454939723, -58.38558715620312256, 4.000000000000000888 ) ) ;
#33227=CIRCLE ( 'NONE', #89111, 2.250000000000001332 ) ;
#33230=AXIS2_PLACEMENT_3D ( 'NONE', #52653, #81665, #5693 ) ;
#33234=ORIENTED_EDGE ( 'NONE', *, *, #11281, .F. ) ;
#33237=ORIENTED_EDGE ( 'NONE', *, *, #43586, .F. ) ;
#33242=CARTESIAN_POINT ( 'NONE',  ( 0.4400000000000020006, 1.019547802438468986, 3.750000000000000000 ) ) ;
#33244=ADVANCED_FACE ( 'NONE', ( #49734 ), #40784, .F. ) ;
#33246=PRESENTATION_STYLE_ASSIGNMENT (( #26246 ) ) ;
#33260=PRESENTATION_STYLE_ASSIGNMENT (( #48264 ) ) ;
#33261=LINE ( 'NONE', #49257, #33625 ) ;
#33267=DIRECTION ( 'NONE',  ( -1.483861936729427615E-16, 1.000000000000000000, 0.000000000000000000 ) ) ;
#33275=( GEOMETRIC_REPRESENTATION_CONTEXT ( 3 ) GLOBAL_UNCERTAINTY_ASSIGNED_CONTEXT ( ( #97169 ) ) GLOBAL_UNIT_ASSIGNED_CONTEXT ( ( #12114, #96620, #89099 ) ) REPRESENTATION_CONTEXT ( 'NONE', 'WORKASPACE' ) );
#33277=CARTESIAN_POINT ( 'NONE',  ( 4.879999999999994564, 43.00000000000000711, -6.250000000000000000 ) ) ;
#33299=ORIENTED_EDGE ( 'NONE', *, *, #18233, .F. ) ;
#33300=( LENGTH_UNIT ( ) NAMED_UNIT ( * ) SI_UNIT ( .MILLI., .METRE. ) );
#33309=DIRECTION ( 'NONE',  ( 0.000000000000000000, 0.000000000000000000, -1.000000000000000000 ) ) ;
#33313=UNCERTAINTY_MEASURE_WITH_UNIT (LENGTH_MEASURE( 1.000000000000000082E-05 ), #81747, 'distance_accuracy_value', 'NONE');
#33335=EDGE_LOOP ( 'NONE', ( #94593, #47255, #8000, #90030 ) ) ;
#33338=CARTESIAN_POINT ( 'NONE',  ( 0.000000000000000000, -97.00000000000000000, 3.750000000000000000 ) ) ;
#33348=ORIENTED_EDGE ( 'NONE', *, *, #5334, .T. ) ;
#33349=DIRECTION ( 'NONE',  ( 1.000000000000000000, 0.000000000000000000, 0.000000000000000000 ) ) ;
#33370=CARTESIAN_POINT ( 'NONE',  ( -7.750000000000000000, 80.32179676972448590, 4.250000000000000000 ) ) ;
#33372=CIRCLE ( 'NONE', #22208, 10.90000000000026326 ) ;
#33374=FILL_AREA_STYLE_COLOUR ( '', #23414 ) ;
#33393=ORIENTED_EDGE ( 'NONE', *, *, #88589, .F. ) ;
#33395=DIRECTION ( 'NONE',  ( 1.000000000000000000, 0.000000000000000000, 0.000000000000000000 ) ) ;
#33397=DIRECTION ( 'NONE',  ( 0.7808688094430307203, -0.6246950475544238435, 0.000000000000000000 ) ) ;
#33401=ADVANCED_FACE ( 'NONE', ( #43224 ), #91173, .T. ) ;
#33402=ORIENTED_EDGE ( 'NONE', *, *, #42395, .T. ) ;
#33406=DIRECTION ( 'NONE',  ( 1.000000000000000000, -0.000000000000000000, -0.000000000000000000 ) ) ;
#33407=CARTESIAN_POINT ( 'NONE',  ( -3.521809514228322335, -0.8352226969046322447, -2.499999999999393818 ) ) ;
#33410=CYLINDRICAL_SURFACE ( 'NONE', #25728, 8.000000000000000000 ) ;
#33413=DIRECTION ( 'NONE',  ( 1.000000000000000000, 0.000000000000000000, 0.000000000000000000 ) ) ;
#33416=CARTESIAN_POINT ( 'NONE',  ( -19.64999999999999858, 92.00000000000000000, 7.750000000000000000 ) ) ;
#33423=ORIENTED_EDGE ( 'NONE', *, *, #43684, .T. ) ;
#33424=ADVANCED_FACE ( 'NONE', ( #41184 ), #48129, .F. ) ;
#33436=SURFACE_STYLE_USAGE ( .BOTH. , #39983 ) ;
#33442=AXIS2_PLACEMENT_3D ( 'NONE', #19419, #49911, #95924 ) ;
#33448=AXIS2_PLACEMENT_3D ( 'NONE', #64430, #92969, #48457 ) ;
#33451=ORIENTED_EDGE ( 'NONE', *, *, #80392, .F. ) ;
#33456=DIRECTION ( 'NONE',  ( 1.927470528863119295E-16, -1.000000000000000000, 0.000000000000000000 ) ) ;
#33461=CARTESIAN_POINT ( 'NONE',  ( -11.62814856721715095, -77.87341909757282110, -3.750000000000000000 ) ) ;
#33476=CIRCLE ( 'NONE', #28702, 0.2500000000000002220 ) ;
#33481=VERTEX_POINT ( 'NONE', #41674 ) ;
#33499=DIRECTION ( 'NONE',  ( -8.673617379884026597E-16, -1.000000000000000000, 7.806255641895624036E-15 ) ) ;
#33501=UNCERTAINTY_MEASURE_WITH_UNIT (LENGTH_MEASURE( 1.000000000000000082E-05 ), #22022, 'distance_accuracy_value', 'NONE');
#33508=( NAMED_UNIT ( * ) SI_UNIT ( $, .STERADIAN. ) SOLID_ANGLE_UNIT ( ) );
#33509=ORIENTED_EDGE ( 'NONE', *, *, #599, .F. ) ;
#33522=EDGE_CURVE ( 'NONE', #31275, #95619, #35349, .T. ) ;
#33533=CARTESIAN_POINT ( 'NONE',  ( -6.732636091893172470, -88.11213685669366669, -3.750000000000000000 ) ) ;
#33534=CIRCLE ( 'NONE', #89442, 4.000000000000001776 ) ;
#33558=ADVANCED_FACE ( 'NONE', ( #89617, #37124, #51628, #66115 ), #96644, .F. ) ;
#33566=DIRECTION ( 'NONE',  ( -1.257402221000611116E-16, 1.000000000000000000, 0.000000000000000000 ) ) ;
#33568=STYLED_ITEM ( 'NONE', ( #774 ), #66500 ) ;
#33569=ORIENTED_EDGE ( 'NONE', *, *, #7958, .F. ) ;
#33580=SURFACE_STYLE_FILL_AREA ( #26582 ) ;
#33584=DIRECTION ( 'NONE',  ( 1.000000000000000000, 0.000000000000000000, 0.000000000000000000 ) ) ;
#33593=SURFACE_STYLE_FILL_AREA ( #3618 ) ;
#33599=ORIENTED_EDGE ( 'NONE', *, *, #30772, .F. ) ;
#33607=AXIS2_PLACEMENT_3D ( 'NONE', #93059, #61087, #77076 ) ;
#33608=EDGE_CURVE ( 'NONE', #65098, #82021, #37618, .T. ) ;
#33612=CARTESIAN_POINT ( 'NONE',  ( -5.559677335904731343, -36.09286816789840202, 2.500000000000000888 ) ) ;
#33614=CARTESIAN_POINT ( 'NONE',  ( 11.44533298129242738, -77.48611261198139744, 3.750000000000000000 ) ) ;
#33617=CARTESIAN_POINT ( 'NONE',  ( 4.219999999999999751, 36.75000000000000000, 2.500000000000000000 ) ) ;
#33618=CARTESIAN_POINT ( 'NONE',  ( -3.750000000000000000, 10.25000000000000000, 2.750000000000000000 ) ) ;
#33621=CARTESIAN_POINT ( 'NONE',  ( 11.34661744925197624, 54.08985607419764818, 0.000000000000000000 ) ) ;
#33623=DIRECTION ( 'NONE',  ( -0.000000000000000000, 0.000000000000000000, 1.000000000000000000 ) ) ;
#33625=VECTOR ( 'NONE', #87248, 1000.000000000000000 ) ;
#33642=CYLINDRICAL_SURFACE ( 'NONE', #13388, 0.2500000000000002220 ) ;
#33643=CIRCLE ( 'NONE', #94334, 0.2499999999999973910 ) ;
#33649=CARTESIAN_POINT ( 'NONE',  ( -8.957305892888854260, -19.72688805319553751, -4.000000000000000000 ) ) ;
#33651=DIRECTION ( 'NONE',  ( 1.000000000000000000, 0.000000000000000000, 0.000000000000000000 ) ) ;
#33664=LINE ( 'NONE', #64160, #35971 ) ;
#33670=CARTESIAN_POINT ( 'NONE',  ( 4.380000000000000782, -0.01592157648205478476, 3.750000000000001776 ) ) ;
#33678=AXIS2_PLACEMENT_3D ( 'NONE', #31323, #92816, #47804 ) ;
#33699=CARTESIAN_POINT ( 'NONE',  ( -7.366168427725257040, -80.69295184796105502, 4.000000000000000000 ) ) ;
#33701=CARTESIAN_POINT ( 'NONE',  ( -7.750000000000000000, 79.82179676972448590, -6.250000000000000000 ) ) ;
#33703=COLOUR_RGB ( '', 0.08235294, 0.09019608, 0.10196078) ;
#33710=TOROIDAL_SURFACE ( 'NONE', #19381, 6.599999999999995204, 0.2500000000000000000 ) ;
#33715=( GEOMETRIC_REPRESENTATION_CONTEXT ( 3 ) GLOBAL_UNCERTAINTY_ASSIGNED_CONTEXT ( ( #98417 ) ) GLOBAL_UNIT_ASSIGNED_CONTEXT ( ( #12541, #65026, #64538 ) ) REPRESENTATION_CONTEXT ( 'NONE', 'WORKASPACE' ) );
#33737=CARTESIAN_POINT ( 'NONE',  ( -14.89999999999998970, 98.50000000000000000, -8.000000000000000000 ) ) ;
#33746=DIRECTION ( 'NONE',  ( -1.000000000000000000, -0.000000000000000000, -0.000000000000000000 ) ) ;
#33748=ADVANCED_FACE ( 'NONE', ( #29104 ), #96905, .T. ) ;
#33758=DIRECTION ( 'NONE',  ( 0.6246950475544238435, 0.7808688094430307203, 0.000000000000000000 ) ) ;
#33763=CARTESIAN_POINT ( 'NONE',  ( -5.069238524696924486, -24.95996629666330335, 2.750000000000002220 ) ) ;
#33768=SURFACE_STYLE_USAGE ( .BOTH. , #49287 ) ;
#33776=CARTESIAN_POINT ( 'NONE',  ( -4.000000000000000000, 36.75000000000000000, -2.750000000000000000 ) ) ;
#33784=CARTESIAN_POINT ( 'NONE',  ( -3.750000000000000000, 36.75000000000000000, -2.500000000000000000 ) ) ;
#33788=FACE_OUTER_BOUND ( 'NONE', #86240, .T. ) ;
#33790=SURFACE_STYLE_USAGE ( .BOTH. , #80796 ) ;
#33806=ADVANCED_FACE ( 'NONE', ( #69585 ), #23611, .T. ) ;
#33815=ORIENTED_EDGE ( 'NONE', *, *, #14605, .T. ) ;
#33819=DIRECTION ( 'NONE',  ( -0.000000000000000000, 0.000000000000000000, 1.000000000000000000 ) ) ;
#33820=DIRECTION ( 'NONE',  ( 1.000000000000000000, -0.000000000000000000, 0.000000000000000000 ) ) ;
#33828=VERTEX_POINT ( 'NONE', #24592 ) ;
#33837=EDGE_CURVE ( 'NONE', #55756, #71742, #86385, .T. ) ;
#33845=TOROIDAL_SURFACE ( 'NONE', #89748, 2.900000000000001243, 0.1000000000000000056 ) ;
#33854=DIRECTION ( 'NONE',  ( 0.000000000000000000, 0.000000000000000000, 1.000000000000000000 ) ) ;
#33863=( NAMED_UNIT ( * ) SI_UNIT ( $, .STERADIAN. ) SOLID_ANGLE_UNIT ( ) );
#33870=ORIENTED_EDGE ( 'NONE', *, *, #42565, .T. ) ;
#33881=ORIENTED_EDGE ( 'NONE', *, *, #5580, .F. ) ;
#33883=CARTESIAN_POINT ( 'NONE',  ( 8.900383361500256996, -1.049454312711732840, 3.750000000000000000 ) ) ;
#33890=EDGE_LOOP ( 'NONE', ( #93096, #16778, #18205, #57808 ) ) ;
#33893=CARTESIAN_POINT ( 'NONE',  ( -3.585386599742077962, -2.690194976740517330, -2.750000000000402789 ) ) ;
#33899=CARTESIAN_POINT ( 'NONE',  ( 5.115475850186006923, -17.53855045867880591, -3.750000000001609823 ) ) ;
#33901=DIRECTION ( 'NONE',  ( 0.000000000000000000, 0.000000000000000000, 1.000000000000000000 ) ) ;
#33904=DIRECTION ( 'NONE',  ( 0.000000000000000000, -1.000000000000000000, 0.000000000000000000 ) ) ;
#33914=AXIS2_PLACEMENT_3D ( 'NONE', #41463, #94923, #34908 ) ;
#33928=COLOUR_RGB ( '', 0.09019608, 0.27058824, 0.51372549) ;
#33948=( LENGTH_UNIT ( ) NAMED_UNIT ( * ) SI_UNIT ( .MILLI., .METRE. ) );
#33950=EDGE_CURVE ( 'NONE', #52793, #49695, #36844, .T. ) ;
#33967=ORIENTED_EDGE ( 'NONE', *, *, #39973, .T. ) ;
#33970=EDGE_LOOP ( 'NONE', ( #13195, #40141, #23444, #4983 ) ) ;
#33981=AXIS2_PLACEMENT_3D ( 'NONE', #94806, #43280, #73775 ) ;
#33985=EDGE_CURVE ( 'NONE', #61040, #86598, #15120, .T. ) ;
#33987=DIRECTION ( 'NONE',  ( -0.000000000000000000, 0.000000000000000000, 1.000000000000000000 ) ) ;
#33990=AXIS2_PLACEMENT_3D ( 'NONE', #86157, #1690, #62646 ) ;
#33992=CARTESIAN_POINT ( 'NONE',  ( 14.49999999999999822, 75.00000000000000000, -8.525133428036872019 ) ) ;
#33994=VECTOR ( 'NONE', #61095, 1000.000000000000000 ) ;
#34001=EDGE_LOOP ( 'NONE', ( #27264, #62923, #48456, #40857 ) ) ;
#34003=( GEOMETRIC_REPRESENTATION_CONTEXT ( 3 ) GLOBAL_UNCERTAINTY_ASSIGNED_CONTEXT ( ( #14268 ) ) GLOBAL_UNIT_ASSIGNED_CONTEXT ( ( #6832, #45319, #30802 ) ) REPRESENTATION_CONTEXT ( 'NONE', 'WORKASPACE' ) );
#34022=CARTESIAN_POINT ( 'NONE',  ( -12.94148294176548930, 90.75484370785778765, 7.596443435273323885 ) ) ;
#34034=CIRCLE ( 'NONE', #3745, 0.2500000000000002220 ) ;
#34053=CARTESIAN_POINT ( 'NONE',  ( -6.000000000000007994, 41.24999999999999289, 6.250000000000000000 ) ) ;
#34056=DIRECTION ( 'NONE',  ( 0.9997628902338883128, -0.02177529129959722073, 0.000000000000000000 ) ) ;
#34057=CARTESIAN_POINT ( 'NONE',  ( -55.15243902439023316, 44.12195121951212684, -8.000000000000000000 ) ) ;
#34065=COLOUR_RGB ( '', 0.09019608, 0.27058824, 0.51372549) ;
#34076=FACE_OUTER_BOUND ( 'NONE', #62763, .T. ) ;
#34079=CARTESIAN_POINT ( 'NONE',  ( 3.969999999999999751, 10.25000000000000000, 3.750000000000000000 ) ) ;
#34080=EDGE_CURVE ( 'NONE', #3379, #36801, #70401, .T. ) ;
#34087=( NAMED_UNIT ( * ) SI_UNIT ( $, .STERADIAN. ) SOLID_ANGLE_UNIT ( ) );
#34088=CARTESIAN_POINT ( 'NONE',  ( 9.838578643762659226, 27.00180849546941175, -3.000000000000000888 ) ) ;
#34100=FACE_OUTER_BOUND ( 'NONE', #19364, .T. ) ;
#34102=DIRECTION ( 'NONE',  ( 0.000000000000000000, -1.000000000000000000, 0.000000000000000000 ) ) ;
#34105=CARTESIAN_POINT ( 'NONE',  ( 10.85666693321173071, -52.68303261953400352, 4.000000000000000000 ) ) ;
#34114=FILL_AREA_STYLE ('',( #49134 ) ) ;
#34127=ORIENTED_EDGE ( 'NONE', *, *, #36268, .T. ) ;
#34133=DIRECTION ( 'NONE',  ( 0.000000000000000000, 0.000000000000000000, 1.000000000000000000 ) ) ;
#34140=CARTESIAN_POINT ( 'NONE',  ( -11.42353084958745590, -90.30959216423875091, -3.750000000000000000 ) ) ;
#34154=UNCERTAINTY_MEASURE_WITH_UNIT (LENGTH_MEASURE( 1.000000000000000082E-05 ), #53786, 'distance_accuracy_value', 'NONE');
#34161=CARTESIAN_POINT ( 'NONE',  ( 4.526800700887880780, -5.190657137169758073, 2.750000000000000000 ) ) ;
#34175=ORIENTED_EDGE ( 'NONE', *, *, #52775, .F. ) ;
#34208=EDGE_CURVE ( 'NONE', #73831, #16571, #10366, .T. ) ;
#34209=ORIENTED_EDGE ( 'NONE', *, *, #44488, .F. ) ;
#34240=DIRECTION ( 'NONE',  ( -1.000000000000000000, -2.107602052970794797E-16, 0.000000000000000000 ) ) ;
#34253=CARTESIAN_POINT ( 'NONE',  ( 6.034179729230694456, -36.06068107361731023, 3.750000000000000888 ) ) ;
#34257=CARTESIAN_POINT ( 'NONE',  ( 15.55000000000000071, 99.99999999999998579, -8.525133428036873795 ) ) ;
#34259=( GEOMETRIC_REPRESENTATION_CONTEXT ( 3 ) GLOBAL_UNCERTAINTY_ASSIGNED_CONTEXT ( ( #19502 ) ) GLOBAL_UNIT_ASSIGNED_CONTEXT ( ( #89351, #81836, #97365 ) ) REPRESENTATION_CONTEXT ( 'NONE', 'WORKASPACE' ) );
#34263=( NAMED_UNIT ( * ) SI_UNIT ( $, .STERADIAN. ) SOLID_ANGLE_UNIT ( ) );
#34271=( GEOMETRIC_REPRESENTATION_CONTEXT ( 3 ) GLOBAL_UNCERTAINTY_ASSIGNED_CONTEXT ( ( #56523 ) ) GLOBAL_UNIT_ASSIGNED_CONTEXT ( ( #17464, #24968, #8473 ) ) REPRESENTATION_CONTEXT ( 'NONE', 'WORKASPACE' ) );
#34277=CARTESIAN_POINT ( 'NONE',  ( 14.99999999999998046, 69.99999999999998579, 4.000000000000000000 ) ) ;
#34279=SURFACE_STYLE_USAGE ( .BOTH. , #66774 ) ;
#34284=EDGE_CURVE ( 'NONE', #25669, #58411, #48046, .T. ) ;
#34296=CYLINDRICAL_SURFACE ( 'NONE', #18373, 0.2500000000000002220 ) ;
#34304=ORIENTED_EDGE ( 'NONE', *, *, #40653, .F. ) ;
#34314=ADVANCED_FACE ( 'NONE', ( #13879 ), #24149, .T. ) ;
#34316=CARTESIAN_POINT ( 'NONE',  ( 0.000000000000000000, -97.00000000000000000, 4.000000000000000000 ) ) ;
#34321=EDGE_CURVE ( 'NONE', #79527, #17231, #28899, .T. ) ;
#34324=EDGE_LOOP ( 'NONE', ( #30289, #72320, #51081, #20442, #39287, #54113 ) ) ;
#34329=VECTOR ( 'NONE', #23811, 1000.000000000000000 ) ;
#34334=CARTESIAN_POINT ( 'NONE',  ( 6.879999999999995453, 70.25000000000000000, -6.500000000000000888 ) ) ;
#34342=AXIS2_PLACEMENT_3D ( 'NONE', #37350, #74829, #27847 ) ;
#34356=CARTESIAN_POINT ( 'NONE',  ( 1.379999999999981908, 20.99999999999999645, 0.000000000000000000 ) ) ;
#34357=LINE ( 'NONE', #55905, #88367 ) ;
#34364=FACE_OUTER_BOUND ( 'NONE', #36612, .T. ) ;
#34366=CIRCLE ( 'NONE', #47144, 0.2499999999999997224 ) ;
#34368=SURFACE_STYLE_FILL_AREA ( #13354 ) ;
#34378=CARTESIAN_POINT ( 'NONE',  ( 5.129999999999990123, 76.07179676972444327, -6.250000000000000000 ) ) ;
#34388=ORIENTED_EDGE ( 'NONE', *, *, #91431, .F. ) ;
#34389=AXIS2_PLACEMENT_3D ( 'NONE', #23750, #84248, #22754 ) ;
#34392=CARTESIAN_POINT ( 'NONE',  ( -4.818768077841676600, -24.96217769842146694, -2.500000000000000000 ) ) ;
#34399=CARTESIAN_POINT ( 'NONE',  ( 6.757940885659567520, -58.32678904743372073, -3.999999999999999556 ) ) ;
#34408=DIRECTION ( 'NONE',  ( -0.000000000000000000, -0.000000000000000000, -1.000000000000000000 ) ) ;
#34411=FILL_AREA_STYLE_COLOUR ( '', #82816 ) ;
#34415=UNCERTAINTY_MEASURE_WITH_UNIT (LENGTH_MEASURE( 1.000000000000000082E-05 ), #44707, 'distance_accuracy_value', 'NONE');
#34422=CARTESIAN_POINT ( 'NONE',  ( 12.14357320772536575, 54.02013147999952736, 0.000000000000000000 ) ) ;
#34434=ORIENTED_EDGE ( 'NONE', *, *, #4119, .T. ) ;
#34438=CIRCLE ( 'NONE', #82335, 3.940000000000000835 ) ;
#34439=CARTESIAN_POINT ( 'NONE',  ( 3.969999999999999751, 37.00000000000000000, -2.500000000000000000 ) ) ;
#34448=EDGE_CURVE ( 'NONE', #55756, #80099, #68855, .T. ) ;
#34461=TOROIDAL_SURFACE ( 'NONE', #55158, 2.750000000000000888, 0.2500000000000000000 ) ;
#34464=ORIENTED_EDGE ( 'NONE', *, *, #73798, .F. ) ;
#34466=DIRECTION ( 'NONE',  ( 1.000000000000000000, 0.000000000000000000, 0.000000000000000000 ) ) ;
#34478=VECTOR ( 'NONE', #64925, 1000.000000000000000 ) ;
#34483=VERTEX_POINT ( 'NONE', #60351 ) ;
#34516=CARTESIAN_POINT ( 'NONE',  ( -6.732636091893173358, -88.11213685669363826, -2.500000000000000000 ) ) ;
#34520=AXIS2_PLACEMENT_3D ( 'NONE', #63069, #93569, #26072 ) ;
#34534=EDGE_LOOP ( 'NONE', ( #24062, #26822, #19295, #14213 ) ) ;
#34549=CARTESIAN_POINT ( 'NONE',  ( -4.139459722423021404, -8.271751626981556527, -4.000000000000000888 ) ) ;
#34550=VECTOR ( 'NONE', #7799, 999.9999999999998863 ) ;
#34569=CIRCLE ( 'NONE', #95240, 9.900000000000002132 ) ;
#34574=CARTESIAN_POINT ( 'NONE',  ( 0.000000000000000000, -97.00000000000000000, 3.750000000000000000 ) ) ;
#34575=AXIS2_PLACEMENT_3D ( 'NONE', #20252, #51237, #20746 ) ;
#34577=COLOUR_RGB ( '', 0.66274510, 0.83137255, 0.94901961) ;
#34584=EDGE_LOOP ( 'NONE', ( #57855, #93053, #95783, #69284 ) ) ;
#34589=DIRECTION ( 'NONE',  ( -1.000000000000000000, 0.000000000000000000, 0.000000000000000000 ) ) ;
#34593=FACE_OUTER_BOUND ( 'NONE', #60630, .T. ) ;
#34594=ORIENTED_EDGE ( 'NONE', *, *, #92397, .T. ) ;
#34597=CARTESIAN_POINT ( 'NONE',  ( 10.76560087618683603, -96.07989234454169036, 4.000000000000000000 ) ) ;
#34602=PLANE ( 'NONE',  #26729 ) ;
#34603=ORIENTED_EDGE ( 'NONE', *, *, #21710, .T. ) ;
#34605=CARTESIAN_POINT ( 'NONE',  ( -5.810137351020829399, -36.09275136659677230, 3.750000000000001332 ) ) ;
#34612=CARTESIAN_POINT ( 'NONE',  ( 11.61481287315787370, -90.96947208220468895, 3.750000000000000000 ) ) ;
#34619=AXIS2_PLACEMENT_3D ( 'NONE', #70765, #47746, #78242 ) ;
#34620=TOROIDAL_SURFACE ( 'NONE', #84119, 2.750000000000001776, 0.2500000000000000000 ) ;
#34628=LINE ( 'NONE', #65127, #43711 ) ;
#34634=CARTESIAN_POINT ( 'NONE',  ( -11.01424773186859696, -93.41215259627330170, -4.000000000000000000 ) ) ;
#34658=CARTESIAN_POINT ( 'NONE',  ( 4.903136312256997087, -13.39483660680936339, 3.750000000000001776 ) ) ;
#34669=ORIENTED_EDGE ( 'NONE', *, *, #47968, .T. ) ;
#34688=CYLINDRICAL_SURFACE ( 'NONE', #57133, 0.2500000000000002220 ) ;
#34710=B_SPLINE_CURVE_WITH_KNOTS ( 'NONE', 3,
 ( #27483, #36970, #13983, #35969, #44457, #73469, #66470, #27972, #81469, #57975, #4510, #97000, #59948, #20986, #59458, #28475, #58467, #89471 ),
 .UNSPECIFIED., .F., .F.,
 ( 4, 2, 2, 2, 2, 2, 2, 2, 4 ),
 ( 0.000000000000000000, 0.002783920674699109140, 0.005567841349398218280, 0.01113568269879643309, 0.02227136539759286271, 0.04454273079518572542, 0.06681409619277858813, 0.07794977889157500561, 0.08908546159037145085 ),
 .UNSPECIFIED. ) ;
#34713=FACE_OUTER_BOUND ( 'NONE', #51047, .T. ) ;
#34716=VECTOR ( 'NONE', #15707, 1000.000000000000000 ) ;
#34720=DIRECTION ( 'NONE',  ( 1.000000000000000000, 0.000000000000000000, 0.000000000000000000 ) ) ;
#34724=( NAMED_UNIT ( * ) PLANE_ANGLE_UNIT ( ) SI_UNIT ( $, .RADIAN. ) );
#34732=SURFACE_STYLE_FILL_AREA ( #10774 ) ;
#34744=B_SPLINE_CURVE_WITH_KNOTS ( 'NONE', 3,
 ( #31315, #9815, #92322, #23847, #78799, #92810, #70821, #54313 ),
 .UNSPECIFIED., .F., .F.,
 ( 4, 2, 2, 4 ),
 ( -1.048808863134852564E-05, 0.0008972750855482683431, 0.001351156672638076373, 0.001805038259727884294 ),
 .UNSPECIFIED. ) ;
#34754=( NAMED_UNIT ( * ) SI_UNIT ( $, .STERADIAN. ) SOLID_ANGLE_UNIT ( ) );
#34765=ADVANCED_FACE ( 'NONE', ( #17334 ), #97608, .T. ) ;
#34766=CARTESIAN_POINT ( 'NONE',  ( -6.607077432771771619, -50.94230397256625764, 2.750000000000001332 ) ) ;
#34774=EDGE_CURVE ( 'NONE', #75803, #92371, #16148, .T. ) ;
#34778=ORIENTED_EDGE ( 'NONE', *, *, #68187, .T. ) ;
#34780=FILL_AREA_STYLE_COLOUR ( '', #76595 ) ;
#34793=( GEOMETRIC_REPRESENTATION_CONTEXT ( 3 ) GLOBAL_UNCERTAINTY_ASSIGNED_CONTEXT ( ( #64299 ) ) GLOBAL_UNIT_ASSIGNED_CONTEXT ( ( #77680, #95528, #2210 ) ) REPRESENTATION_CONTEXT ( 'NONE', 'WORKASPACE' ) );
#34794=STYLED_ITEM ( 'NONE', ( #65056 ), #70016 ) ;
#34795=ORIENTED_EDGE ( 'NONE', *, *, #2208, .T. ) ;
#34801=CARTESIAN_POINT ( 'NONE',  ( -7.750355510519348456, 84.07179676972448590, -4.000000000000000000 ) ) ;
#34816=DIRECTION ( 'NONE',  ( 0.8070303256584298035, -0.5905099943842175847, 0.000000000000000000 ) ) ;
#34829=VERTEX_POINT ( 'NONE', #95782 ) ;
#34830=CARTESIAN_POINT ( 'NONE',  ( -19.00000000000000000, 75.76920769491739804, -3.000000000000000000 ) ) ;
#34839=CARTESIAN_POINT ( 'NONE',  ( -15.00000000000000000, 83.99999999999998579, -3.750000000000000000 ) ) ;
#34853=ADVANCED_FACE ( 'NONE', ( #58241 ), #20272, .F. ) ;
#34868=DIRECTION ( 'NONE',  ( -1.000000000000000000, -0.000000000000000000, -0.000000000000000000 ) ) ;
#34874=DIRECTION ( 'NONE',  ( 1.000000000000000000, 0.000000000000000000, -0.000000000000000000 ) ) ;
#34882=DIRECTION ( 'NONE',  ( 0.000000000000000000, 0.000000000000000000, 1.000000000000000000 ) ) ;
#34885=EDGE_CURVE ( 'NONE', #93321, #27291, #45952, .T. ) ;
#34896=ORIENTED_EDGE ( 'NONE', *, *, #89157, .F. ) ;
#34897=CARTESIAN_POINT ( 'NONE',  ( 7.007893109692266087, -58.32153039260716554, -4.000000000000000000 ) ) ;
#34899=SURFACE_STYLE_FILL_AREA ( #42419 ) ;
#34908=DIRECTION ( 'NONE',  ( -1.000000000000000000, 0.000000000000000000, 0.000000000000000000 ) ) ;
#34910=CARTESIAN_POINT ( 'NONE',  ( -15.00000000000000000, 84.07179676972448590, 4.000000000000000000 ) ) ;
#34917=VERTEX_POINT ( 'NONE', #42776 ) ;
#34926=VERTEX_POINT ( 'NONE', #80772 ) ;
#34928=EDGE_CURVE ( 'NONE', #875, #62733, #3802, .T. ) ;
#34943=CARTESIAN_POINT ( 'NONE',  ( 9.879999999999990123, 20.99999999999999645, 0.000000000000000000 ) ) ;
#34962=PLANE ( 'NONE',  #88833 ) ;
#34963=ORIENTED_EDGE ( 'NONE', *, *, #56725, .F. ) ;
#34990=ORIENTED_EDGE ( 'NONE', *, *, #24734, .T. ) ;
#35016=ORIENTED_EDGE ( 'NONE', *, *, #79791, .F. ) ;
#35017=VECTOR ( 'NONE', #69989, 1000.000000000000000 ) ;
#35022=CARTESIAN_POINT ( 'NONE',  ( 17.81748129626896215, 78.53842255729841781, -4.009548935143140369 ) ) ;
#35036=AXIS2_PLACEMENT_3D ( 'NONE', #25600, #55082, #46602 ) ;
#35038=ADVANCED_FACE ( 'NONE', ( #64759 ), #60107, .F. ) ;
#35040=FILL_AREA_STYLE ('',( #42559 ) ) ;
#35044=SURFACE_STYLE_USAGE ( .BOTH. , #67041 ) ;
#35051=DIRECTION ( 'NONE',  ( 1.000000000000000000, 0.000000000000000000, 0.000000000000000000 ) ) ;
#35064=ORIENTED_EDGE ( 'NONE', *, *, #46528, .F. ) ;
#35070=CARTESIAN_POINT ( 'NONE',  ( 9.879999999999988347, 26.99999999999999645, -2.900000000000000799 ) ) ;
#35072=ORIENTED_EDGE ( 'NONE', *, *, #59271, .T. ) ;
#35082=( NAMED_UNIT ( * ) SI_UNIT ( $, .STERADIAN. ) SOLID_ANGLE_UNIT ( ) );
#35084=( GEOMETRIC_REPRESENTATION_CONTEXT ( 3 ) GLOBAL_UNCERTAINTY_ASSIGNED_CONTEXT ( ( #26187 ) ) GLOBAL_UNIT_ASSIGNED_CONTEXT ( ( #59311, #69786, #61769 ) ) REPRESENTATION_CONTEXT ( 'NONE', 'WORKASPACE' ) );
#35088=PLANE ( 'NONE',  #71273 ) ;
#35091=EDGE_LOOP ( 'NONE', ( #72136, #33102, #95414 ) ) ;
#35095=FACE_OUTER_BOUND ( 'NONE', #51797, .T. ) ;
#35096=ORIENTED_EDGE ( 'NONE', *, *, #98248, .F. ) ;
#35103=ORIENTED_EDGE ( 'NONE', *, *, #87810, .T. ) ;
#35112=DIRECTION ( 'NONE',  ( 0.8070303256584298035, -0.5905099943842175847, 0.000000000000000000 ) ) ;
#35113=EDGE_CURVE ( 'NONE', #47034, #55759, #27749, .T. ) ;
#35123=FACE_OUTER_BOUND ( 'NONE', #98630, .T. ) ;
#35132=LINE ( 'NONE', #42173, #46818 ) ;
#35134=CARTESIAN_POINT ( 'NONE',  ( -3.749999999999993783, 43.00000000000000711, 4.000000000000000000 ) ) ;
#35142=UNCERTAINTY_MEASURE_WITH_UNIT (LENGTH_MEASURE( 1.000000000000000082E-05 ), #48010, 'distance_accuracy_value', 'NONE');
#35146=ORIENTED_EDGE ( 'NONE', *, *, #59717, .F. ) ;
#35149=CARTESIAN_POINT ( 'NONE',  ( 6.937721053838227014, -80.66520463107747219, 3.750000000000001776 ) ) ;
#35158=CIRCLE ( 'NONE', #86283, 1.500000000000001332 ) ;
#35160=VERTEX_POINT ( 'NONE', #5273 ) ;
#35161=SURFACE_SIDE_STYLE ('',( #3217 ) ) ;
#35163=ORIENTED_EDGE ( 'NONE', *, *, #61875, .F. ) ;
#35171=( LENGTH_UNIT ( ) NAMED_UNIT ( * ) SI_UNIT ( .MILLI., .METRE. ) );
#35178=FACE_OUTER_BOUND ( 'NONE', #63679, .T. ) ;
#35180=VERTEX_POINT ( 'NONE', #43247 ) ;
#35181=DIRECTION ( 'NONE',  ( -0.000000000000000000, -0.000000000000000000, -1.000000000000000000 ) ) ;
#35208=ADVANCED_FACE ( 'NONE', ( #96772 ), #44231, .F. ) ;
#35211=ADVANCED_FACE ( 'NONE', ( #28248 ), #58743, .F. ) ;
#35213=COLOUR_RGB ( '', 0.08235294, 0.09019608, 0.10196078) ;
#35214=DIRECTION ( 'NONE',  ( 0.000000000000000000, 1.000000000000000000, 0.000000000000000000 ) ) ;
#35215=AXIS2_PLACEMENT_3D ( 'NONE', #73031, #55593, #40591 ) ;
#35226=CIRCLE ( 'NONE', #30448, 0.2500000000000002220 ) ;
#35235=EDGE_CURVE ( 'NONE', #80582, #67582, #12258, .T. ) ;
#35238=PLANE ( 'NONE',  #20167 ) ;
#35249=DIRECTION ( 'NONE',  ( 0.000000000000000000, 0.000000000000000000, -1.000000000000000000 ) ) ;
#35253=CARTESIAN_POINT ( 'NONE',  ( 11.24699797944280100, 54.09857164847241506, -2.899999999999999467 ) ) ;
#35259=ORIENTED_EDGE ( 'NONE', *, *, #30368, .T. ) ;
#35262=DIRECTION ( 'NONE',  ( 0.000000000000000000, -0.000000000000000000, -1.000000000000000000 ) ) ;
#35263=CARTESIAN_POINT ( 'NONE',  ( -10.34223742324318884, 89.23976162705962167, -5.715022854599768110 ) ) ;
#35265=DIRECTION ( 'NONE',  ( 0.000000000000000000, 0.000000000000000000, 1.000000000000000000 ) ) ;
#35266=UNCERTAINTY_MEASURE_WITH_UNIT (LENGTH_MEASURE( 1.000000000000000082E-05 ), #55945, 'distance_accuracy_value', 'NONE');
#35270=ORIENTED_EDGE ( 'NONE', *, *, #75307, .F. ) ;
#35271=FILL_AREA_STYLE ('',( #26788 ) ) ;
#35289=FILL_AREA_STYLE_COLOUR ( '', #17329 ) ;
#35294=DIRECTION ( 'NONE',  ( -4.336808689942013792E-16, 1.000000000000000000, 0.000000000000000000 ) ) ;
#35299=MECHANICAL_DESIGN_GEOMETRIC_PRESENTATION_REPRESENTATION('',(#225),#79983);
#35300=DIRECTION ( 'NONE',  ( 1.000000000000000000, 0.000000000000000000, 0.000000000000000000 ) ) ;
#35303=DIRECTION ( 'NONE',  ( -0.000000000000000000, 0.000000000000000000, 1.000000000000000000 ) ) ;
#35307=ORIENTED_EDGE ( 'NONE', *, *, #90944, .F. ) ;
#35313=FILL_AREA_STYLE_COLOUR ( '', #66838 ) ;
#35333=CIRCLE ( 'NONE', #19495, 0.2500000000000002220 ) ;
#35349=CIRCLE ( 'NONE', #96039, 1.249999999999987121 ) ;
#35357=VERTEX_POINT ( 'NONE', #76228 ) ;
#35359=DIRECTION ( 'NONE',  ( 1.927470528863119295E-16, -1.000000000000000000, 0.000000000000000000 ) ) ;
#35366=STYLED_ITEM ( 'NONE', ( #29497 ), #46646 ) ;
#35375=AXIS2_PLACEMENT_3D ( 'NONE', #17614, #48580, #19566 ) ;
#35379=FACE_OUTER_BOUND ( 'NONE', #59781, .T. ) ;
#35382=EDGE_CURVE ( 'NONE', #70499, #38896, #36129, .T. ) ;
#35383=LINE ( 'NONE', #20394, #13180 ) ;
#35385=VERTEX_POINT ( 'NONE', #98264 ) ;
#35387=CARTESIAN_POINT ( 'NONE',  ( -6.732636091893170693, -88.11213685669366669, -2.500000000000000888 ) ) ;
#35394=CARTESIAN_POINT ( 'NONE',  ( 4.920853330210497312, -13.83152733635706433, -3.750000000000804690 ) ) ;
#35396=CARTESIAN_POINT ( 'NONE',  ( -4.021969307579356112, -6.415483651463659953, 3.999999999999999112 ) ) ;
#35406=AXIS2_PLACEMENT_3D ( 'NONE', #6252, #12754, #87762 ) ;
#35407=FILL_AREA_STYLE ('',( #34411 ) ) ;
#35415=ORIENTED_EDGE ( 'NONE', *, *, #35235, .T. ) ;
#35426=ADVANCED_FACE ( 'NONE', ( #84711 ), #7742, .F. ) ;
#35433=CARTESIAN_POINT ( 'NONE',  ( 4.441537491530695547, -2.700695904843435802, 4.000000000000000000 ) ) ;
#35463=ORIENTED_EDGE ( 'NONE', *, *, #83758, .T. ) ;
#35465=FACE_OUTER_BOUND ( 'NONE', #54145, .T. ) ;
#35470=CARTESIAN_POINT ( 'NONE',  ( -6.982525766850296911, -88.11956318484570261, 2.750000000000000444 ) ) ;
#35487=PRESENTATION_STYLE_ASSIGNMENT (( #96509 ) ) ;
#35492=VERTEX_POINT ( 'NONE', #85202 ) ;
#35506=DIRECTION ( 'NONE',  ( 1.000000000000000000, 0.000000000000000000, 0.000000000000000000 ) ) ;
#35510=AXIS2_PLACEMENT_3D ( 'NONE', #86273, #25778, #2799 ) ;
#35516=CARTESIAN_POINT ( 'NONE',  ( 6.879999999999995453, 41.24999999999999289, 6.250000000000000000 ) ) ;
#35521=AXIS2_PLACEMENT_3D ( 'NONE', #47312, #54323, #60847 ) ;
#35523=CARTESIAN_POINT ( 'NONE',  ( 12.99999999999999822, 75.00000000000000000, -8.525133428036872019 ) ) ;
#35527=CARTESIAN_POINT ( 'NONE',  ( 17.78441314508118509, 78.67289652296345537, -4.000000000000000000 ) ) ;
#35533=FILL_AREA_STYLE ('',( #50047 ) ) ;
#35538=CYLINDRICAL_SURFACE ( 'NONE', #36634, 1.000000000000000888 ) ;
#35551=CARTESIAN_POINT ( 'NONE',  ( 8.956085929493502462, -3.116154469452326214, -3.750000000000000000 ) ) ;
#35552=CARTESIAN_POINT ( 'NONE',  ( -3.628626191893884467, -3.642031182898920694, -3.750000000000000000 ) ) ;
#35565=LINE ( 'NONE', #44547, #65809 ) ;
#35568=ORIENTED_EDGE ( 'NONE', *, *, #5338, .F. ) ;
#35569=SURFACE_STYLE_FILL_AREA ( #74052 ) ;
#35570=ORIENTED_EDGE ( 'NONE', *, *, #78452, .T. ) ;
#35576=DIRECTION ( 'NONE',  ( 0.000000000000000000, 0.000000000000000000, 1.000000000000000000 ) ) ;
#35581=AXIS2_PLACEMENT_3D ( 'NONE', #75197, #83697, #97737 ) ;
#35583=AXIS2_PLACEMENT_3D ( 'NONE', #5995, #59470, #88994 ) ;
#35585=ORIENTED_EDGE ( 'NONE', *, *, #21195, .T. ) ;
#35593=FILL_AREA_STYLE_COLOUR ( '', #79294 ) ;
#35595=PRESENTATION_STYLE_ASSIGNMENT (( #5103 ) ) ;
#35600=DIRECTION ( 'NONE',  ( 0.000000000000000000, 0.000000000000000000, -1.000000000000000000 ) ) ;
#35602=CARTESIAN_POINT ( 'NONE',  ( -6.982525766139713319, -88.11956320875633253, 2.750000000000000000 ) ) ;
#35610=CARTESIAN_POINT ( 'NONE',  ( -8.000000000000000000, 79.82179676972448590, 4.250000000000000000 ) ) ;
#35614=CARTESIAN_POINT ( 'NONE',  ( 8.879999999999995453, 40.74999999999999289, 3.750000000000000000 ) ) ;
#35619=CARTESIAN_POINT ( 'NONE',  ( 51.94498256489735155, 70.99147617202632432, -8.000000000000000000 ) ) ;
#35623=VECTOR ( 'NONE', #8304, 1000.000000000000114 ) ;
#35630=CARTESIAN_POINT ( 'NONE',  ( -3.635384400432159158, -3.854802480546752896, -3.750000000000000000 ) ) ;
#35633=FACE_OUTER_BOUND ( 'NONE', #70062, .T. ) ;
#35638=CARTESIAN_POINT ( 'NONE',  ( -10.85639881947519036, -98.10817599903623432, -4.000000000005668355 ) ) ;
#35647=DIRECTION ( 'NONE',  ( 0.000000000000000000, 0.000000000000000000, -1.000000000000000000 ) ) ;
#35667=CARTESIAN_POINT ( 'NONE',  ( 14.99999999999997868, 80.07179676972448590, -4.250000000000000000 ) ) ;
#35672=SURFACE_STYLE_USAGE ( .BOTH. , #89657 ) ;
#35679=( NAMED_UNIT ( * ) SI_UNIT ( $, .STERADIAN. ) SOLID_ANGLE_UNIT ( ) );
#35686=LINE ( 'NONE', #4716, #76341 ) ;
#35698=EDGE_CURVE ( 'NONE', #79084, #73802, #78103, .T. ) ;
#35711=DIRECTION ( 'NONE',  ( 0.9961946980917453232, -0.08715574274766037244, 0.000000000000000000 ) ) ;
#35714=VECTOR ( 'NONE', #77725, 1000.000000000000114 ) ;
#35728=LINE ( 'NONE', #66216, #44823 ) ;
#35731=DIRECTION ( 'NONE',  ( 0.08715574274765139351, 0.9961946980917461003, 0.000000000000000000 ) ) ;
#35739=VERTEX_POINT ( 'NONE', #95061 ) ;
#35750=( NAMED_UNIT ( * ) SI_UNIT ( $, .STERADIAN. ) SOLID_ANGLE_UNIT ( ) );
#35754=CARTESIAN_POINT ( 'NONE',  ( 6.905580141755321755, -69.44847572026166915, 3.750000000000000444 ) ) ;
#35759=VERTEX_POINT ( 'NONE', #10109 ) ;
#35762=CARTESIAN_POINT ( 'NONE',  ( 0.000000000000000000, -97.00000000000000000, 4.000000000000000000 ) ) ;
#35763=CARTESIAN_POINT ( 'NONE',  ( -13.05265508282229980, 90.73577164613095647, -7.477963345816291962 ) ) ;
#35765=EDGE_CURVE ( 'NONE', #40706, #2502, #94576, .T. ) ;
#35779=( NAMED_UNIT ( * ) PLANE_ANGLE_UNIT ( ) SI_UNIT ( $, .RADIAN. ) );
#35785=EDGE_CURVE ( 'NONE', #68711, #14972, #88733, .T. ) ;
#35788=SURFACE_SIDE_STYLE ('',( #97304 ) ) ;
#35789=CIRCLE ( 'NONE', #16672, 1.249999999999987121 ) ;
#35809=VERTEX_POINT ( 'NONE', #2631 ) ;
#35816=LINE ( 'NONE', #66302, #6852 ) ;
#35836=LINE ( 'NONE', #12344, #89797 ) ;
#35848=PLANE ( 'NONE',  #53877 ) ;
#35851=VERTEX_POINT ( 'NONE', #55092 ) ;
#35858=COLOUR_RGB ( '', 0.66274510, 0.83137255, 0.94901961) ;
#35862=CARTESIAN_POINT ( 'NONE',  ( -6.430724159521292727, -88.51069574204372259, 3.750000000000000000 ) ) ;
#35875=CARTESIAN_POINT ( 'NONE',  ( -13.77612262535527954, 90.93158326518027934, 7.883772450803742338 ) ) ;
#35878=CARTESIAN_POINT ( 'NONE',  ( 6.829574850505127692, -88.00372650098204019, -3.749999999999998668 ) ) ;
#35886=DIRECTION ( 'NONE',  ( -1.000000000000000000, -2.569960705150834273E-16, 0.000000000000000000 ) ) ;
#35890=CARTESIAN_POINT ( 'NONE',  ( 5.800000000000003375, 99.99999999999998579, -8.000000000000000000 ) ) ;
#35893=DIRECTION ( 'NONE',  ( 1.000000000000000000, 1.257402221000611116E-16, -0.000000000000000000 ) ) ;
#35899=ADVANCED_FACE ( 'NONE', ( #16623 ), #74309, .T. ) ;
#35910=EDGE_LOOP ( 'NONE', ( #86322, #11613, #38731, #49990 ) ) ;
#35912=LINE ( 'NONE', #19442, #52589 ) ;
#35918=ORIENTED_EDGE ( 'NONE', *, *, #15312, .T. ) ;
#35928=CARTESIAN_POINT ( 'NONE',  ( -15.00000000000004974, 91.00000000000000000, -7.750000000000000000 ) ) ;
#35929=CARTESIAN_POINT ( 'NONE',  ( -7.750000000000000000, 43.00000000000000000, 6.500000000000000888 ) ) ;
#35930=CARTESIAN_POINT ( 'NONE',  ( -19.00000000000000000, 75.76920769491739804, 3.000000000000000000 ) ) ;
#35935=CARTESIAN_POINT ( 'NONE',  ( -11.02682316214847980, -96.56463058013387979, -3.750000000000000000 ) ) ;
#35948=ADVANCED_FACE ( 'NONE', ( #88055 ), #64736, .T. ) ;
#35950=FACE_OUTER_BOUND ( 'NONE', #68781, .T. ) ;
#35963=LINE ( 'NONE', #37465, #72364 ) ;
#35969=CARTESIAN_POINT ( 'NONE',  ( 4.691427381388423079, -2.693150427207441133, 4.000000000000000888 ) ) ;
#35971=VECTOR ( 'NONE', #94179, 1000.000000000000000 ) ;
#36003=DIRECTION ( 'NONE',  ( 0.000000000000000000, 0.000000000000000000, -1.000000000000000000 ) ) ;
#36006=FACE_OUTER_BOUND ( 'NONE', #62462, .T. ) ;
#36015=VERTEX_POINT ( 'NONE', #53509 ) ;
#36026=CYLINDRICAL_SURFACE ( 'NONE', #36955, 1.249999999999987121 ) ;
#36038=CARTESIAN_POINT ( 'NONE',  ( 17.75000000000000000, 84.07179676972448590, -12.00000000000000000 ) ) ;
#36050=DIRECTION ( 'NONE',  ( 0.9961946980917462113, -0.08715574274765114371, -0.000000000000000000 ) ) ;
#36051=LINE ( 'NONE', #36558, #49852 ) ;
#36056=CARTESIAN_POINT ( 'NONE',  ( 6.599999999999995204, -97.00000000000000000, -3.750000000000000000 ) ) ;
#36083=CARTESIAN_POINT ( 'NONE',  ( 17.82550663882221542, 78.51652494792099901, -4.000000000000000888 ) ) ;
#36097=EDGE_LOOP ( 'NONE', ( #53274, #33118, #228, #42943 ) ) ;
#36108=DIRECTION ( 'NONE',  ( -1.000000000000000000, 0.000000000000000000, 0.000000000000000000 ) ) ;
#36110=AXIS2_PLACEMENT_3D ( 'NONE', #21431, #75405, #89917 ) ;
#36117=CARTESIAN_POINT ( 'NONE',  ( 44.01201084850834633, 60.14974815962801813, -8.000000000000000000 ) ) ;
#36123=CARTESIAN_POINT ( 'NONE',  ( -10.82625193726620338, -96.00405735513218985, -4.000000000000000000 ) ) ;
#36126=VECTOR ( 'NONE', #39820, 1000.000000000000000 ) ;
#36128=CARTESIAN_POINT ( 'NONE',  ( 6.934011249083991579, -73.15940021104376001, -3.750000000000000444 ) ) ;
#36129=CIRCLE ( 'NONE', #25033, 0.2500000000000002220 ) ;
#36131=AXIS2_PLACEMENT_3D ( 'NONE', #15358, #55293, #47791 ) ;
#36132=CIRCLE ( 'NONE', #61678, 7.250000000000002665 ) ;
#36162=ORIENTED_EDGE ( 'NONE', *, *, #60120, .F. ) ;
#36172=CARTESIAN_POINT ( 'NONE',  ( -11.20041124612599504, -94.46430075981348295, 3.750000000000000000 ) ) ;
#36183=ORIENTED_EDGE ( 'NONE', *, *, #23665, .F. ) ;
#36184=EDGE_LOOP ( 'NONE', ( #60653, #3365, #26828, #33234 ) ) ;
#36190=CARTESIAN_POINT ( 'NONE',  ( -8.900000000000002132, 80.99999999999994316, 3.000000000000000000 ) ) ;
#36197=EDGE_LOOP ( 'NONE', ( #96366, #49492, #28185, #68502 ) ) ;
#36210=CARTESIAN_POINT ( 'NONE',  ( 14.99999999999997868, 80.07179676972448590, -6.500000000000000888 ) ) ;
#36228=CARTESIAN_POINT ( 'NONE',  ( 11.34661744925197624, 54.08985607419764818, 0.000000000000000000 ) ) ;
#36231=ADVANCED_FACE ( 'NONE', ( #70497 ), #85001, .T. ) ;
#36253=FILL_AREA_STYLE_COLOUR ( '', #83305 ) ;
#36263=CARTESIAN_POINT ( 'NONE',  ( -5.999999999999994671, 43.00000000000000000, 6.500000000000000888 ) ) ;
#36268=EDGE_CURVE ( 'NONE', #79084, #12193, #3000, .T. ) ;
#36277=CARTESIAN_POINT ( 'NONE',  ( 6.880000000000009663, 40.74999999999999289, 4.250000000000000000 ) ) ;
#36287=CARTESIAN_POINT ( 'NONE',  ( -8.099999999999999645, 80.99999999999994316, -3.000000000000000000 ) ) ;
#36296=CARTESIAN_POINT ( 'NONE',  ( 6.655501998725182666, -69.44085999584420676, -2.499999999999999556 ) ) ;
#36299=COLOUR_RGB ( '', 0.66274510, 0.83137255, 0.94901961) ;
#36300=( LENGTH_UNIT ( ) NAMED_UNIT ( * ) SI_UNIT ( .MILLI., .METRE. ) );
#36318=EDGE_CURVE ( 'NONE', #91549, #38899, #13654, .T. ) ;
#36348=AXIS2_PLACEMENT_3D ( 'NONE', #67550, #13552, #22549 ) ;
#36349=CARTESIAN_POINT ( 'NONE',  ( -5.999999999999994671, 43.00000000000000000, -4.250000000000000000 ) ) ;
#36357=DIRECTION ( 'NONE',  ( 0.6246950475544238435, 0.7808688094430307203, 0.000000000000000000 ) ) ;
#36362=AXIS2_PLACEMENT_3D ( 'NONE', #50189, #35181, #87208 ) ;
#36369=ORIENTED_EDGE ( 'NONE', *, *, #43686, .F. ) ;
#36371=VECTOR ( 'NONE', #51500, 1000.000000000000114 ) ;
#36391=CARTESIAN_POINT ( 'NONE',  ( -11.33436264772833724, -69.53389133802667743, -3.999999999999999112 ) ) ;
#36415=DIRECTION ( 'NONE',  ( -0.9961946980917461003, 0.08715574274765068574, 0.000000000000000000 ) ) ;
#36431=SURFACE_STYLE_FILL_AREA ( #43427 ) ;
#36432=FILL_AREA_STYLE_COLOUR ( '', #56884 ) ;
#36437=CARTESIAN_POINT ( 'NONE',  ( -10.85532661662059972, -98.11526154878892214, -3.749999999999999556 ) ) ;
#36462=PRODUCT ( '1.0 Fixed Jaw', '1.0 Fixed Jaw', '', ( #60699 ) ) ;
#36467=CARTESIAN_POINT ( 'NONE',  ( -6.871342362925322078, -73.24551516664604378, 2.500000000000000000 ) ) ;
#36471=CARTESIAN_POINT ( 'NONE',  ( 9.729341964144056831, -19.62354698955503451, 4.000000000000000000 ) ) ;
#36476=CARTESIAN_POINT ( 'NONE',  ( -7.199999999999996625, 99.99999999999998579, -8.525133428036873795 ) ) ;
#36488=DIRECTION ( 'NONE',  ( -0.000000000000000000, 0.000000000000000000, 1.000000000000000000 ) ) ;
#36523=MECHANICAL_DESIGN_GEOMETRIC_PRESENTATION_REPRESENTATION('',(#2998),#41318);
#36526=FACE_OUTER_BOUND ( 'NONE', #4021, .T. ) ;
#36550=CARTESIAN_POINT ( 'NONE',  ( 9.730224124549700093, -19.64066503251600793, -3.750000000000000444 ) ) ;
#36558=CARTESIAN_POINT ( 'NONE',  ( -5.149999999999996803, 98.49999999999998579, 8.000000000000000000 ) ) ;
#36578=EDGE_CURVE ( 'NONE', #68087, #8055, #81913, .T. ) ;
#36592=DIRECTION ( 'NONE',  ( 1.000000000000000000, -1.244644646440729013E-15, 0.000000000000000000 ) ) ;
#36608=CARTESIAN_POINT ( 'NONE',  ( 4.469999999999999751, 10.00000000000000000, 4.000000000000000000 ) ) ;
#36612=EDGE_LOOP ( 'NONE', ( #72801, #83848, #9252, #46614 ) ) ;
#36621=CARTESIAN_POINT ( 'NONE',  ( -9.000000000000001776, 80.99999999999994316, 0.000000000000000000 ) ) ;
#36631=EDGE_CURVE ( 'NONE', #35160, #57591, #53694, .T. ) ;
#36634=AXIS2_PLACEMENT_3D ( 'NONE', #4074, #27541, #43048 ) ;
#36662=ORIENTED_EDGE ( 'NONE', *, *, #23665, .T. ) ;
#36674=CARTESIAN_POINT ( 'NONE',  ( -11.02874191901561041, -96.54482102870888127, 4.000000000000000000 ) ) ;
#36689=ORIENTED_EDGE ( 'NONE', *, *, #98608, .F. ) ;
#36712=EDGE_LOOP ( 'NONE', ( #64899, #1758, #48040, #14703 ) ) ;
#36713=ADVANCED_FACE ( 'NONE', ( #44408 ), #61605, .F. ) ;
#36714=CIRCLE ( 'NONE', #92586, 3.250000000000002665 ) ;
#36718=DIRECTION ( 'NONE',  ( -0.000000000000000000, 1.000000000000000000, -0.000000000000000000 ) ) ;
#36719=SURFACE_STYLE_USAGE ( .BOTH. , #6215 ) ;
#36723=CARTESIAN_POINT ( 'NONE',  ( -3.750000000000000000, 10.25000000000000000, -2.750000000000000000 ) ) ;
#36730=DIRECTION ( 'NONE',  ( 0.000000000000000000, -0.000000000000000000, -1.000000000000000000 ) ) ;
#36744=FILL_AREA_STYLE ('',( #52231 ) ) ;
#36746=FACE_OUTER_BOUND ( 'NONE', #74800, .T. ) ;
#36766=LINE ( 'NONE', #81266, #24472 ) ;
#36772=CARTESIAN_POINT ( 'NONE',  ( 9.729335482426746395, -19.62342160288699588, -3.750000000000000000 ) ) ;
#36779=PRESENTATION_STYLE_ASSIGNMENT (( #74255 ) ) ;
#36797=DIRECTION ( 'NONE',  ( -0.9961946980917459893, 0.08715574274765408580, -0.000000000000000000 ) ) ;
#36800=CARTESIAN_POINT ( 'NONE',  ( -3.628626191893843167, -3.642031182898128439, 3.749999999999596323 ) ) ;
#36801=VERTEX_POINT ( 'NONE', #54908 ) ;
#36807=EDGE_CURVE ( 'NONE', #46091, #25626, #49379, .T. ) ;
#36811=MECHANICAL_DESIGN_GEOMETRIC_PRESENTATION_REPRESENTATION('',(#33568),#88);
#36817=VECTOR ( 'NONE', #82517, 1000.000000000000000 ) ;
#36825=AXIS2_PLACEMENT_3D ( 'NONE', #28205, #58701, #81693 ) ;
#36844=CIRCLE ( 'NONE', #30479, 2.000000000000000888 ) ;
#36848=ORIENTED_EDGE ( 'NONE', *, *, #90779, .T. ) ;
#36854=CARTESIAN_POINT ( 'NONE',  ( 6.935134328218562239, -80.57830137102044432, -2.750000000000000444 ) ) ;
#36857=DIRECTION ( 'NONE',  ( 0.5150380749100554878, 1.049727191138617710E-16, 0.8571673007021115565 ) ) ;
#36863=DIRECTION ( 'NONE',  ( 1.000000000000000000, 0.000000000000000000, 0.000000000000000000 ) ) ;
#36868=ORIENTED_EDGE ( 'NONE', *, *, #38207, .F. ) ;
#36869=FILL_AREA_STYLE_COLOUR ( '', #46478 ) ;
#36872=DIRECTION ( 'NONE',  ( -0.000000000000000000, -0.000000000000000000, 1.000000000000000000 ) ) ;
#36874=MECHANICAL_DESIGN_GEOMETRIC_PRESENTATION_REPRESENTATION('',(#27290),#14550);
#36876=SURFACE_SIDE_STYLE ('',( #6868 ) ) ;
#36880=CARTESIAN_POINT ( 'NONE',  ( -7.037799270021981357, -86.25965645051654462, -2.749999999998791189 ) ) ;
#36916=ORIENTED_EDGE ( 'NONE', *, *, #19708, .T. ) ;
#36921=ADVANCED_FACE ( 'NONE', ( #31905 ), #10410, .F. ) ;
#36929=AXIS2_PLACEMENT_3D ( 'NONE', #6496, #59004, #82993 ) ;
#36933=EDGE_CURVE ( 'NONE', #5021, #89406, #24933, .T. ) ;
#36934=CARTESIAN_POINT ( 'NONE',  ( 0.000000000000000000, 91.25000000000000000, 7.750000000000000000 ) ) ;
#36943=CARTESIAN_POINT ( 'NONE',  ( -7.750000000000000000, 40.74999999999999289, -4.250000000000000000 ) ) ;
#36944=( GEOMETRIC_REPRESENTATION_CONTEXT ( 3 ) GLOBAL_UNCERTAINTY_ASSIGNED_CONTEXT ( ( #64421 ) ) GLOBAL_UNIT_ASSIGNED_CONTEXT ( ( #90700, #44207, #5251 ) ) REPRESENTATION_CONTEXT ( 'NONE', 'WORKASPACE' ) );
#36955=AXIS2_PLACEMENT_3D ( 'NONE', #66528, #65529, #50540 ) ;
#36963=CARTESIAN_POINT ( 'NONE',  ( -6.030006457173053391, -39.79017371240020395, 2.499999999999193534 ) ) ;
#36966=CARTESIAN_POINT ( 'NONE',  ( -3.999999999999994671, 43.00000000000000711, 6.250000000000000000 ) ) ;
#36970=CARTESIAN_POINT ( 'NONE',  ( 4.630000000000001670, 0.09071050906739680508, 4.000000000000000000 ) ) ;
#36989=CARTESIAN_POINT ( 'NONE',  ( 18.00000000000000000, 78.06026161867410451, 3.869897282520398551 ) ) ;
#36990=EDGE_CURVE ( 'NONE', #73831, #85496, #92329, .T. ) ;
#36996=CIRCLE ( 'NONE', #43328, 0.2500000000000002220 ) ;
#36998=VERTEX_POINT ( 'NONE', #77912 ) ;
#37013=SURFACE_STYLE_FILL_AREA ( #81509 ) ;
#37026=DIRECTION ( 'NONE',  ( 1.000000000000000000, -0.000000000000000000, 0.000000000000000000 ) ) ;
#37028=STYLED_ITEM ( 'NONE', ( #7811 ), #47403 ) ;
#37043=CARTESIAN_POINT ( 'NONE',  ( 8.880000000000000782, 1.019547802438458550, -3.750000000000000000 ) ) ;
#37044=CARTESIAN_POINT ( 'NONE',  ( -5.070949216187652375, -24.98410106517849982, -3.750000000001612044 ) ) ;
#37045=VERTEX_POINT ( 'NONE', #9923 ) ;
#37046=ORIENTED_EDGE ( 'NONE', *, *, #83578, .F. ) ;
#37052=CARTESIAN_POINT ( 'NONE',  ( -13.59072821819446020, 90.85999462608982924, -7.686992381060815838 ) ) ;
#37063=ORIENTED_EDGE ( 'NONE', *, *, #39541, .T. ) ;
#37066=VERTEX_POINT ( 'NONE', #4396 ) ;
#37089=DIRECTION ( 'NONE',  ( 0.000000000000000000, 0.000000000000000000, 1.000000000000000000 ) ) ;
#37093=VERTEX_POINT ( 'NONE', #65358 ) ;
#37096=COLOUR_RGB ( '', 0.72549020, 0.75294118, 0.79215686) ;
#37099=PRESENTATION_STYLE_ASSIGNMENT (( #6102 ) ) ;
#37107=AXIS2_PLACEMENT_3D ( 'NONE', #65878, #43865, #96406 ) ;
#37115=AXIS2_PLACEMENT_3D ( 'NONE', #49671, #94699, #4698 ) ;
#37117=ORIENTED_EDGE ( 'NONE', *, *, #6400, .T. ) ;
#37124=FACE_BOUND ( 'NONE', #34324, .T. ) ;
#37134=DIRECTION ( 'NONE',  ( -0.000000000000000000, -0.000000000000000000, -1.000000000000000000 ) ) ;
#37152=CARTESIAN_POINT ( 'NONE',  ( 0.000000000000000000, 40.74999999999999289, -4.250000000000000000 ) ) ;
#37163=STYLED_ITEM ( 'NONE', ( #49614 ), #65095 ) ;
#37167=EDGE_LOOP ( 'NONE', ( #37063, #1496, #2297, #92492 ) ) ;
#37168=ORIENTED_EDGE ( 'NONE', *, *, #6952, .F. ) ;
#37169=( LENGTH_UNIT ( ) NAMED_UNIT ( * ) SI_UNIT ( .MILLI., .METRE. ) );
#37176=CARTESIAN_POINT ( 'NONE',  ( -8.330954873910256353, -7.272562134485029084, 4.000000000000000000 ) ) ;
#37184=FILL_AREA_STYLE ('',( #74159 ) ) ;
#37189=VERTEX_POINT ( 'NONE', #58848 ) ;
#37202=ORIENTED_EDGE ( 'NONE', *, *, #92786, .T. ) ;
#37218=CARTESIAN_POINT ( 'NONE',  ( 11.49974963341099077, 56.98753627293847757, 0.000000000000000000 ) ) ;
#37223=CARTESIAN_POINT ( 'NONE',  ( 6.880000000000009663, 40.99999999999999289, -4.250000000000000000 ) ) ;
#37238=MECHANICAL_DESIGN_GEOMETRIC_PRESENTATION_REPRESENTATION('',(#3684),#26021);
#37248=AXIS2_PLACEMENT_3D ( 'NONE', #7121, #90112, #83614 ) ;
#37261=DIRECTION ( 'NONE',  ( -0.9997628902338895340, 0.02177529129954166101, 1.734723475976803939E-15 ) ) ;
#37262=ADVANCED_FACE ( 'NONE', ( #43353 ), #74983, .F. ) ;
#37277=CARTESIAN_POINT ( 'NONE',  ( 11.18126922390458589, -92.99194761432693213, -3.999999999999103384 ) ) ;
#37289=TOROIDAL_SURFACE ( 'NONE', #26070, 9.900000000000002132, 0.1000000000000000056 ) ;
#37298=CARTESIAN_POINT ( 'NONE',  ( -19.64999999999999858, 0.000000000000000000, 7.750000000000000000 ) ) ;
#37303=CYLINDRICAL_SURFACE ( 'NONE', #52300, 2.999999999999998224 ) ;
#37306=FACE_OUTER_BOUND ( 'NONE', #53962, .T. ) ;
#37307=ORIENTED_EDGE ( 'NONE', *, *, #64553, .T. ) ;
#37311=ORIENTED_EDGE ( 'NONE', *, *, #96135, .F. ) ;
#37317=AXIS2_PLACEMENT_3D ( 'NONE', #22591, #84563, #16065 ) ;
#37326=SURFACE_STYLE_USAGE ( .BOTH. , #83798 ) ;
#37344=CARTESIAN_POINT ( 'NONE',  ( 4.920097194114470440, -13.81670059445664300, -3.749999999999997780 ) ) ;
#37346=PRESENTATION_STYLE_ASSIGNMENT (( #68821 ) ) ;
#37350=CARTESIAN_POINT ( 'NONE',  ( -0.000000000000000000, 37.25000000000000000, -3.750000000000000000 ) ) ;
#37371=CARTESIAN_POINT ( 'NONE',  ( -41.28048780487802105, 33.02439024390238131, -8.000000000000000000 ) ) ;
#37372=ADVANCED_FACE ( 'NONE', ( #71657 ), #10626, .T. ) ;
#37375=DIRECTION ( 'NONE',  ( 0.02970531260826360376, -0.9995586998285020952, -0.000000000000000000 ) ) ;
#37378=( NAMED_UNIT ( * ) PLANE_ANGLE_UNIT ( ) SI_UNIT ( $, .RADIAN. ) );
#37392=( NAMED_UNIT ( * ) PLANE_ANGLE_UNIT ( ) SI_UNIT ( $, .RADIAN. ) );
#37403=LINE ( 'NONE', #51401, #63454 ) ;
#37407=EDGE_CURVE ( 'NONE', #85917, #66682, #28171, .T. ) ;
#37427=( LENGTH_UNIT ( ) NAMED_UNIT ( * ) SI_UNIT ( .MILLI., .METRE. ) );
#37428=EDGE_LOOP ( 'NONE', ( #55866, #89257, #464, #47897 ) ) ;
#37431=CARTESIAN_POINT ( 'NONE',  ( 7.007893109692266087, -58.32153039260716554, 4.000000000000000000 ) ) ;
#37465=CARTESIAN_POINT ( 'NONE',  ( 4.219999999999999751, 10.25000000000000000, 2.500000000000000000 ) ) ;
#37477=PRODUCT_DEFINITION_CONTEXT ( 'detailed design', #25126, 'design' ) ;
#37478=CARTESIAN_POINT ( 'NONE',  ( -8.665245649996185406, 87.00799529562631562, 4.320095926137915932 ) ) ;
#37483=CARTESIAN_POINT ( 'NONE',  ( 8.879999999999991900, 21.00000000000000000, -2.900000000000000799 ) ) ;
#37485=CARTESIAN_POINT ( 'NONE',  ( 6.533420211785746723, -50.31490269211863620, -3.750000000000000888 ) ) ;
#37505=CARTESIAN_POINT ( 'NONE',  ( -6.430724159521292727, -88.51069574204372259, 4.000000000000000000 ) ) ;
#37528=( NAMED_UNIT ( * ) SI_UNIT ( $, .STERADIAN. ) SOLID_ANGLE_UNIT ( ) );
#37542=CARTESIAN_POINT ( 'NONE',  ( -8.000000000000000000, 1.019547802438458550, 4.000000000000000000 ) ) ;
#37544=CARTESIAN_POINT ( 'NONE',  ( -6.982525766850296023, -88.11956318484570261, -4.000000000000000000 ) ) ;
#37552=CARTESIAN_POINT ( 'NONE',  ( -10.03950393934837670, 88.95408272063291122, -5.473102654076496876 ) ) ;
#37570=VECTOR ( 'NONE', #42592, 1000.000000000000000 ) ;
#37577=VERTEX_POINT ( 'NONE', #13111 ) ;
#37585=CARTESIAN_POINT ( 'NONE',  ( 10.69983265767916514, -97.11219342806609234, 3.999999999999999112 ) ) ;
#37591=DIRECTION ( 'NONE',  ( -0.000000000000000000, 0.000000000000000000, 1.000000000000000000 ) ) ;
#37605=CARTESIAN_POINT ( 'NONE',  ( 12.24319267753454099, 54.01141590572476048, 2.899999999999999467 ) ) ;
#37606=ADVANCED_FACE ( 'NONE', ( #44090 ), #82098, .F. ) ;
#37609=ORIENTED_EDGE ( 'NONE', *, *, #44829, .F. ) ;
#37612=VERTEX_POINT ( 'NONE', #60585 ) ;
#37618=LINE ( 'NONE', #13619, #11278 ) ;
#37625=LINE ( 'NONE', #90602, #33994 ) ;
#37628=AXIS2_PLACEMENT_3D ( 'NONE', #81125, #88130, #3670 ) ;
#37629=PLANE ( 'NONE',  #94318 ) ;
#37652=LINE ( 'NONE', #74648, #40171 ) ;
#37656=CIRCLE ( 'NONE', #50411, 0.2500000000000002220 ) ;
#37662=CARTESIAN_POINT ( 'NONE',  ( -8.159331231749115787, -4.163042900881196218, 3.750000000000000000 ) ) ;
#37668=PRESENTATION_STYLE_ASSIGNMENT (( #29642 ) ) ;
#37672=VERTEX_POINT ( 'NONE', #37605 ) ;
#37673=DIRECTION ( 'NONE',  ( 1.000000000000000000, 0.000000000000000000, 0.000000000000000000 ) ) ;
#37675=( NAMED_UNIT ( * ) SI_UNIT ( $, .STERADIAN. ) SOLID_ANGLE_UNIT ( ) );
#37678=LINE ( 'NONE', #30145, #90373 ) ;
#37687=( GEOMETRIC_REPRESENTATION_CONTEXT ( 3 ) GLOBAL_UNCERTAINTY_ASSIGNED_CONTEXT ( ( #27153 ) ) GLOBAL_UNIT_ASSIGNED_CONTEXT ( ( #5641, #42166, #4661 ) ) REPRESENTATION_CONTEXT ( 'NONE', 'WORKASPACE' ) );
#37689=ORIENTED_EDGE ( 'NONE', *, *, #58130, .T. ) ;
#37704=ORIENTED_EDGE ( 'NONE', *, *, #1732, .T. ) ;
#37712=CARTESIAN_POINT ( 'NONE',  ( 7.850000000000003197, 98.49999999999998579, -8.525133428036873795 ) ) ;
#37713=CARTESIAN_POINT ( 'NONE',  ( -6.581680125707233486, -88.31141629936868753, -2.750000000000000000 ) ) ;
#37717=LINE ( 'NONE', #67722, #22446 ) ;
#37725=DIRECTION ( 'NONE',  ( -0.06975647374412544122, -0.9975640502598241977, 0.000000000000000000 ) ) ;
#37729=ORIENTED_EDGE ( 'NONE', *, *, #19659, .F. ) ;
#37733=ADVANCED_FACE ( 'NONE', ( #21618 ), #14113, .F. ) ;
#37734=ORIENTED_EDGE ( 'NONE', *, *, #80127, .F. ) ;
#37741=DIRECTION ( 'NONE',  ( 0.8070303256584298035, -0.5905099943842175847, 0.000000000000000000 ) ) ;
#37743=LINE ( 'NONE', #14246, #13688 ) ;
#37757=TOROIDAL_SURFACE ( 'NONE', #23417, 0.5000000000000000000, 0.2500000000000000000 ) ;
#37762=CARTESIAN_POINT ( 'NONE',  ( 0.000000000000000000, -97.00000000000000000, -3.750000000000000000 ) ) ;
#37768=CARTESIAN_POINT ( 'NONE',  ( 11.29392812321118100, -89.88967135473500036, -3.750000000000000000 ) ) ;
#37769=DIRECTION ( 'NONE',  ( 0.6246950475544238435, 0.7808688094430307203, 0.000000000000000000 ) ) ;
#37795=( NAMED_UNIT ( * ) SI_UNIT ( $, .STERADIAN. ) SOLID_ANGLE_UNIT ( ) );
#37805=SURFACE_STYLE_USAGE ( .BOTH. , #60289 ) ;
#37806=VECTOR ( 'NONE', #49768, 1000.000000000000000 ) ;
#37808=STYLED_ITEM ( 'NONE', ( #85265 ), #17991 ) ;
#37810=VERTEX_POINT ( 'NONE', #73604 ) ;
#37815=EDGE_CURVE ( 'NONE', #70878, #83825, #5129, .T. ) ;
#37816=DIRECTION ( 'NONE',  ( 0.000000000000000000, 1.000000000000000000, 0.000000000000000000 ) ) ;
#37819=SURFACE_SIDE_STYLE ('',( #75798 ) ) ;
#37826=COLOUR_RGB ( '', 0.09019608, 0.27058824, 0.51372549) ;
#37852=CARTESIAN_POINT ( 'NONE',  ( 6.574584770565365055, -50.88238473842167053, -2.749999999998390177 ) ) ;
#37855=EDGE_CURVE ( 'NONE', #28474, #44602, #52157, .T. ) ;
#37856=CARTESIAN_POINT ( 'NONE',  ( 1.379999999999981908, 20.99999999999999645, 1.249999999999987121 ) ) ;
#37869=CARTESIAN_POINT ( 'NONE',  ( -8.081452932198143202, -7.288464344205941359, -4.000000000000000000 ) ) ;
#37872=CARTESIAN_POINT ( 'NONE',  ( 6.579634127946654587, -87.99828267815715321, 3.750000000000000000 ) ) ;
#37884=DIRECTION ( 'NONE',  ( -1.000000000000000000, 0.000000000000000000, 0.000000000000000000 ) ) ;
#37886=CARTESIAN_POINT ( 'NONE',  ( -8.957305892841448625, -19.72688805321238448, -4.000000000000000000 ) ) ;
#37901=CIRCLE ( 'NONE', #68228, 0.2500000000000002220 ) ;
#37917=VERTEX_POINT ( 'NONE', #24081 ) ;
#37921=FILL_AREA_STYLE_COLOUR ( '', #95148 ) ;
#37925=CARTESIAN_POINT ( 'NONE',  ( 5.115475850225431387, -17.53855045868316154, 4.000000000004829914 ) ) ;
#37952=ORIENTED_EDGE ( 'NONE', *, *, #10801, .F. ) ;
#37958=AXIS2_PLACEMENT_3D ( 'NONE', #95905, #6359, #59851 ) ;
#37961=DIRECTION ( 'NONE',  ( 0.000000000000000000, 0.000000000000000000, -1.000000000000000000 ) ) ;
#37963=VECTOR ( 'NONE', #39687, 1000.000000000000000 ) ;
#37965=DIRECTION ( 'NONE',  ( 1.000000000000000000, -0.000000000000000000, 0.000000000000000000 ) ) ;
#37968=AXIS2_PLACEMENT_3D ( 'NONE', #29280, #59776, #90269 ) ;
#37969=CARTESIAN_POINT ( 'NONE',  ( 7.850000000000003197, 98.49999999999998579, 8.000000000000000000 ) ) ;
#37980=LINE ( 'NONE', #37483, #89301 ) ;
#37996=DIRECTION ( 'NONE',  ( 1.000000000000000000, 0.000000000000000000, 0.000000000000000000 ) ) ;
#38009=EDGE_LOOP ( 'NONE', ( #809, #86714, #87596, #3055 ) ) ;
#38010=ADVANCED_FACE ( 'NONE', ( #84085 ), #2084, .T. ) ;
#38021=EDGE_LOOP ( 'NONE', ( #12349, #88843, #80903, #38246, #42500, #22083 ) ) ;
#38029=VECTOR ( 'NONE', #4139, 999.9999999999998863 ) ;
#38036=CIRCLE ( 'NONE', #98720, 0.2500000000000002220 ) ;
#38038=CARTESIAN_POINT ( 'NONE',  ( -7.080143328648153656, -69.54337233422633346, -3.749999999999999556 ) ) ;
#38055=ORIENTED_EDGE ( 'NONE', *, *, #63417, .F. ) ;
#38057=VERTEX_POINT ( 'NONE', #91078 ) ;
#38073=ORIENTED_EDGE ( 'NONE', *, *, #1499, .F. ) ;
#38078=ADVANCED_FACE ( 'NONE', ( #9066 ), #37757, .T. ) ;
#38079=DIRECTION ( 'NONE',  ( 0.000000000000000000, 1.000000000000000000, 0.000000000000000000 ) ) ;
#38083=CARTESIAN_POINT ( 'NONE',  ( 8.650320195642805743, -1.048895414480025323, 4.000000000000000000 ) ) ;
#38092=MECHANICAL_DESIGN_GEOMETRIC_PRESENTATION_REPRESENTATION('',(#68426),#25466);
#38097=PRESENTATION_STYLE_ASSIGNMENT (( #38578 ) ) ;
#38099=ORIENTED_EDGE ( 'NONE', *, *, #50212, .T. ) ;
#38104=CIRCLE ( 'NONE', #55649, 0.2500000000000002220 ) ;
#38107=CYLINDRICAL_SURFACE ( 'NONE', #38804, 2.000000000000000888 ) ;
#38116=CARTESIAN_POINT ( 'NONE',  ( -7.081429851441987999, -84.79152421822192309, -2.750000000000000444 ) ) ;
#38119=EDGE_CURVE ( 'NONE', #35357, #25656, #96932, .T. ) ;
#38134=UNCERTAINTY_MEASURE_WITH_UNIT (LENGTH_MEASURE( 1.000000000000000082E-05 ), #12870, 'distance_accuracy_value', 'NONE');
#38143=DIRECTION ( 'NONE',  ( 1.000000000000000000, 0.000000000000000000, 0.000000000000000000 ) ) ;
#38159=CARTESIAN_POINT ( 'NONE',  ( -11.60563658639003037, -81.99692803277919495, 3.750000000000000000 ) ) ;
#38167=TOROIDAL_SURFACE ( 'NONE', #3050, 10.65000000000026326, 0.2500000000000000000 ) ;
#38170=DIRECTION ( 'NONE',  ( -0.000000000000000000, 1.000000000000000000, 4.510281037539694028E-14 ) ) ;
#38172=EDGE_LOOP ( 'NONE', ( #46183, #91151, #74053, #78854 ) ) ;
#38173=CARTESIAN_POINT ( 'NONE',  ( -4.249999999999994671, 43.00000000000000000, 6.250000000000000000 ) ) ;
#38178=CYLINDRICAL_SURFACE ( 'NONE', #83803, 0.2500000000000002220 ) ;
#38181=EDGE_CURVE ( 'NONE', #6552, #18240, #56053, .T. ) ;
#38198=STYLED_ITEM ( 'NONE', ( #45069 ), #26526 ) ;
#38203=SURFACE_STYLE_FILL_AREA ( #45689 ) ;
#38207=EDGE_CURVE ( 'NONE', #27291, #39290, #41034, .T. ) ;
#38246=ORIENTED_EDGE ( 'NONE', *, *, #68592, .T. ) ;
#38251=FACE_OUTER_BOUND ( 'NONE', #81420, .T. ) ;
#38257=CARTESIAN_POINT ( 'NONE',  ( 10.83696084481538691, -98.17058944465519232, -3.750000000000000000 ) ) ;
#38259=AXIS2_PLACEMENT_3D ( 'NONE', #93123, #18616, #40138 ) ;
#38283=( NAMED_UNIT ( * ) PLANE_ANGLE_UNIT ( ) SI_UNIT ( $, .RADIAN. ) );
#38286=CARTESIAN_POINT ( 'NONE',  ( -3.500000000000000444, 1.019547802438453887, 3.750000000000000000 ) ) ;
#38304=VERTEX_POINT ( 'NONE', #41555 ) ;
#38308=FILL_AREA_STYLE ('',( #7813 ) ) ;
#38313=DIRECTION ( 'NONE',  ( 1.000000000000000000, 0.000000000000000000, 0.000000000000000000 ) ) ;
#38330=COLOUR_RGB ( '', 0.08235294, 0.09019608, 0.10196078) ;
#38339=CARTESIAN_POINT ( 'NONE',  ( 4.130000001237588592, 0.09091675484614469838, -2.500000000000000000 ) ) ;
#38343=CARTESIAN_POINT ( 'NONE',  ( 4.441302488725760611, -2.692589364095749005, 2.750000000000000888 ) ) ;
#38350=AXIS2_PLACEMENT_3D ( 'NONE', #80265, #72266, #43244 ) ;
#38357=EDGE_CURVE ( 'NONE', #68676, #64082, #7523, .T. ) ;
#38393=VECTOR ( 'NONE', #61957, 1000.000000000000000 ) ;
#38399=VERTEX_POINT ( 'NONE', #66493 ) ;
#38400=ADVANCED_FACE ( 'NONE', ( #90462 ), #12992, .T. ) ;
#38401=AXIS2_PLACEMENT_3D ( 'NONE', #4008, #5486, #28465 ) ;
#38406=ORIENTED_EDGE ( 'NONE', *, *, #95242, .F. ) ;
#38432=ORIENTED_EDGE ( 'NONE', *, *, #44531, .T. ) ;
#38450=ORIENTED_EDGE ( 'NONE', *, *, #11246, .T. ) ;
#38451=COLOUR_RGB ( '', 0.40784314, 0.44705882, 0.49803922) ;
#38458=TOROIDAL_SURFACE ( 'NONE', #67212, 11.15000000000026326, 0.2500000000000000000 ) ;
#38459=FACE_OUTER_BOUND ( 'NONE', #78717, .T. ) ;
#38461=VECTOR ( 'NONE', #30490, 1000.000000000000000 ) ;
#38508=SURFACE_SIDE_STYLE ('',( #68018 ) ) ;
#38510=ORIENTED_EDGE ( 'NONE', *, *, #427, .T. ) ;
#38524=CARTESIAN_POINT ( 'NONE',  ( -6.031993939728319987, -39.82530731229964971, -4.000000000000000000 ) ) ;
#38532=CARTESIAN_POINT ( 'NONE',  ( -8.000343251535921851, 84.06932101904432386, -3.750000000000000000 ) ) ;
#38538=FILL_AREA_STYLE ('',( #55506 ) ) ;
#38564=MECHANICAL_DESIGN_GEOMETRIC_PRESENTATION_REPRESENTATION('',(#46543),#8231);
#38571=ORIENTED_EDGE ( 'NONE', *, *, #51544, .F. ) ;
#38578=SURFACE_STYLE_USAGE ( .BOTH. , #47549 ) ;
#38588=CARTESIAN_POINT ( 'NONE',  ( -7.750000000000000000, 83.99999999999994316, -4.000000000000000000 ) ) ;
#38589=AXIS2_PLACEMENT_3D ( 'NONE', #7637, #90607, #61098 ) ;
#38598=CARTESIAN_POINT ( 'NONE',  ( -5.812563760649267941, -35.09659463721938977, -2.750000000000000444 ) ) ;
#38600=CARTESIAN_POINT ( 'NONE',  ( -8.924603092375777535, 75.06466731010172566, -3.000000000000000000 ) ) ;
#38628=( LENGTH_UNIT ( ) NAMED_UNIT ( * ) SI_UNIT ( .MILLI., .METRE. ) );
#38630=SURFACE_STYLE_FILL_AREA ( #31603 ) ;
#38632=ORIENTED_EDGE ( 'NONE', *, *, #8576, .F. ) ;
#38640=CARTESIAN_POINT ( 'NONE',  ( -11.30179204363884082, -57.06033576789361206, 4.000000000000000000 ) ) ;
#38659=SURFACE_STYLE_USAGE ( .BOTH. , #16154 ) ;
#38666=CIRCLE ( 'NONE', #94537, 10.65000000000000036 ) ;
#38669=CIRCLE ( 'NONE', #8331, 0.7500000000000006661 ) ;
#38671=ORIENTED_EDGE ( 'NONE', *, *, #75522, .T. ) ;
#38678=CARTESIAN_POINT ( 'NONE',  ( -6.787878914541003006, -86.25326249609904039, 2.499999999999999556 ) ) ;
#38685=FACE_OUTER_BOUND ( 'NONE', #6080, .T. ) ;
#38687=B_SPLINE_SURFACE_WITH_KNOTS ( 'NONE', 3, 1, ( 
 ( #18699, #41702 ),
 ( #80168, #42189 ),
 ( #43154, #35149 ),
 ( #18207, #26673 ),
 ( #95672, #11680 ),
 ( #4686, #73641 ),
 ( #26193, #65649 ),
 ( #72653, #50160 ),
 ( #96172, #95166 ),
 ( #27159, #94185 ),
 ( #3701, #4188 ),
 ( #88651, #34658 ),
 ( #86702, #3207 ),
 ( #34161, #19178 ),
 ( #57167, #87664 ),
 ( #79684, #87177 ),
 ( #58142, #33670 ),
 ( #64653, #48687 ) ),
 .UNSPECIFIED., .F., .F., .F.,
 ( 4, 2, 2, 2, 2, 2, 2, 2, 4 ),
 ( 2, 2 ),
 ( 0.1401766717507622606, 0.2499999999999989453, 0.3749999999999986122, 0.4374999999999986677, 0.4999999999999986677, 0.7499999999999992228, 0.8749999999999996669, 0.9374999999999997780, 1.000000000000000000 ),
 ( 0.000000000000000000, 1.000000000000000000 ),
 .UNSPECIFIED. ) ;
#38688=CARTESIAN_POINT ( 'NONE',  ( 8.880000000000000782, -0.01162444801151916833, 3.750000000006731060 ) ) ;
#38707=EDGE_LOOP ( 'NONE', ( #25529, #19329, #33237, #71807 ) ) ;
#38709=ORIENTED_EDGE ( 'NONE', *, *, #15078, .F. ) ;
#38714=CARTESIAN_POINT ( 'NONE',  ( 9.879999999999990123, 20.99999999999999645, 0.000000000000000000 ) ) ;
#38718=DIRECTION ( 'NONE',  ( -0.000000000000000000, -0.000000000000000000, -1.000000000000000000 ) ) ;
#38731=ORIENTED_EDGE ( 'NONE', *, *, #76887, .F. ) ;
#38739=( GEOMETRIC_REPRESENTATION_CONTEXT ( 3 ) GLOBAL_UNCERTAINTY_ASSIGNED_CONTEXT ( ( #51284 ) ) GLOBAL_UNIT_ASSIGNED_CONTEXT ( ( #1583, #1088, #8570 ) ) REPRESENTATION_CONTEXT ( 'NONE', 'WORKASPACE' ) );
#38743=ORIENTED_EDGE ( 'NONE', *, *, #61633, .T. ) ;
#38746=CARTESIAN_POINT ( 'NONE',  ( 11.04808542157948992, -95.57857389791176672, -3.750000000000000000 ) ) ;
#38753=FILL_AREA_STYLE_COLOUR ( '', #32001 ) ;
#38757=AXIS2_PLACEMENT_3D ( 'NONE', #7260, #59249, #98779 ) ;
#38760=CARTESIAN_POINT ( 'NONE',  ( 8.879999999999991900, 76.07179676972447169, -4.250000000000000000 ) ) ;
#38761=FACE_OUTER_BOUND ( 'NONE', #84397, .T. ) ;
#38769=CARTESIAN_POINT ( 'NONE',  ( 18.00000000000000000, 78.68095262110993815, 3.967704011867259517 ) ) ;
#38774=ORIENTED_EDGE ( 'NONE', *, *, #45616, .T. ) ;
#38776=( BOUNDED_CURVE ( )  B_SPLINE_CURVE ( 3, ( #26222, #88683, #73672, #89180 ),
 .UNSPECIFIED., .F., .T. ) 
 B_SPLINE_CURVE_WITH_KNOTS ( ( 4, 4 ),
 ( 4.712388980384689674, 6.283185307179586232 ),
 .UNSPECIFIED. ) 
 CURVE ( )  GEOMETRIC_REPRESENTATION_ITEM ( )  RATIONAL_B_SPLINE_CURVE ( ( 1.000000000000000000, 0.8047378541243649375, 0.8047378541243649375, 1.000000000000000000 ) ) 
 REPRESENTATION_ITEM ( '' )  );
#38785=CIRCLE ( 'NONE', #42000, 0.2500000000000002220 ) ;
#38789=ORIENTED_EDGE ( 'NONE', *, *, #49339, .T. ) ;
#38790=( NAMED_UNIT ( * ) SI_UNIT ( $, .STERADIAN. ) SOLID_ANGLE_UNIT ( ) );
#38791=ORIENTED_EDGE ( 'NONE', *, *, #88589, .T. ) ;
#38804=AXIS2_PLACEMENT_3D ( 'NONE', #14116, #7613, #36108 ) ;
#38808=VECTOR ( 'NONE', #29454, 1000.000000000000000 ) ;
#38829=CARTESIAN_POINT ( 'NONE',  ( 6.933985542720472850, -73.15302115696529484, -2.750000000000000444 ) ) ;
#38846=CARTESIAN_POINT ( 'NONE',  ( -8.897294703554354811, -15.56348197609296058, -3.750000000000000000 ) ) ;
#38848=AXIS2_PLACEMENT_3D ( 'NONE', #54647, #93145, #92652 ) ;
#38853=ADVANCED_FACE ( 'NONE', ( #63418 ), #41440, .F. ) ;
#38864=CARTESIAN_POINT ( 'NONE',  ( -8.900000000000002132, 83.99999999999994316, 0.000000000000000000 ) ) ;
#38876=CYLINDRICAL_SURFACE ( 'NONE', #13229, 0.2500000000000002220 ) ;
#38896=VERTEX_POINT ( 'NONE', #63894 ) ;
#38899=VERTEX_POINT ( 'NONE', #55931 ) ;
#38904=CARTESIAN_POINT ( 'NONE',  ( 6.034747819266367053, -36.07388523691940918, 3.999999999999999556 ) ) ;
#38909=CARTESIAN_POINT ( 'NONE',  ( -3.878335320991981305, -3.629921146508663821, -4.000000000000000000 ) ) ;
#38922=EDGE_CURVE ( 'NONE', #72511, #12076, #52824, .T. ) ;
#38929=B_SPLINE_CURVE_WITH_KNOTS ( 'NONE', 3,
 ( #69326, #62793, #93786, #38343, #847, #55801, #62293, #68838, #30818, #1832, #61316, #23345, #31305, #61807, #11762, #26268, #42270, #73239 ),
 .UNSPECIFIED., .F., .F.,
 ( 4, 2, 2, 2, 2, 2, 2, 2, 4 ),
 ( 2.168404344971008868E-18, 0.002783570816222668415, 0.005567141632445335095, 0.01113428326489066672, 0.02226856652978132997, 0.04453713305956264606, 0.06680569958934397257, 0.07793998285423464623, 0.08907426611912530601 ),
 .UNSPECIFIED. ) ;
#38934=DIRECTION ( 'NONE',  ( 0.000000000000000000, 0.000000000000000000, -1.000000000000000000 ) ) ;
#38942=ORIENTED_EDGE ( 'NONE', *, *, #77550, .F. ) ;
#38948=CIRCLE ( 'NONE', #94824, 3.000000000000002665 ) ;
#38955=CARTESIAN_POINT ( 'NONE',  ( 4.130000001237588592, 0.09091675483695403626, 2.500000000000000000 ) ) ;
#38959=CARTESIAN_POINT ( 'NONE',  ( 6.829574850505127692, -88.00372650098204019, -3.749999999999998668 ) ) ;
#38967=ADVANCED_FACE ( 'NONE', ( #51868 ), #59237, .T. ) ;
#38973=CYLINDRICAL_SURFACE ( 'NONE', #19537, 0.2500000000000002220 ) ;
#38977=SURFACE_STYLE_USAGE ( .BOTH. , #54449 ) ;
#38981=DIRECTION ( 'NONE',  ( -1.000000000000000000, 0.000000000000000000, 0.000000000000000000 ) ) ;
#39009=CARTESIAN_POINT ( 'NONE',  ( 4.219999999999999751, 37.25000000000000000, 4.000000000000000000 ) ) ;
#39013=ORIENTED_EDGE ( 'NONE', *, *, #55858, .T. ) ;
#39023=AXIS2_PLACEMENT_3D ( 'NONE', #36476, #5497, #88981 ) ;
#39033=ORIENTED_EDGE ( 'NONE', *, *, #13086, .T. ) ;
#39034=DIRECTION ( 'NONE',  ( -0.08715574274766037244, -0.9961946980917453232, -0.000000000000000000 ) ) ;
#39043=ORIENTED_EDGE ( 'NONE', *, *, #9128, .F. ) ;
#39050=ORIENTED_EDGE ( 'NONE', *, *, #45977, .T. ) ;
#39060=ADVANCED_FACE ( 'NONE', ( #35379 ), #73650, .T. ) ;
#39063=ORIENTED_EDGE ( 'NONE', *, *, #26997, .F. ) ;
#39066=ORIENTED_EDGE ( 'NONE', *, *, #83639, .T. ) ;
#39080=CARTESIAN_POINT ( 'NONE',  ( -7.749999999999996447, 83.99999999999994316, -3.750000000000000000 ) ) ;
#39082=CARTESIAN_POINT ( 'NONE',  ( 8.879999999999991900, 27.04366094290857347, -2.900000000000000799 ) ) ;
#39083=ADVANCED_FACE ( 'NONE', ( #74350 ), #94434, .T. ) ;
#39096=CARTESIAN_POINT ( 'NONE',  ( 5.129999999999991900, 76.07179676972444327, -6.500000000000000888 ) ) ;
#39102=VECTOR ( 'NONE', #33267, 1000.000000000000000 ) ;
#39112=VECTOR ( 'NONE', #12764, 1000.000000000000000 ) ;
#39118=ORIENTED_EDGE ( 'NONE', *, *, #87589, .T. ) ;
#39120=B_SPLINE_CURVE_WITH_KNOTS ( 'NONE', 3,
 ( #79621, #36083, #42125, #4125, #51086, #80606 ),
 .UNSPECIFIED., .F., .F.,
 ( 4, 2, 4 ),
 ( 0.000000000000000000, 0.0008870672566257227975, 0.001774134513251445595 ),
 .UNSPECIFIED. ) ;
#39122=CARTESIAN_POINT ( 'NONE',  ( 8.879999999999991900, 27.04366094290857703, 2.958578643762690863 ) ) ;
#39123=EDGE_CURVE ( 'NONE', #88822, #44602, #16334, .T. ) ;
#39131=MECHANICAL_DESIGN_GEOMETRIC_PRESENTATION_REPRESENTATION('',(#67823),#23147);
#39139=CARTESIAN_POINT ( 'NONE',  ( -9.206628575834976402, -19.70849028575129935, 3.750000000000000000 ) ) ;
#39152=PRESENTATION_STYLE_ASSIGNMENT (( #32109 ) ) ;
#39174=CARTESIAN_POINT ( 'NONE',  ( 8.629999999999995453, 43.00000000000000000, 6.250000000000000000 ) ) ;
#39181=CARTESIAN_POINT ( 'NONE',  ( -3.500000001558553286, 0.09224605988771300558, 2.499999999999595879 ) ) ;
#39183=CARTESIAN_POINT ( 'NONE',  ( 8.705946125150790138, -3.115782928412242025, 4.000000000000000000 ) ) ;
#39190=LINE ( 'NONE', #37712, #69994 ) ;
#39195=PRESENTATION_STYLE_ASSIGNMENT (( #54174 ) ) ;
#39201=CARTESIAN_POINT ( 'NONE',  ( 5.114679605276696073, -17.52310038222973887, -2.750000000000000444 ) ) ;
#39202=ORIENTED_EDGE ( 'NONE', *, *, #12330, .T. ) ;
#39222=B_SPLINE_CURVE_WITH_KNOTS ( 'NONE', 3,
 ( #45440, #98481, #90434, #54411, #7467, #77404, #29440, #75448, #53430, #59944, #29937, #22462, #15939, #15466, #950, #52938, #83448, #68944 ),
 .UNSPECIFIED., .F., .F.,
 ( 4, 2, 2, 2, 2, 2, 2, 2, 4 ),
 ( 0.000000000000000000, 0.01113267275063152192, 0.02226534550126304385, 0.04453069100252608770, 0.06679603650378912461, 0.07792870925442065000, 0.08349504562973641963, 0.08627821381739429751, 0.08906138200505217539 ),
 .UNSPECIFIED. ) ;
#39230=AXIS2_PLACEMENT_3D ( 'NONE', #74847, #28839, #6347 ) ;
#39255=UNCERTAINTY_MEASURE_WITH_UNIT (LENGTH_MEASURE( 1.000000000000000082E-05 ), #41171, 'distance_accuracy_value', 'NONE');
#39257=VERTEX_POINT ( 'NONE', #7854 ) ;
#39258=DIRECTION ( 'NONE',  ( 0.7808688094430307203, -0.6246950475544238435, 0.000000000000000000 ) ) ;
#39279=( GEOMETRIC_REPRESENTATION_CONTEXT ( 3 ) GLOBAL_UNCERTAINTY_ASSIGNED_CONTEXT ( ( #48325 ) ) GLOBAL_UNIT_ASSIGNED_CONTEXT ( ( #60221, #76700, #59723 ) ) REPRESENTATION_CONTEXT ( 'NONE', 'WORKASPACE' ) );
#39284=EDGE_LOOP ( 'NONE', ( #85116, #77134, #91780, #92800 ) ) ;
#39286=CARTESIAN_POINT ( 'NONE',  ( -4.249999999999994671, 43.00000000000000711, -6.500000000000000888 ) ) ;
#39287=ORIENTED_EDGE ( 'NONE', *, *, #72463, .T. ) ;
#39290=VERTEX_POINT ( 'NONE', #21876 ) ;
#39295=CARTESIAN_POINT ( 'NONE',  ( 12.99999999999999822, 75.00000000000000000, 6.500000000000000888 ) ) ;
#39298=EDGE_CURVE ( 'NONE', #34829, #70878, #52354, .T. ) ;
#39299=AXIS2_PLACEMENT_3D ( 'NONE', #1945, #41424, #55414 ) ;
#39304=VECTOR ( 'NONE', #54157, 1000.000000000000000 ) ;
#39314=DIRECTION ( 'NONE',  ( -0.1496197561345335991, 0.9887436111420608853, 1.038195613746000465E-15 ) ) ;
#39320=CARTESIAN_POINT ( 'NONE',  ( -10.80370554825985430, 89.74834511847251406, 6.353281608588779328 ) ) ;
#39324=ORIENTED_EDGE ( 'NONE', *, *, #18631, .T. ) ;
#39325=( NAMED_UNIT ( * ) SI_UNIT ( $, .STERADIAN. ) SOLID_ANGLE_UNIT ( ) );
#39338=SURFACE_STYLE_FILL_AREA ( #46817 ) ;
#39340=CARTESIAN_POINT ( 'NONE',  ( -11.16008302858703694, -52.90628376244900011, -3.999999999996394440 ) ) ;
#39347=SURFACE_SIDE_STYLE ('',( #31327 ) ) ;
#39348=DIRECTION ( 'NONE',  ( -0.000000000000000000, -0.000000000000000000, 1.000000000000000000 ) ) ;
#39362=CARTESIAN_POINT ( 'NONE',  ( 8.879999999999991900, 69.99999999999998579, 6.250000000000000000 ) ) ;
#39383=EDGE_CURVE ( 'NONE', #48651, #47034, #89651, .T. ) ;
#39393=ORIENTED_EDGE ( 'NONE', *, *, #29003, .F. ) ;
#39396=CARTESIAN_POINT ( 'NONE',  ( 6.934035614042552531, -73.16521313705239038, 3.999999999998390177 ) ) ;
#39397=FACE_OUTER_BOUND ( 'NONE', #26129, .T. ) ;
#39416=EDGE_CURVE ( 'NONE', #98330, #69208, #9794, .T. ) ;
#39421=ORIENTED_EDGE ( 'NONE', *, *, #74804, .T. ) ;
#39431=DIRECTION ( 'NONE',  ( 0.9975640502598257520, -0.06975647374410356982, 0.000000000000000000 ) ) ;
#39437=( BOUNDED_SURFACE ( )  B_SPLINE_SURFACE ( 3, 2, ( 
 ( #18150, #63138, #17663 ),
 ( #39679, #39181, #78149 ),
 ( #69670, #40155, #70170 ),
 ( #24178, #16674, #86642 ),
 ( #57969, #1686, #85165 ),
 ( #94624, #47146, #48624 ),
 ( #70661, #93640, #10156 ),
 ( #31657, #79128, #32139 ),
 ( #27476, #55654, #88475 ),
 ( #55140, #78650, #41154 ),
 ( #40651, #71150, #85654 ),
 ( #33612, #90430, #20981 ),
 ( #96993, #36963, #29932 ),
 ( #12966, #51966, #59940 ),
 ( #5974, #90930, #67954 ),
 ( #81462, #67458, #74950 ),
 ( #36467, #13973, #73461 ),
 ( #20481, #4989, #12477 ),
 ( #42981, #88973, #82450 ),
 ( #29435, #50968, #73962 ),
 ( #66962, #14464, #98477 ),
 ( #74447, #22458, #35470 ) ),
 .UNSPECIFIED., .F., .F., .F. ) 
 B_SPLINE_SURFACE_WITH_KNOTS ( ( 4, 2, 2, 2, 2, 2, 2, 2, 2, 2, 4 ),
 ( 3, 3 ),
 ( 0.000000000000000000, 0.002788823349942589833, 0.005577646699885179665, 0.01115529339977035933, 0.02231058679954071866, 0.03346588019931107799, 0.04462117359908143732, 0.06693176039862215598, 0.07808705379839250837, 0.08366470049827769151, 0.08924234719816287464 ),
 ( 0.000000000000000000, 1.000000000000000000 ),
 .UNSPECIFIED. ) 
 GEOMETRIC_REPRESENTATION_ITEM ( )  RATIONAL_B_SPLINE_SURFACE ( (
 ( 1.000000000000000000, 0.7071067811865475727, 1.000000000000000000),
 ( 1.000000000000000000, 0.7071067811865475727, 1.000000000000000000),
 ( 1.000000000000000000, 0.7071067811865482389, 1.000000000000000000),
 ( 1.000000000000000000, 0.7071067811865482389, 1.000000000000000000),
 ( 1.000000000000000000, 0.7071067811865482389, 1.000000000000000000),
 ( 1.000000000000000000, 0.7071067811865482389, 1.000000000000000000),
 ( 1.000000000000000000, 0.7071067811865487940, 1.000000000000000000),
 ( 1.000000000000000000, 0.7071067811865487940, 1.000000000000000000),
 ( 1.000000000000000000, 0.7071067811865477948, 1.000000000000000000),
 ( 1.000000000000000000, 0.7071067811865477948, 1.000000000000000000),
 ( 1.000000000000000000, 0.7071067811865493491, 1.000000000000000000),
 ( 1.000000000000000000, 0.7071067811865493491, 1.000000000000000000),
 ( 1.000000000000000000, 0.7071067811865473507, 1.000000000000000000),
 ( 1.000000000000000000, 0.7071067811865473507, 1.000000000000000000),
 ( 1.000000000000000000, 0.7071067811865482389, 1.000000000000000000),
 ( 1.000000000000000000, 0.7071067811865482389, 1.000000000000000000),
 ( 1.000000000000000000, 0.7071067811865482389, 1.000000000000000000),
 ( 1.000000000000000000, 0.7071067811865482389, 1.000000000000000000),
 ( 1.000000000000000000, 0.7071067811865482389, 1.000000000000000000),
 ( 1.000000000000000000, 0.7071067811865482389, 1.000000000000000000),
 ( 1.000000000000000000, 0.7071067811865482389, 1.000000000000000000),
 ( 1.000000000000000000, 0.7071067811865482389, 1.000000000000000000) ) ) 
 REPRESENTATION_ITEM ( '' )  SURFACE ( )  );
#39452=CARTESIAN_POINT ( 'NONE',  ( 4.919406150870956118, -13.80316667505430495, 2.750000000000000000 ) ) ;
#39466=VERTEX_POINT ( 'NONE', #25804 ) ;
#39468=DIRECTION ( 'NONE',  ( 0.000000000000000000, 0.000000000000000000, 1.000000000000000000 ) ) ;
#39473=PRESENTATION_STYLE_ASSIGNMENT (( #38977 ) ) ;
#39475=CARTESIAN_POINT ( 'NONE',  ( 4.630000000000001670, 1.019547802438464545, -4.000000000000000000 ) ) ;
#39477=LINE ( 'NONE', #69967, #91810 ) ;
#39485=DIRECTION ( 'NONE',  ( 0.000000000000000000, 1.000000000000000000, 0.000000000000000000 ) ) ;
#39513=ORIENTED_EDGE ( 'NONE', *, *, #1773, .F. ) ;
#39532=CIRCLE ( 'NONE', #1295, 10.90000000000000036 ) ;
#39541=EDGE_CURVE ( 'NONE', #15515, #87018, #5012, .T. ) ;
#39544=ORIENTED_EDGE ( 'NONE', *, *, #83264, .T. ) ;
#39564=EDGE_CURVE ( 'NONE', #20729, #22610, #97609, .T. ) ;
#39567=TOROIDAL_SURFACE ( 'NONE', #9226, 2.899999999999999467, 0.1000000000000000056 ) ;
#39568=DIRECTION ( 'NONE',  ( 1.049065152435176504E-16, -1.000000000000000000, 0.000000000000000000 ) ) ;
#39583=ORIENTED_EDGE ( 'NONE', *, *, #60064, .F. ) ;
#39590=CARTESIAN_POINT ( 'NONE',  ( -7.081429851441987999, -84.79152421822192309, -3.750000000000000000 ) ) ;
#39599=DIRECTION ( 'NONE',  ( -1.000000000000000000, -1.927470528863119542E-16, 0.000000000000000000 ) ) ;
#39603=CARTESIAN_POINT ( 'NONE',  ( -11.17376097835657411, -90.29818107662934779, 4.000000000000000888 ) ) ;
#39605=AXIS2_PLACEMENT_3D ( 'NONE', #12191, #19699, #41243 ) ;
#39617=CARTESIAN_POINT ( 'NONE',  ( -5.999999999999994671, 79.82179676972448590, 6.250000000000000000 ) ) ;
#39627=CARTESIAN_POINT ( 'NONE',  ( -3.750000000000000000, 10.25000000000000000, 4.000000000000000000 ) ) ;
#39648=ADVANCED_FACE ( 'NONE', ( #82237 ), #96777, .F. ) ;
#39656=CARTESIAN_POINT ( 'NONE',  ( -5.999999999999994671, 43.00000000000000000, -6.500000000000000888 ) ) ;
#39657=TOROIDAL_SURFACE ( 'NONE', #93955, 0.7500000000000008882, 0.2500000000000000000 ) ;
#39665=ORIENTED_EDGE ( 'NONE', *, *, #96255, .F. ) ;
#39672=CARTESIAN_POINT ( 'NONE',  ( -6.581680125707233486, -88.31141629936868753, -3.750000000000000000 ) ) ;
#39675=MECHANICAL_DESIGN_GEOMETRIC_PRESENTATION_REPRESENTATION('',(#76419),#46026);
#39676=DIRECTION ( 'NONE',  ( 0.000000000000000000, 0.000000000000000000, 1.000000000000000000 ) ) ;
#39679=CARTESIAN_POINT ( 'NONE',  ( -3.250000001579299802, 0.08818787376450962223, 2.500000000000000000 ) ) ;
#39681=SURFACE_STYLE_FILL_AREA ( #78151 ) ;
#39683=CARTESIAN_POINT ( 'NONE',  ( -8.099999999999999645, 80.99999999999994316, 0.000000000000000000 ) ) ;
#39685=FILL_AREA_STYLE_COLOUR ( '', #69146 ) ;
#39687=DIRECTION ( 'NONE',  ( -0.000000000000000000, -0.000000000000000000, 1.000000000000000000 ) ) ;
#39710=CARTESIAN_POINT ( 'NONE',  ( -4.000000000000000000, 10.00000000000000000, -3.750000000000000000 ) ) ;
#39732=CARTESIAN_POINT ( 'NONE',  ( 9.209312257346764952, -9.300771453421772250, -3.750000000000000000 ) ) ;
#39739=DIRECTION ( 'NONE',  ( 0.000000000000000000, 0.000000000000000000, 1.000000000000000000 ) ) ;
#39743=LINE ( 'NONE', #1271, #5929 ) ;
#39745=VERTEX_POINT ( 'NONE', #80767 ) ;
#39748=DIRECTION ( 'NONE',  ( 0.000000000000000000, 0.000000000000000000, 1.000000000000000000 ) ) ;
#39762=ORIENTED_EDGE ( 'NONE', *, *, #69352, .T. ) ;
#39787=VERTEX_POINT ( 'NONE', #35253 ) ;
#39788=DIRECTION ( 'NONE',  ( 1.000000000000000000, 0.000000000000000000, 0.000000000000000000 ) ) ;
#39801=DIRECTION ( 'NONE',  ( -0.9887436111420608853, -0.1496197561345335991, 0.000000000000000000 ) ) ;
#39805=TOROIDAL_SURFACE ( 'NONE', #87673, 0.5000000000000000000, 0.2500000000000000000 ) ;
#39811=CARTESIAN_POINT ( 'NONE',  ( -8.819573739049973327, 87.31373983715974418, 4.675023147224795395 ) ) ;
#39820=DIRECTION ( 'NONE',  ( -1.257402221000611116E-16, 1.000000000000000000, 0.000000000000000000 ) ) ;
#39823=DIRECTION ( 'NONE',  ( 0.000000000000000000, 0.000000000000000000, 1.000000000000000000 ) ) ;
#39830=CARTESIAN_POINT ( 'NONE',  ( -8.860528122731230027, 87.38741345285838236, -4.488970891313635470 ) ) ;
#39838=FILL_AREA_STYLE ('',( #9336 ) ) ;
#39847=CARTESIAN_POINT ( 'NONE',  ( 8.629999999999995453, 40.74999999999999289, -4.250000000000000000 ) ) ;
#39853=CIRCLE ( 'NONE', #81373, 0.5000000000000000000 ) ;
#39880=CARTESIAN_POINT ( 'NONE',  ( 12.50465990577749409, 56.99999999999999289, 3.000000000000000000 ) ) ;
#39884=EDGE_CURVE ( 'NONE', #25163, #64978, #68732, .T. ) ;
#39888=ORIENTED_EDGE ( 'NONE', *, *, #24777, .F. ) ;
#39900=ORIENTED_EDGE ( 'NONE', *, *, #44473, .T. ) ;
#39911=CARTESIAN_POINT ( 'NONE',  ( -10.91596227336299663, -97.59461837500816728, 3.749999999999999556 ) ) ;
#39912=FACE_OUTER_BOUND ( 'NONE', #17732, .T. ) ;
#39916=ADVANCED_FACE ( 'NONE', ( #75729 ), #46702, .F. ) ;
#39939=CARTESIAN_POINT ( 'NONE',  ( 8.956109388601815269, -3.116898856182344080, 3.750000000000001332 ) ) ;
#39944=CARTESIAN_POINT ( 'NONE',  ( -6.000000000000014211, 80.07179676972448590, -4.250000000000000000 ) ) ;
#39954=DIRECTION ( 'NONE',  ( -0.000000000000000000, -0.000000000000000000, 1.000000000000000000 ) ) ;
#39957=CARTESIAN_POINT ( 'NONE',  ( 14.99999999999998046, 70.25000000000000000, -6.500000000000000888 ) ) ;
#39966=TOROIDAL_SURFACE ( 'NONE', #38401, 7.250000000000002665, 0.2500000000000000000 ) ;
#39973=EDGE_CURVE ( 'NONE', #69208, #76544, #84716, .T. ) ;
#39978=DIRECTION ( 'NONE',  ( 0.000000000000000000, 1.000000000000000000, 0.000000000000000000 ) ) ;
#39983=SURFACE_SIDE_STYLE ('',( #17974 ) ) ;
#39998=EDGE_CURVE ( 'NONE', #52968, #49408, #61244, .T. ) ;
#40011=VERTEX_POINT ( 'NONE', #67248 ) ;
#40021=ORIENTED_EDGE ( 'NONE', *, *, #38922, .F. ) ;
#40037=CARTESIAN_POINT ( 'NONE',  ( -8.124115902427741176, 75.04369783535875627, 3.000000000000000000 ) ) ;
#40040=ORIENTED_EDGE ( 'NONE', *, *, #82692, .F. ) ;
#40043=VERTEX_POINT ( 'NONE', #15742 ) ;
#40044=CARTESIAN_POINT ( 'NONE',  ( -7.750000000000000000, 79.82179676972448590, 6.250000000000000000 ) ) ;
#40051=DIRECTION ( 'NONE',  ( -1.000000000000000000, 0.000000000000000000, 0.000000000000000000 ) ) ;
#40064=ORIENTED_EDGE ( 'NONE', *, *, #8840, .T. ) ;
#40073=DIRECTION ( 'NONE',  ( -0.000000000000000000, -0.000000000000000000, 1.000000000000000000 ) ) ;
#40080=DIRECTION ( 'NONE',  ( -0.9975640502598243087, 0.06975647374412545509, 0.000000000000000000 ) ) ;
#40082=ADVANCED_FACE ( 'NONE', ( #61219, #29237, #61696, #91722 ), #23243, .T. ) ;
#40094=CIRCLE ( 'NONE', #12886, 1.249999999999987121 ) ;
#40096=ORIENTED_EDGE ( 'NONE', *, *, #39564, .F. ) ;
#40105=SURFACE_STYLE_FILL_AREA ( #47605 ) ;
#40108=CARTESIAN_POINT ( 'NONE',  ( -10.20000000000000107, 43.92361346574197256, -2.900000000000000799 ) ) ;
#40114=EDGE_CURVE ( 'NONE', #60118, #74806, #85161, .T. ) ;
#40117=CARTESIAN_POINT ( 'NONE',  ( -18.89999999999999503, 98.99999999999998579, 8.000000000000000000 ) ) ;
#40124=EDGE_CURVE ( 'NONE', #14317, #18642, #48389, .T. ) ;
#40138=DIRECTION ( 'NONE',  ( 6.938893903907222067E-15, -1.000000000000000000, 0.000000000000000000 ) ) ;
#40141=ORIENTED_EDGE ( 'NONE', *, *, #16476, .F. ) ;
#40153=STYLED_ITEM ( 'NONE', ( #81626 ), #63320 ) ;
#40155=CARTESIAN_POINT ( 'NONE',  ( -3.521809514228321003, -0.8352226969044395100, 2.499999999999597655 ) ) ;
#40157=DIRECTION ( 'NONE',  ( 0.9975640502598257520, -0.06975647374410356982, 0.000000000000000000 ) ) ;
#40164=DIRECTION ( 'NONE',  ( 1.000000000000000000, 1.189524669241238632E-14, 0.000000000000000000 ) ) ;
#40169=VERTEX_POINT ( 'NONE', #87154 ) ;
#40171=VECTOR ( 'NONE', #66151, 1000.000000000000000 ) ;
#40176=DIRECTION ( 'NONE',  ( 0.000000000000000000, 0.000000000000000000, -1.000000000000000000 ) ) ;
#40193=DIRECTION ( 'NONE',  ( 0.000000000000000000, -1.000000000000000000, 0.000000000000000000 ) ) ;
#40201=AXIS2_PLACEMENT_3D ( 'NONE', #36277, #3824, #12780 ) ;
#40214=ORIENTED_EDGE ( 'NONE', *, *, #68885, .F. ) ;
#40244=CARTESIAN_POINT ( 'NONE',  ( 18.00000000000000000, 77.07179676972447169, 4.250000000000000000 ) ) ;
#40248=CARTESIAN_POINT ( 'NONE',  ( -7.124934413272103306, -78.83349193436582425, 4.000000000000000888 ) ) ;
#40273=AXIS2_PLACEMENT_3D ( 'NONE', #62495, #24533, #75541 ) ;
#40282=EDGE_CURVE ( 'NONE', #43677, #63872, #24513, .T. ) ;
#40288=DIRECTION ( 'NONE',  ( 1.000000000000000000, 0.000000000000000000, 0.000000000000000000 ) ) ;
#40289=CARTESIAN_POINT ( 'NONE',  ( 9.879999999999988347, 26.99999999999999645, 3.000000000000000000 ) ) ;
#40303=VERTEX_POINT ( 'NONE', #81625 ) ;
#40309=( NAMED_UNIT ( * ) SI_UNIT ( $, .STERADIAN. ) SOLID_ANGLE_UNIT ( ) );
#40315=CIRCLE ( 'NONE', #67437, 0.2500000000000002220 ) ;
#40325=DIRECTION ( 'NONE',  ( -0.02177529129954166101, -0.9997628902338895340, -5.564908543122672015E-14 ) ) ;
#40329=FACE_OUTER_BOUND ( 'NONE', #77218, .T. ) ;
#40332=EDGE_CURVE ( 'NONE', #79587, #9323, #35132, .T. ) ;
#40344=DIRECTION ( 'NONE',  ( 0.000000000000000000, -1.000000000000000000, 0.000000000000000000 ) ) ;
#40350=PRESENTATION_STYLE_ASSIGNMENT (( #54346 ) ) ;
#40368=ADVANCED_FACE ( 'NONE', ( #80148 ), #59591, .F. ) ;
#40378=EDGE_LOOP ( 'NONE', ( #92142, #67753, #68262, #47193 ) ) ;
#40388=AXIS2_PLACEMENT_3D ( 'NONE', #74971, #12498, #80995 ) ;
#40400=DIRECTION ( 'NONE',  ( 0.000000000000000000, 1.000000000000000000, -0.000000000000000000 ) ) ;
#40405=VERTEX_POINT ( 'NONE', #19652 ) ;
#40409=MECHANICAL_DESIGN_GEOMETRIC_PRESENTATION_REPRESENTATION('',(#61161),#30822);
#40414=CARTESIAN_POINT ( 'NONE',  ( -11.60534915929947708, -82.02544043777214711, 3.750000000000000444 ) ) ;
#40425=FILL_AREA_STYLE ('',( #26379 ) ) ;
#40430=DIRECTION ( 'NONE',  ( 0.000000000000000000, 0.000000000000000000, 1.000000000000000000 ) ) ;
#40431=DIRECTION ( 'NONE',  ( 2.569960705150826877E-16, -1.000000000000000000, -0.000000000000000000 ) ) ;
#40452=CARTESIAN_POINT ( 'NONE',  ( -4.010449548136814535, -13.83555390988818523, -2.500000000000000888 ) ) ;
#40457=( NAMED_UNIT ( * ) PLANE_ANGLE_UNIT ( ) SI_UNIT ( $, .RADIAN. ) );
#40459=CARTESIAN_POINT ( 'NONE',  ( 4.630000001262032150, 0.09071174558778491437, -4.000000000000000000 ) ) ;
#40460=SURFACE_STYLE_USAGE ( .BOTH. , #47934 ) ;
#40463=LINE ( 'NONE', #1982, #38393 ) ;
#40474=CARTESIAN_POINT ( 'NONE',  ( 18.00000000000001776, 4.625929269271493211E-15, 3.750000000000000000 ) ) ;
#40475=UNCERTAINTY_MEASURE_WITH_UNIT (LENGTH_MEASURE( 1.000000000000000082E-05 ), #19141, 'distance_accuracy_value', 'NONE');
#40482=LINE ( 'NONE', #8498, #308 ) ;
#40484=DIRECTION ( 'NONE',  ( 1.049065152435176504E-16, -1.000000000000000000, 0.000000000000000000 ) ) ;
#40500=CIRCLE ( 'NONE', #19711, 0.2500000000000002220 ) ;
#40509=CARTESIAN_POINT ( 'NONE',  ( -8.469613711665671119, -9.365740742666716301, -3.750000000000000444 ) ) ;
#40536=DIRECTION ( 'NONE',  ( 0.000000000000000000, 0.000000000000000000, 1.000000000000000000 ) ) ;
#40558=CARTESIAN_POINT ( 'NONE',  ( 8.979999999999991545, 27.03929484861771826, -3.000000000000000000 ) ) ;
#40569=CARTESIAN_POINT ( 'NONE',  ( -7.804338076140435732, 84.96756567522902515, 4.038273117401847578 ) ) ;
#40581=CARTESIAN_POINT ( 'NONE',  ( -9.543970587329795308, -28.01866822101010612, 3.999999999999999112 ) ) ;
#40591=DIRECTION ( 'NONE',  ( 0.000000000000000000, 0.000000000000000000, 1.000000000000000000 ) ) ;
#40606=DIRECTION ( 'NONE',  ( -0.02177529129959714441, -0.9997628902338883128, 0.000000000000000000 ) ) ;
#40621=EDGE_CURVE ( 'NONE', #19964, #46091, #13281, .T. ) ;
#40626=ORIENTED_EDGE ( 'NONE', *, *, #55843, .T. ) ;
#40634=CIRCLE ( 'NONE', #69603, 3.000000000000002665 ) ;
#40649=STYLED_ITEM ( 'NONE', ( #56878 ), #98724 ) ;
#40651=CARTESIAN_POINT ( 'NONE',  ( -5.079065453169564037, -28.67168118942975497, 2.500000000000000888 ) ) ;
#40652=ORIENTED_EDGE ( 'NONE', *, *, #48337, .F. ) ;
#40653=EDGE_CURVE ( 'NONE', #37189, #51203, #69181, .T. ) ;
#40654=SURFACE_STYLE_USAGE ( .BOTH. , #9662 ) ;
#40656=ADVANCED_FACE ( 'NONE', ( #91481 ), #45480, .T. ) ;
#40657=CIRCLE ( 'NONE', #24751, 0.2500000000000002220 ) ;
#40659=CARTESIAN_POINT ( 'NONE',  ( -3.635384400432159158, -3.854802480546752896, 2.750000000000000000 ) ) ;
#40665=VERTEX_POINT ( 'NONE', #76476 ) ;
#40673=CARTESIAN_POINT ( 'NONE',  ( 4.573260519721095818, -6.401749983321133541, -2.750000000000000000 ) ) ;
#40690=AXIS2_PLACEMENT_3D ( 'NONE', #2658, #33110, #24649 ) ;
#40706=VERTEX_POINT ( 'NONE', #7991 ) ;
#40719=ORIENTED_EDGE ( 'NONE', *, *, #18796, .T. ) ;
#40721=CARTESIAN_POINT ( 'NONE',  ( 2.550000000000003819, 99.99999999999998579, -8.525133428036873795 ) ) ;
#40727=SURFACE_STYLE_FILL_AREA ( #26692 ) ;
#40731=AXIS2_PLACEMENT_3D ( 'NONE', #64849, #42376, #4387 ) ;
#40737=CARTESIAN_POINT ( 'NONE',  ( -6.031993939728320875, -39.82530731229964260, 3.999999999998387068 ) ) ;
#40740=ORIENTED_EDGE ( 'NONE', *, *, #61171, .T. ) ;
#40746=DIRECTION ( 'NONE',  ( -1.000000000000000000, 0.000000000000000000, 0.000000000000000000 ) ) ;
#40750=( GEOMETRIC_REPRESENTATION_CONTEXT ( 3 ) GLOBAL_UNCERTAINTY_ASSIGNED_CONTEXT ( ( #3201 ) ) GLOBAL_UNIT_ASSIGNED_CONTEXT ( ( #69237, #61228, #53236 ) ) REPRESENTATION_CONTEXT ( 'NONE', 'WORKASPACE' ) );
#40765=ADVANCED_FACE ( 'NONE', ( #94915 ), #3443, .F. ) ;
#40768=SURFACE_SIDE_STYLE ('',( #49719 ) ) ;
#40771=ADVANCED_FACE ( 'NONE', ( #86448 ), #75521, .T. ) ;
#40772=FACE_OUTER_BOUND ( 'NONE', #63293, .T. ) ;
#40783=( NAMED_UNIT ( * ) SI_UNIT ( $, .STERADIAN. ) SOLID_ANGLE_UNIT ( ) );
#40784=CYLINDRICAL_SURFACE ( 'NONE', #75263, 7.000000000000002665 ) ;
#40793=CARTESIAN_POINT ( 'NONE',  ( -9.483770294663347755, 88.32858231846624619, 5.216041430090285758 ) ) ;
#40801=CARTESIAN_POINT ( 'NONE',  ( 14.99999999999997868, 79.82179676972448590, -6.250000000000000000 ) ) ;
#40812=EDGE_CURVE ( 'NONE', #67453, #15068, #26066, .T. ) ;
#40827=CARTESIAN_POINT ( 'NONE',  ( 14.99999999999997868, 80.07179676972448590, -4.250000000000000000 ) ) ;
#40832=CARTESIAN_POINT ( 'NONE',  ( 10.47193227288532569, -40.28585825680447385, -3.999999999999999112 ) ) ;
#40848=DIRECTION ( 'NONE',  ( -0.9975640502598257520, 0.06975647374410356982, 0.000000000000000000 ) ) ;
#40857=ORIENTED_EDGE ( 'NONE', *, *, #24949, .F. ) ;
#40880=ORIENTED_EDGE ( 'NONE', *, *, #60401, .F. ) ;
#40897=EDGE_LOOP ( 'NONE', ( #64418, #76512, #21833, #9770, #54586, #90671, #22560, #6840, #37117, #73950 ) ) ;
#40901=CARTESIAN_POINT ( 'NONE',  ( -10.07519558535470239, -32.17712024071101951, 3.750000000000001332 ) ) ;
#40906=CIRCLE ( 'NONE', #74433, 0.09999999999999982514 ) ;
#40907=CARTESIAN_POINT ( 'NONE',  ( -3.499999999999998668, 1.019547802438465434, 2.500000000000000000 ) ) ;
#40912=ORIENTED_EDGE ( 'NONE', *, *, #21359, .T. ) ;
#40916=EDGE_CURVE ( 'NONE', #3878, #43714, #18072, .T. ) ;
#40921=DIRECTION ( 'NONE',  ( 0.000000000000000000, 1.000000000000000000, 0.000000000000000000 ) ) ;
#40932=ORIENTED_EDGE ( 'NONE', *, *, #10178, .F. ) ;
#40943=CIRCLE ( 'NONE', #96841, 2.250000000000000444 ) ;
#40944=CARTESIAN_POINT ( 'NONE',  ( -3.250000000000000444, 1.019547802438465656, -2.500000000000000000 ) ) ;
#40953=MANIFOLD_SOLID_BREP ( 'Fillet11', #60156 ) ;
#40955=CARTESIAN_POINT ( 'NONE',  ( -7.750000000000000000, 43.00000000000000000, 6.250000000000000000 ) ) ;
#40984=AXIS2_PLACEMENT_3D ( 'NONE', #80968, #73452, #4002 ) ;
#40990=AXIS2_PLACEMENT_3D ( 'NONE', #73576, #20094, #34589 ) ;
#41000=CARTESIAN_POINT ( 'NONE',  ( -11.30269888132237810, -57.08933895092661004, -3.749999999999999556 ) ) ;
#41013=LINE ( 'NONE', #26478, #93754 ) ;
#41015=CIRCLE ( 'NONE', #90527, 0.2500000000000002220 ) ;
#41021=ORIENTED_EDGE ( 'NONE', *, *, #87262, .F. ) ;
#41031=ORIENTED_EDGE ( 'NONE', *, *, #21354, .F. ) ;
#41032=MECHANICAL_DESIGN_GEOMETRIC_PRESENTATION_REPRESENTATION('',(#95329),#92123);
#41034=CIRCLE ( 'NONE', #66574, 0.2499999999999997780 ) ;
#41043=( NAMED_UNIT ( * ) PLANE_ANGLE_UNIT ( ) SI_UNIT ( $, .RADIAN. ) );
#41046=( NAMED_UNIT ( * ) PLANE_ANGLE_UNIT ( ) SI_UNIT ( $, .RADIAN. ) );
#41052=CARTESIAN_POINT ( 'NONE',  ( 0.000000000000000000, -97.00000000000000000, -3.750000000000000000 ) ) ;
#41056=COLOUR_RGB ( '', 0.40784314, 0.44705882, 0.49803922) ;
#41059=ORIENTED_EDGE ( 'NONE', *, *, #61660, .T. ) ;
#41073=FILL_AREA_STYLE_COLOUR ( '', #10124 ) ;
#41076=CARTESIAN_POINT ( 'NONE',  ( -7.750000000000000000, 1.019547802438458550, 4.000000000000000000 ) ) ;
#41080=DIRECTION ( 'NONE',  ( -0.000000000000000000, -0.000000000000000000, -1.000000000000000000 ) ) ;
#41081=( LENGTH_UNIT ( ) NAMED_UNIT ( * ) SI_UNIT ( .MILLI., .METRE. ) );
#41083=MECHANICAL_DESIGN_GEOMETRIC_PRESENTATION_REPRESENTATION('',(#79397),#92175);
#41087=FACE_OUTER_BOUND ( 'NONE', #69987, .T. ) ;
#41088=CYLINDRICAL_SURFACE ( 'NONE', #80051, 0.2500000000000002220 ) ;
#41104=AXIS2_PLACEMENT_3D ( 'NONE', #24952, #33397, #3916 ) ;
#41105=ADVANCED_FACE ( 'NONE', ( #84665 ), #8662, .T. ) ;
#41106=CIRCLE ( 'NONE', #9182, 0.2500000000000002220 ) ;
#41109=AXIS2_PLACEMENT_3D ( 'NONE', #54001, #8508, #84993 ) ;
#41116=CARTESIAN_POINT ( 'NONE',  ( 12.24319267753454099, 54.01141590572476048, 0.000000000000000000 ) ) ;
#41121=SURFACE_SIDE_STYLE ('',( #33580 ) ) ;
#41134=LINE ( 'NONE', #57582, #37570 ) ;
#41137=EDGE_CURVE ( 'NONE', #35809, #93854, #66521, .T. ) ;
#41140=ORIENTED_EDGE ( 'NONE', *, *, #55529, .T. ) ;
#41144=ORIENTED_EDGE ( 'NONE', *, *, #18998, .F. ) ;
#41151=AXIS2_PLACEMENT_3D ( 'NONE', #27064, #56109, #35051 ) ;
#41154=CARTESIAN_POINT ( 'NONE',  ( -5.068142462348440347, -24.94450071860939033, 2.749999999999193978 ) ) ;
#41156=CARTESIAN_POINT ( 'NONE',  ( 11.18123354730910002, -92.99280210684537451, 4.000000000000002665 ) ) ;
#41160=CARTESIAN_POINT ( 'NONE',  ( -7.127794346849581686, -80.93619716733995517, 3.750000000000000444 ) ) ;
#41165=DIRECTION ( 'NONE',  ( 1.483861936729427615E-16, -1.000000000000000000, 0.000000000000000000 ) ) ;
#41169=( LENGTH_UNIT ( ) NAMED_UNIT ( * ) SI_UNIT ( .MILLI., .METRE. ) );
#41171=( LENGTH_UNIT ( ) NAMED_UNIT ( * ) SI_UNIT ( .MILLI., .METRE. ) );
#41174=ADVANCED_FACE ( 'NONE', ( #34100 ), #27593, .T. ) ;
#41184=FACE_OUTER_BOUND ( 'NONE', #8677, .T. ) ;
#41185=CARTESIAN_POINT ( 'NONE',  ( 0.000000000000000000, 84.07179676972448590, -4.000000000000000000 ) ) ;
#41186=ADVANCED_FACE ( 'NONE', ( #66080 ), #96108, .T. ) ;
#41193=CARTESIAN_POINT ( 'NONE',  ( -11.30180206635974116, -57.06075279890724516, -4.000000000003605116 ) ) ;
#41196=DIRECTION ( 'NONE',  ( 1.000000000000000000, 1.927470528863119542E-16, -0.000000000000000000 ) ) ;
#41203=ORIENTED_EDGE ( 'NONE', *, *, #7259, .T. ) ;
#41210=UNCERTAINTY_MEASURE_WITH_UNIT (LENGTH_MEASURE( 1.000000000000000082E-05 ), #45625, 'distance_accuracy_value', 'NONE');
#41211=( BOUNDED_SURFACE ( )  B_SPLINE_SURFACE ( 3, 2, ( 
 ( #78927, #49897, #2471 ),
 ( #72393, #11411, #95912 ),
 ( #93934, #33407, #57883 ),
 ( #33893, #3434, #3922 ),
 ( #25458, #94907, #88397 ),
 ( #10924, #64398, #26406 ),
 ( #80406, #56906, #95406 ),
 ( #87409, #42410, #40452 ),
 ( #18926, #63905, #49402 ),
 ( #71442, #86440, #34392 ),
 ( #26903, #17940, #57399 ),
 ( #72889, #48424, #47926 ),
 ( #78432, #9949, #2956 ),
 ( #94416, #86920, #18431 ),
 ( #48914, #60354, #28385 ),
 ( #90347, #12880, #82868 ),
 ( #97899, #21885, #80897 ),
 ( #58877, #20399, #73380 ),
 ( #89379, #19894, #50387 ),
 ( #13381, #12393, #43378 ),
 ( #36880, #97393, #52363 ),
 ( #42898, #20892, #35387 ) ),
 .UNSPECIFIED., .F., .F., .F. ) 
 B_SPLINE_SURFACE_WITH_KNOTS ( ( 4, 2, 2, 2, 2, 2, 2, 2, 2, 2, 4 ),
 ( 3, 3 ),
 ( -1.040834085586084257E-17, 0.002788823349942579858, 0.005577646699885170124, 0.01115529339977035066, 0.02231058679954071172, 0.03346588019931107105, 0.04462117359908143038, 0.06693176039862215598, 0.07808705379839250837, 0.08366470049827769151, 0.08924234719816287464 ),
 ( 0.000000000000000000, 1.000000000000000000 ),
 .UNSPECIFIED. ) 
 GEOMETRIC_REPRESENTATION_ITEM ( )  RATIONAL_B_SPLINE_SURFACE ( (
 ( 1.000000000000000000, 0.7071067811865475727, 1.000000000000000000),
 ( 1.000000000000000000, 0.7071067811865475727, 1.000000000000000000),
 ( 1.000000000000000000, 0.7071067811865469066, 1.000000000000000000),
 ( 1.000000000000000000, 0.7071067811865469066, 1.000000000000000000),
 ( 1.000000000000000000, 0.7071067811865482389, 1.000000000000000000),
 ( 1.000000000000000000, 0.7071067811865482389, 1.000000000000000000),
 ( 1.000000000000000000, 0.7071067811865487940, 1.000000000000000000),
 ( 1.000000000000000000, 0.7071067811865487940, 1.000000000000000000),
 ( 1.000000000000000000, 0.7071067811865482389, 1.000000000000000000),
 ( 1.000000000000000000, 0.7071067811865482389, 1.000000000000000000),
 ( 1.000000000000000000, 0.7071067811865493491, 1.000000000000000000),
 ( 1.000000000000000000, 0.7071067811865493491, 1.000000000000000000),
 ( 1.000000000000000000, 0.7071067811865473507, 1.000000000000000000),
 ( 1.000000000000000000, 0.7071067811865473507, 1.000000000000000000),
 ( 1.000000000000000000, 0.7071067811865482389, 1.000000000000000000),
 ( 1.000000000000000000, 0.7071067811865482389, 1.000000000000000000),
 ( 1.000000000000000000, 0.7071067811865482389, 1.000000000000000000),
 ( 1.000000000000000000, 0.7071067811865482389, 1.000000000000000000),
 ( 1.000000000000000000, 0.7071067811865482389, 1.000000000000000000),
 ( 1.000000000000000000, 0.7071067811865482389, 1.000000000000000000),
 ( 1.000000000000000000, 0.7071067811865482389, 1.000000000000000000),
 ( 1.000000000000000000, 0.7071067811865482389, 1.000000000000000000) ) ) 
 REPRESENTATION_ITEM ( '' )  SURFACE ( )  );
#41216=CARTESIAN_POINT ( 'NONE',  ( 8.955816604300867567, -3.107613341155669229, -4.000000000000000000 ) ) ;
#41227=DIRECTION ( 'NONE',  ( -0.000000000000000000, 0.000000000000000000, 1.000000000000000000 ) ) ;
#41228=ORIENTED_EDGE ( 'NONE', *, *, #39383, .F. ) ;
#41232=CARTESIAN_POINT ( 'NONE',  ( -11.81797300553251162, -43.76346696326814367, 3.750000000000000000 ) ) ;
#41239=EDGE_CURVE ( 'NONE', #22085, #74593, #84089, .T. ) ;
#41243=DIRECTION ( 'NONE',  ( 1.000000000000000000, -5.551115123125777653E-14, 0.000000000000000000 ) ) ;
#41248=CARTESIAN_POINT ( 'NONE',  ( -7.124934413296625912, -78.83349193436581004, 3.750000000000000888 ) ) ;
#41249=ORIENTED_EDGE ( 'NONE', *, *, #24332, .F. ) ;
#41259=CIRCLE ( 'NONE', #4554, 4.190000000000001279 ) ;
#41262=EDGE_CURVE ( 'NONE', #72885, #27580, #39120, .T. ) ;
#41296=EDGE_CURVE ( 'NONE', #61288, #52968, #93447, .T. ) ;
#41298=AXIS2_PLACEMENT_3D ( 'NONE', #30392, #15905, #76883 ) ;
#41301=CARTESIAN_POINT ( 'NONE',  ( -8.443706647342963834, 87.03308080853030049, 4.556631258847859911 ) ) ;
#41318=( GEOMETRIC_REPRESENTATION_CONTEXT ( 3 ) GLOBAL_UNCERTAINTY_ASSIGNED_CONTEXT ( ( #95302 ) ) GLOBAL_UNIT_ASSIGNED_CONTEXT ( ( #16146, #93116, #9631 ) ) REPRESENTATION_CONTEXT ( 'NONE', 'WORKASPACE' ) );
#41326=DIRECTION ( 'NONE',  ( 0.6038238647437471629, -0.7971177707001175783, -1.734723475976782837E-15 ) ) ;
#41327=CARTESIAN_POINT ( 'NONE',  ( -9.093709202272499681, 88.10000367580643399, -5.077063215882387404 ) ) ;
#41331=ADVANCED_FACE ( 'NONE', ( #67079 ), #45058, .T. ) ;
#41335=ORIENTED_EDGE ( 'NONE', *, *, #12845, .T. ) ;
#41336=SURFACE_STYLE_USAGE ( .BOTH. , #4794 ) ;
#41394=DIRECTION ( 'NONE',  ( -1.000000000000000000, 0.000000000000000000, 0.000000000000000000 ) ) ;
#41398=( GEOMETRIC_REPRESENTATION_CONTEXT ( 3 ) GLOBAL_UNCERTAINTY_ASSIGNED_CONTEXT ( ( #3331 ) ) GLOBAL_UNIT_ASSIGNED_CONTEXT ( ( #72088, #50575, #4601 ) ) REPRESENTATION_CONTEXT ( 'NONE', 'WORKASPACE' ) );
#41412=( NAMED_UNIT ( * ) SI_UNIT ( $, .STERADIAN. ) SOLID_ANGLE_UNIT ( ) );
#41414=CARTESIAN_POINT ( 'NONE',  ( 0.000000000000000000, -97.00000000000000000, 2.750000000000000000 ) ) ;
#41424=DIRECTION ( 'NONE',  ( 0.7808688094430307203, -0.6246950475544238435, 0.000000000000000000 ) ) ;
#41434=CIRCLE ( 'NONE', #47756, 0.2500000000000002220 ) ;
#41440=SPHERICAL_SURFACE ( 'NONE', #83235, 0.2500000000000000000 ) ;
#41442=FACE_OUTER_BOUND ( 'NONE', #79233, .T. ) ;
#41446=EDGE_LOOP ( 'NONE', ( #8949, #98324, #53543, #91392 ) ) ;
#41449=FILL_AREA_STYLE ('',( #70952 ) ) ;
#41456=CARTESIAN_POINT ( 'NONE',  ( -6.857531195348600228, -50.94829529698463233, 4.000000000000000888 ) ) ;
#41463=CARTESIAN_POINT ( 'NONE',  ( 15.00000000000000178, 73.00000000000000000, -6.500000000000000888 ) ) ;
#41466=VERTEX_POINT ( 'NONE', #73974 ) ;
#41476=ORIENTED_EDGE ( 'NONE', *, *, #57475, .F. ) ;
#41484=ORIENTED_EDGE ( 'NONE', *, *, #3243, .F. ) ;
#41505=VERTEX_POINT ( 'NONE', #26507 ) ;
#41534=ORIENTED_EDGE ( 'NONE', *, *, #57735, .T. ) ;
#41535=CARTESIAN_POINT ( 'NONE',  ( -5.999999999999994671, 43.00000000000000000, -4.000000000000000000 ) ) ;
#41543=DIRECTION ( 'NONE',  ( 1.000000000000000000, 0.000000000000000000, 0.000000000000000000 ) ) ;
#41545=CARTESIAN_POINT ( 'NONE',  ( 8.879999999999991900, 69.99999999999998579, 6.250000000000000000 ) ) ;
#41550=AXIS2_PLACEMENT_3D ( 'NONE', #8894, #69905, #63847 ) ;
#41555=CARTESIAN_POINT ( 'NONE',  ( 12.14357320772536752, 54.02013147999952736, 3.000000000000000000 ) ) ;
#41567=PLANE ( 'NONE',  #57676 ) ;
#41576=CARTESIAN_POINT ( 'NONE',  ( -11.38910604377741898, -77.84323126545000093, -4.000000000000000888 ) ) ;
#41578=LINE ( 'NONE', #48058, #32066 ) ;
#41590=FILL_AREA_STYLE ('',( #11069 ) ) ;
#41603=( NAMED_UNIT ( * ) SI_UNIT ( $, .STERADIAN. ) SOLID_ANGLE_UNIT ( ) );
#41605=ORIENTED_EDGE ( 'NONE', *, *, #24251, .F. ) ;
#41609=CARTESIAN_POINT ( 'NONE',  ( -8.900000000000002132, 83.89999999999994884, 0.000000000000000000 ) ) ;
#41610=DIRECTION ( 'NONE',  ( 0.08715574274766037244, 0.9961946980917453232, 1.511911130105620530E-15 ) ) ;
#41624=ORIENTED_EDGE ( 'NONE', *, *, #66614, .T. ) ;
#41632=ORIENTED_EDGE ( 'NONE', *, *, #56758, .F. ) ;
#41643=FACE_OUTER_BOUND ( 'NONE', #54521, .T. ) ;
#41647=CARTESIAN_POINT ( 'NONE',  ( 10.83696084481538691, -98.17058944465519232, 3.750000000000000000 ) ) ;
#41651=CARTESIAN_POINT ( 'NONE',  ( -4.247994584727555534, -13.56436116443237516, 3.750000000000000444 ) ) ;
#41652=DIRECTION ( 'NONE',  ( 0.000000000000000000, -0.000000000000000000, -1.000000000000000000 ) ) ;
#41660=CARTESIAN_POINT ( 'NONE',  ( 10.83696084481538691, -98.17058944465519232, 3.750000000000000000 ) ) ;
#41674=CARTESIAN_POINT ( 'NONE',  ( -19.89999999999999858, 98.99999999999998579, 7.750000000000000000 ) ) ;
#41676=DIRECTION ( 'NONE',  ( -0.000000000000000000, -0.000000000000000000, 1.000000000000000000 ) ) ;
#41681=CARTESIAN_POINT ( 'NONE',  ( -11.02864780715742299, -96.54579228616290720, -3.750000000000000000 ) ) ;
#41683=DIRECTION ( 'NONE',  ( -0.000000000000000000, -0.000000000000000000, 1.000000000000000000 ) ) ;
#41696=EDGE_CURVE ( 'NONE', #35160, #71617, #79520, .T. ) ;
#41702=CARTESIAN_POINT ( 'NONE',  ( 6.829574850499570360, -88.00372650123708240, 3.750000000000001332 ) ) ;
#41716=CIRCLE ( 'NONE', #44902, 0.2500000000000002220 ) ;
#41728=LINE ( 'NONE', #78229, #340 ) ;
#41748=EDGE_LOOP ( 'NONE', ( #77257, #61784, #66227, #84219 ) ) ;
#41750=ORIENTED_EDGE ( 'NONE', *, *, #71947, .T. ) ;
#41775=AXIS2_PLACEMENT_3D ( 'NONE', #64266, #92811, #56780 ) ;
#41782=CARTESIAN_POINT ( 'NONE',  ( -8.099999999999999645, 75.73428692542562146, -3.000000000000000000 ) ) ;
#41785=( BOUNDED_SURFACE ( )  B_SPLINE_SURFACE ( 3, 2, ( 
 ( #53677, #84194, #8191 ),
 ( #15703, #46188, #38688 ),
 ( #84674, #16182, #8671 ),
 ( #39183, #69672, #1201 ),
 ( #31659, #62146, #92654 ),
 ( #24180, #54649, #16676 ),
 ( #64110, #80109, #21470 ),
 ( #5979, #51969, #6457 ),
 ( #19119, #36471, #56630 ),
 ( #81957, #94626, #59453 ),
 ( #11616, #94130, #86644 ),
 ( #34105, #63624, #25657 ),
 ( #57110, #56150, #87118 ),
 ( #13471, #42132, #97484 ),
 ( #79628, #65091, #18636 ),
 ( #72598, #82454, #33614 ),
 ( #89954, #26137, #95106 ),
 ( #3149, #49600, #48626 ),
 ( #57602, #27102, #13978 ),
 ( #19611, #41156, #79130 ),
 ( #4134, #87608, #88102 ),
 ( #95615, #51468, #43952 ),
 ( #34597, #49126, #74451 ),
 ( #66965, #28951, #10642 ),
 ( #44453, #18152, #74954 ),
 ( #11129, #71641, #41647 ) ),
 .UNSPECIFIED., .F., .F., .F. ) 
 B_SPLINE_SURFACE_WITH_KNOTS ( ( 4, 2, 2, 2, 2, 2, 2, 2, 2, 2, 2, 2, 4 ),
 ( 3, 3 ),
 ( 0.000000000000000000, 0.003100998889883697755, 0.006201997779767395511, 0.01240399555953479102, 0.02480799111906958204, 0.04961598223813916408, 0.06201997779767395164, 0.07442397335720873919, 0.08682796891674353368, 0.09302996669651092398, 0.09613096558639462608, 0.09768146503133648406, 0.09923196447627832817 ),
 ( 0.000000000000000000, 1.000000000000000000 ),
 .UNSPECIFIED. ) 
 GEOMETRIC_REPRESENTATION_ITEM ( )  RATIONAL_B_SPLINE_SURFACE ( (
 ( 1.000000000000000000, 0.7071067811865475727, 1.000000000000000000),
 ( 1.000000000000000000, 0.7071067811865475727, 1.000000000000000000),
 ( 1.000000000000000000, 0.7071067811865475727, 1.000000000000000000),
 ( 1.000000000000000000, 0.7071067811865475727, 1.000000000000000000),
 ( 1.000000000000000000, 0.7071067811865475727, 1.000000000000000000),
 ( 1.000000000000000000, 0.7071067811865475727, 1.000000000000000000),
 ( 1.000000000000000000, 0.7071067811865475727, 1.000000000000000000),
 ( 1.000000000000000000, 0.7071067811865475727, 1.000000000000000000),
 ( 1.000000000000000000, 0.7071067811865475727, 1.000000000000000000),
 ( 1.000000000000000000, 0.7071067811865475727, 1.000000000000000000),
 ( 1.000000000000000000, 0.7071067811865472397, 1.000000000000000000),
 ( 1.000000000000000000, 0.7071067811865472397, 1.000000000000000000),
 ( 1.000000000000000000, 0.7071067811865475727, 1.000000000000000000),
 ( 1.000000000000000000, 0.7071067811865475727, 1.000000000000000000),
 ( 1.000000000000000000, 0.7071067811865475727, 1.000000000000000000),
 ( 1.000000000000000000, 0.7071067811865475727, 1.000000000000000000),
 ( 1.000000000000000000, 0.7071067811865477948, 1.000000000000000000),
 ( 1.000000000000000000, 0.7071067811865477948, 1.000000000000000000),
 ( 1.000000000000000000, 0.7071067811865443531, 1.000000000000000000),
 ( 1.000000000000000000, 0.7071067811865443531, 1.000000000000000000),
 ( 1.000000000000000000, 0.7071067811865475727, 1.000000000000000000),
 ( 1.000000000000000000, 0.7071067811865475727, 1.000000000000000000),
 ( 1.000000000000000000, 0.7071067811865475727, 1.000000000000000000),
 ( 1.000000000000000000, 0.7071067811865475727, 1.000000000000000000),
 ( 1.000000000000000000, 0.7071067811865475727, 1.000000000000000000),
 ( 1.000000000000000000, 0.7071067811865475727, 1.000000000000000000) ) ) 
 REPRESENTATION_ITEM ( '' )  SURFACE ( )  );
#41802=AXIS2_PLACEMENT_3D ( 'NONE', #8799, #39314, #39801 ) ;
#41803=CARTESIAN_POINT ( 'NONE',  ( -4.260926853938491021, -13.83313663034587115, 2.750000000000000888 ) ) ;
#41809=PRESENTATION_STYLE_ASSIGNMENT (( #33768 ) ) ;
#41819=DIRECTION ( 'NONE',  ( -0.000000000000000000, 0.000000000000000000, 1.000000000000000000 ) ) ;
#41820=PRESENTATION_STYLE_ASSIGNMENT (( #11299 ) ) ;
#41825=LINE ( 'NONE', #34277, #52858 ) ;
#41853=ADVANCED_FACE ( 'NONE', ( #38459 ), #68952, .F. ) ;
#41854=DIRECTION ( 'NONE',  ( 0.000000000000000000, 0.000000000000000000, -1.000000000000000000 ) ) ;
#41870=CARTESIAN_POINT ( 'NONE',  ( 0.000000000000000000, -97.00000000000000000, -3.750000000000000000 ) ) ;
#41874=FACE_OUTER_BOUND ( 'NONE', #20112, .T. ) ;
#41887=ORIENTED_EDGE ( 'NONE', *, *, #26671, .F. ) ;
#41890=AXIS2_PLACEMENT_3D ( 'NONE', #5523, #83483, #36003 ) ;
#41896=DIRECTION ( 'NONE',  ( -0.06975647374410356982, -0.9975640502598257520, -0.000000000000000000 ) ) ;
#41924=CARTESIAN_POINT ( 'NONE',  ( 11.43651723230273021, -81.64184067850541737, 3.750000000000000888 ) ) ;
#41929=EDGE_CURVE ( 'NONE', #10746, #85496, #72377, .T. ) ;
#41932=SURFACE_STYLE_USAGE ( .BOTH. , #27391 ) ;
#41936=CARTESIAN_POINT ( 'NONE',  ( 0.4400000000000020006, 1.019547802438468986, 2.500000000000000000 ) ) ;
#41938=ORIENTED_EDGE ( 'NONE', *, *, #91561, .F. ) ;
#41939=EDGE_CURVE ( 'NONE', #91147, #48124, #69440, .T. ) ;
#41940=CARTESIAN_POINT ( 'NONE',  ( 6.757940885639631468, -58.32678904743398363, -3.750000000000000000 ) ) ;
#41960=EDGE_LOOP ( 'NONE', ( #23865, #73558, #24271, #3626, #19986, #96263 ) ) ;
#41970=EDGE_CURVE ( 'NONE', #56730, #35739, #67987, .T. ) ;
#41978=FACE_BOUND ( 'NONE', #95947, .T. ) ;
#41987=AXIS2_PLACEMENT_3D ( 'NONE', #5493, #51467, #89466 ) ;
#42000=AXIS2_PLACEMENT_3D ( 'NONE', #5840, #13334, #66825 ) ;
#42007=ORIENTED_EDGE ( 'NONE', *, *, #32274, .F. ) ;
#42020=EDGE_CURVE ( 'NONE', #57591, #35160, #85541, .T. ) ;
#42027=AXIS2_PLACEMENT_3D ( 'NONE', #72116, #95108, #62645 ) ;
#42029=MECHANICAL_DESIGN_GEOMETRIC_PRESENTATION_REPRESENTATION('',(#94684),#3699);
#42032=CARTESIAN_POINT ( 'NONE',  ( -6.732636091893168029, -88.11213685669366669, 3.750000000000000000 ) ) ;
#42048=VERTEX_POINT ( 'NONE', #23950 ) ;
#42057=CARTESIAN_POINT ( 'NONE',  ( -6.829866546992953147, -69.52413922185967010, -2.500000000000000000 ) ) ;
#42062=AXIS2_PLACEMENT_3D ( 'NONE', #89135, #13132, #29978 ) ;
#42063=( NAMED_UNIT ( * ) SI_UNIT ( $, .STERADIAN. ) SOLID_ANGLE_UNIT ( ) );
#42068=CARTESIAN_POINT ( 'NONE',  ( -4.250000000000000000, 36.75000000000000000, -4.000000000000000000 ) ) ;
#42073=CARTESIAN_POINT ( 'NONE',  ( -3.888677292528964102, -8.267505865805661713, -3.750000000000000000 ) ) ;
#42085=DIRECTION ( 'NONE',  ( 1.000000000000000000, 0.000000000000000000, 0.000000000000000000 ) ) ;
#42094=STYLED_ITEM ( 'NONE', ( #6880 ), #96348 ) ;
#42107=AXIS2_PLACEMENT_3D ( 'NONE', #80241, #28718, #89226 ) ;
#42108=FACE_OUTER_BOUND ( 'NONE', #83898, .T. ) ;
#42125=CARTESIAN_POINT ( 'NONE',  ( 17.88942678785190665, 78.22945985324594176, -4.041087757000573433 ) ) ;
#42128=EDGE_LOOP ( 'NONE', ( #98822, #12081, #37729, #24132, #98979, #5166, #48719, #35259, #32530, #85148 ) ) ;
#42132=CARTESIAN_POINT ( 'NONE',  ( 11.35644480889520302, -65.08008077083090370, 4.000000000000000000 ) ) ;
#42140=DIRECTION ( 'NONE',  ( 0.000000000000000000, 0.000000000000000000, 1.000000000000000000 ) ) ;
#42155=VERTEX_POINT ( 'NONE', #65858 ) ;
#42164=EDGE_CURVE ( 'NONE', #76530, #63379, #95381, .T. ) ;
#42166=( NAMED_UNIT ( * ) PLANE_ANGLE_UNIT ( ) SI_UNIT ( $, .RADIAN. ) );
#42171=CARTESIAN_POINT ( 'NONE',  ( -11.20030343255358218, -94.46585862443534154, -3.750000000000000000 ) ) ;
#42173=CARTESIAN_POINT ( 'NONE',  ( 4.380000000000002558, 1.019547802438462547, 2.500000000000000000 ) ) ;
#42187=EDGE_LOOP ( 'NONE', ( #51484, #30337, #81323, #93424 ) ) ;
#42189=CARTESIAN_POINT ( 'NONE',  ( 6.903457398626330566, -84.61157762779829739, 3.750000000000001332 ) ) ;
#42197=CARTESIAN_POINT ( 'NONE',  ( 6.879999999999995453, 43.00000000000000000, 4.250000000000000000 ) ) ;
#42229=CIRCLE ( 'NONE', #707, 0.2500000000000002220 ) ;
#42234=ORIENTED_EDGE ( 'NONE', *, *, #45564, .T. ) ;
#42270=CARTESIAN_POINT ( 'NONE',  ( 6.910409932109719655, -84.29236789247111972, 2.749999999999999556 ) ) ;
#42273=DIRECTION ( 'NONE',  ( 0.000000000000000000, 1.000000000000000000, 0.000000000000000000 ) ) ;
#42278=VECTOR ( 'NONE', #88306, 1000.000000000000000 ) ;
#42285=CARTESIAN_POINT ( 'NONE',  ( -7.124966304139052298, -78.82422094453229988, 2.750000000000000000 ) ) ;
#42296=ORIENTED_EDGE ( 'NONE', *, *, #45407, .T. ) ;
#42297=FACE_OUTER_BOUND ( 'NONE', #18288, .T. ) ;
#42303=CARTESIAN_POINT ( 'NONE',  ( 10.93147959995856944, -92.98161664596344167, -3.999999999999999112 ) ) ;
#42305=PRESENTATION_STYLE_ASSIGNMENT (( #34279 ) ) ;
#42306=SURFACE_STYLE_FILL_AREA ( #71337 ) ;
#42310=UNCERTAINTY_MEASURE_WITH_UNIT (LENGTH_MEASURE( 1.000000000000000082E-05 ), #60788, 'distance_accuracy_value', 'NONE');
#42314=CARTESIAN_POINT ( 'NONE',  ( -6.581680125707233486, -88.31141629936868753, -2.500000000000000000 ) ) ;
#42334=EDGE_CURVE ( 'NONE', #22610, #25163, #56411, .T. ) ;
#42336=ORIENTED_EDGE ( 'NONE', *, *, #11961, .F. ) ;
#42346=ORIENTED_EDGE ( 'NONE', *, *, #40916, .T. ) ;
#42353=EDGE_CURVE ( 'NONE', #46257, #49695, #37656, .T. ) ;
#42369=ORIENTED_EDGE ( 'NONE', *, *, #55560, .T. ) ;
#42371=CARTESIAN_POINT ( 'NONE',  ( 4.782492776157768688, 54.66414256906417535, 3.000000000000000000 ) ) ;
#42376=DIRECTION ( 'NONE',  ( 0.000000000000000000, 1.000000000000000000, 0.000000000000000000 ) ) ;
#42393=DIRECTION ( 'NONE',  ( 0.000000000000000000, 1.000000000000000000, 0.000000000000000000 ) ) ;
#42395=EDGE_CURVE ( 'NONE', #67582, #56519, #48890, .T. ) ;
#42397=CARTESIAN_POINT ( 'NONE',  ( 6.910443788307254032, -84.29081344371353168, 2.500000000014485302 ) ) ;
#42402=CARTESIAN_POINT ( 'NONE',  ( 10.83696084481538691, -98.17058944465519232, 3.750000000000000000 ) ) ;
#42407=ORIENTED_EDGE ( 'NONE', *, *, #64664, .F. ) ;
#42410=CARTESIAN_POINT ( 'NONE',  ( -4.259797194938747644, -13.81744876718660819, -2.500000000001613820 ) ) ;
#42413=CARTESIAN_POINT ( 'NONE',  ( 0.000000000000000000, 84.07179676972448590, -12.00000000000000000 ) ) ;
#42416=CARTESIAN_POINT ( 'NONE',  ( 4.879999999999991900, 76.07179676972444327, 4.250000000000000000 ) ) ;
#42419=FILL_AREA_STYLE ('',( #72899 ) ) ;
#42432=UNCERTAINTY_MEASURE_WITH_UNIT (LENGTH_MEASURE( 1.000000000000000082E-05 ), #21396, 'distance_accuracy_value', 'NONE');
#42433=AXIS2_PLACEMENT_3D ( 'NONE', #55918, #2447, #61923 ) ;
#42442=CARTESIAN_POINT ( 'NONE',  ( 18.00000000000000355, 77.07179676972445748, -4.250000000000000000 ) ) ;
#42476=DIRECTION ( 'NONE',  ( -1.000000000000000000, -0.000000000000000000, -0.000000000000000000 ) ) ;
#42492=DIRECTION ( 'NONE',  ( 0.000000000000000000, -0.000000000000000000, -1.000000000000000000 ) ) ;
#42495=ORIENTED_EDGE ( 'NONE', *, *, #2301, .T. ) ;
#42500=ORIENTED_EDGE ( 'NONE', *, *, #10969, .T. ) ;
#42509=CARTESIAN_POINT ( 'NONE',  ( 6.937721053838227014, -80.66520463107747219, -2.750000000000000000 ) ) ;
#42517=ADVANCED_FACE ( 'NONE', ( #52343 ), #97371, .F. ) ;
#42537=CYLINDRICAL_SURFACE ( 'NONE', #60777, 1.500000000000001332 ) ;
#42543=( GEOMETRIC_REPRESENTATION_CONTEXT ( 3 ) GLOBAL_UNCERTAINTY_ASSIGNED_CONTEXT ( ( #23130 ) ) GLOBAL_UNIT_ASSIGNED_CONTEXT ( ( #20942, #66924, #74918 ) ) REPRESENTATION_CONTEXT ( 'NONE', 'WORKASPACE' ) );
#42547=DIRECTION ( 'NONE',  ( -1.000000000000000000, 0.000000000000000000, 0.000000000000000000 ) ) ;
#42559=FILL_AREA_STYLE_COLOUR ( '', #60212 ) ;
#42561=STYLED_ITEM ( 'NONE', ( #96776 ), #776 ) ;
#42565=EDGE_CURVE ( 'NONE', #75573, #31275, #75334, .T. ) ;
#42567=ORIENTED_EDGE ( 'NONE', *, *, #10740, .F. ) ;
#42572=CARTESIAN_POINT ( 'NONE',  ( 15.00000000000000000, 77.07179676972447169, -6.250000000000000000 ) ) ;
#42583=CARTESIAN_POINT ( 'NONE',  ( 4.219999999999999751, 10.25000000000000000, 2.750000000000000000 ) ) ;
#42585=PRESENTATION_STYLE_ASSIGNMENT (( #20072 ) ) ;
#42592=DIRECTION ( 'NONE',  ( 1.000000000000000000, -0.000000000000000000, 0.000000000000000000 ) ) ;
#42594=( GEOMETRIC_REPRESENTATION_CONTEXT ( 3 ) GLOBAL_UNCERTAINTY_ASSIGNED_CONTEXT ( ( #73158 ) ) GLOBAL_UNIT_ASSIGNED_CONTEXT ( ( #3395, #24928, #85914 ) ) REPRESENTATION_CONTEXT ( 'NONE', 'WORKASPACE' ) );
#42609=AXIS2_PLACEMENT_3D ( 'NONE', #3634, #50100, #72591 ) ;
#42611=VERTEX_POINT ( 'NONE', #52831 ) ;
#42613=CARTESIAN_POINT ( 'NONE',  ( 0.000000000000000000, 0.000000000000000000, -3.000000000000000000 ) ) ;
#42614=CARTESIAN_POINT ( 'NONE',  ( -5.812563760649267941, -35.09659463721938977, 2.750000000000000000 ) ) ;
#42625=CARTESIAN_POINT ( 'NONE',  ( 11.57153612472183646, -43.60599867514397943, -3.750000000000001776 ) ) ;
#42633=AXIS2_PLACEMENT_3D ( 'NONE', #72722, #80735, #12230 ) ;
#42643=FILL_AREA_STYLE ('',( #27631 ) ) ;
#42644=CIRCLE ( 'NONE', #79408, 0.2500000000000002220 ) ;
#42650=CARTESIAN_POINT ( 'NONE',  ( -11.58434547256946168, -69.53046085282417721, -4.000000000003604228 ) ) ;
#42657=( GEOMETRIC_REPRESENTATION_CONTEXT ( 3 ) GLOBAL_UNCERTAINTY_ASSIGNED_CONTEXT ( ( #69258 ) ) GLOBAL_UNIT_ASSIGNED_CONTEXT ( ( #21545, #44526, #90024 ) ) REPRESENTATION_CONTEXT ( 'NONE', 'WORKASPACE' ) );
#42668=DIRECTION ( 'NONE',  ( -1.000000000000000000, -0.000000000000000000, -0.000000000000000000 ) ) ;
#42676=DIRECTION ( 'NONE',  ( -0.5905099943842175847, -0.8070303256584298035, 0.000000000000000000 ) ) ;
#42679=CARTESIAN_POINT ( 'NONE',  ( 0.000000000000000000, 0.000000000000000000, -8.000000000000000000 ) ) ;
#42691=CARTESIAN_POINT ( 'NONE',  ( -16.94999999999999929, 100.0000000000000000, 7.896446609406727823 ) ) ;
#42699=CARTESIAN_POINT ( 'NONE',  ( 9.879999999999991900, 20.99999999999999645, 1.249999999999987121 ) ) ;
#42702=ORIENTED_EDGE ( 'NONE', *, *, #84704, .T. ) ;
#42717=EDGE_CURVE ( 'NONE', #75803, #81788, #32923, .T. ) ;
#42728=ADVANCED_FACE ( 'NONE', ( #16815 ), #32783, .F. ) ;
#42737=CARTESIAN_POINT ( 'NONE',  ( 6.579634127946654587, -87.99828267815715321, -2.750000000000000000 ) ) ;
#42739=CARTESIAN_POINT ( 'NONE',  ( -9.000000000000001776, 80.99999999999994316, -1.249999999999987121 ) ) ;
#42755=ORIENTED_EDGE ( 'NONE', *, *, #1056, .F. ) ;
#42766=DIRECTION ( 'NONE',  ( 0.8070303256584299145, -0.5905099943842175847, 0.000000000000000000 ) ) ;
#42770=CARTESIAN_POINT ( 'NONE',  ( 6.829574850505126804, -88.00372650098204019, 3.750000000000001332 ) ) ;
#42772=EDGE_CURVE ( 'NONE', #54617, #2502, #80823, .T. ) ;
#42776=CARTESIAN_POINT ( 'NONE',  ( 5.129999999999990123, 76.07179676972444327, 6.500000000000000888 ) ) ;
#42783=FACE_OUTER_BOUND ( 'NONE', #70737, .T. ) ;
#42794=MECHANICAL_DESIGN_GEOMETRIC_PRESENTATION_REPRESENTATION('',(#65097),#1290);
#42795=LINE ( 'NONE', #8250, #90458 ) ;
#42797=CARTESIAN_POINT ( 'NONE',  ( 10.58840669699852199, -98.14374106289703548, -4.000000000000000000 ) ) ;
#42804=( GEOMETRIC_REPRESENTATION_CONTEXT ( 3 ) GLOBAL_UNCERTAINTY_ASSIGNED_CONTEXT ( ( #1272 ) ) GLOBAL_UNIT_ASSIGNED_CONTEXT ( ( #83156, #68168, #45652 ) ) REPRESENTATION_CONTEXT ( 'NONE', 'WORKASPACE' ) );
#42820=FACE_OUTER_BOUND ( 'NONE', #60039, .T. ) ;
#42821=ORIENTED_EDGE ( 'NONE', *, *, #44484, .F. ) ;
#42824=ORIENTED_EDGE ( 'NONE', *, *, #95568, .T. ) ;
#42829=DIRECTION ( 'NONE',  ( 0.000000000000000000, 0.000000000000000000, 1.000000000000000000 ) ) ;
#42837=ORIENTED_EDGE ( 'NONE', *, *, #97835, .F. ) ;
#42847=ORIENTED_EDGE ( 'NONE', *, *, #53624, .F. ) ;
#42859=DIRECTION ( 'NONE',  ( -0.9961946980917458783, 0.08715574274765407192, 0.000000000000000000 ) ) ;
#42871=CIRCLE ( 'NONE', #23695, 7.000000000000002665 ) ;
#42890=EDGE_CURVE ( 'NONE', #79587, #49408, #38929, .T. ) ;
#42897=DIRECTION ( 'NONE',  ( 2.569960705150826877E-16, -1.000000000000000000, 0.000000000000000000 ) ) ;
#42898=CARTESIAN_POINT ( 'NONE',  ( -6.982525766850296911, -88.11956318484570261, -2.750000000000000444 ) ) ;
#42905=CARTESIAN_POINT ( 'NONE',  ( 6.034747819266367053, -36.07388523691940918, -3.999999999999999556 ) ) ;
#42908=CARTESIAN_POINT ( 'NONE',  ( -5.580435433942707135, -28.67474180225212166, 4.000000000000000888 ) ) ;
#42910=CARTESIAN_POINT ( 'NONE',  ( 3.969999999999999751, 37.00000000000000000, 4.000000000000000000 ) ) ;
#42911=( GEOMETRIC_REPRESENTATION_CONTEXT ( 3 ) GLOBAL_UNCERTAINTY_ASSIGNED_CONTEXT ( ( #33183 ) ) GLOBAL_UNIT_ASSIGNED_CONTEXT ( ( #3816, #95288, #69246 ) ) REPRESENTATION_CONTEXT ( 'NONE', 'WORKASPACE' ) );
#42916=PLANE ( 'NONE',  #7595 ) ;
#42919=CARTESIAN_POINT ( 'NONE',  ( -0.6999999999999957367, 99.99999999999998579, -8.525133428036873795 ) ) ;
#42921=EDGE_CURVE ( 'NONE', #48471, #17079, #4274, .T. ) ;
#42933=CIRCLE ( 'NONE', #98844, 0.2500000000000002220 ) ;
#42943=ORIENTED_EDGE ( 'NONE', *, *, #80851, .F. ) ;
#42950=CARTESIAN_POINT ( 'NONE',  ( -1.899999999999997247, 98.49999999999998579, 8.000000000000000000 ) ) ;
#42975=ORIENTED_EDGE ( 'NONE', *, *, #77203, .F. ) ;
#42981=CARTESIAN_POINT ( 'NONE',  ( -6.866255446112624838, -80.67934795256483937, 2.500000000000000000 ) ) ;
#42993=AXIS2_PLACEMENT_3D ( 'NONE', #57662, #40344, #63311 ) ;
#43012=EDGE_LOOP ( 'NONE', ( #27909, #4224, #21095, #54821 ) ) ;
#43021=CARTESIAN_POINT ( 'NONE',  ( -5.780262629516635720, -39.80185923444033591, -2.500000000000000000 ) ) ;
#43022=VECTOR ( 'NONE', #47125, 1000.000000000000000 ) ;
#43029=AXIS2_PLACEMENT_3D ( 'NONE', #9981, #48945, #27424 ) ;
#43031=SURFACE_STYLE_USAGE ( .BOTH. , #28017 ) ;
#43035=EDGE_CURVE ( 'NONE', #96234, #76621, #17798, .T. ) ;
#43048=DIRECTION ( 'NONE',  ( -1.000000000000000000, 0.000000000000000000, 0.000000000000000000 ) ) ;
#43059=CARTESIAN_POINT ( 'NONE',  ( 10.93542311823294355, -97.13826248502067529, -3.749999999999999112 ) ) ;
#43072=ORIENTED_EDGE ( 'NONE', *, *, #2208, .F. ) ;
#43074=ORIENTED_EDGE ( 'NONE', *, *, #51136, .F. ) ;
#43104=CARTESIAN_POINT ( 'NONE',  ( 0.000000000000000000, 36.75000000000000000, 2.750000000000000000 ) ) ;
#43105=DIRECTION ( 'NONE',  ( 0.000000000000000000, 0.000000000000000000, 1.000000000000000000 ) ) ;
#43109=ORIENTED_EDGE ( 'NONE', *, *, #68592, .F. ) ;
#43116=EDGE_CURVE ( 'NONE', #37093, #52793, #85799, .T. ) ;
#43133=CARTESIAN_POINT ( 'NONE',  ( -11.33436264776094404, -69.53389133807300482, -4.000000000000000000 ) ) ;
#43141=ADVANCED_FACE ( 'NONE', ( #77790 ), #44312, .T. ) ;
#43154=CARTESIAN_POINT ( 'NONE',  ( 6.937721053838227014, -80.66520463107747219, 2.750000000000000000 ) ) ;
#43164=VECTOR ( 'NONE', #16293, 1000.000000000000000 ) ;
#43183=DIRECTION ( 'NONE',  ( 0.000000000000000000, 1.000000000000000000, 0.000000000000000000 ) ) ;
#43185=AXIS2_PLACEMENT_3D ( 'NONE', #92094, #32566, #32062 ) ;
#43192=CARTESIAN_POINT ( 'NONE',  ( -19.64999999999999858, 98.99999999999998579, -8.000000000000000000 ) ) ;
#43211=DIRECTION ( 'NONE',  ( -1.000000000000000000, 0.000000000000000000, 0.000000000000000000 ) ) ;
#43215=SURFACE_STYLE_FILL_AREA ( #4254 ) ;
#43217=ORIENTED_EDGE ( 'NONE', *, *, #24251, .T. ) ;
#43223=DIRECTION ( 'NONE',  ( -1.000000000000000000, 0.000000000000000000, 0.000000000000000000 ) ) ;
#43224=FACE_OUTER_BOUND ( 'NONE', #49870, .T. ) ;
#43235=EDGE_CURVE ( 'NONE', #63974, #27580, #11263, .T. ) ;
#43244=DIRECTION ( 'NONE',  ( 1.000000000000000000, 0.000000000000000000, 0.000000000000000000 ) ) ;
#43247=CARTESIAN_POINT ( 'NONE',  ( -8.900000000000002132, 80.99999999999994316, -3.000000000000000000 ) ) ;
#43251=CARTESIAN_POINT ( 'NONE',  ( 4.395800986235852470, -0.8373804211230448935, 3.750000000000000000 ) ) ;
#43258=ORIENTED_EDGE ( 'NONE', *, *, #44571, .T. ) ;
#43262=CARTESIAN_POINT ( 'NONE',  ( -12.19495285927234463, 90.49761223356972550, -7.228801115472371031 ) ) ;
#43263=CARTESIAN_POINT ( 'NONE',  ( 8.979999999999991545, 21.00000000000000000, 0.000000000000000000 ) ) ;
#43266=VERTEX_POINT ( 'NONE', #41782 ) ;
#43268=EDGE_CURVE ( 'NONE', #72111, #32092, #23121, .T. ) ;
#43276=CARTESIAN_POINT ( 'NONE',  ( -6.000000000000014211, 80.32179676972448590, 4.000000000000000000 ) ) ;
#43278=CARTESIAN_POINT ( 'NONE',  ( -7.750000000000000000, 41.24999999999999289, 6.250000000000000000 ) ) ;
#43280=DIRECTION ( 'NONE',  ( -0.000000000000000000, 0.000000000000000000, 1.000000000000000000 ) ) ;
#43291=CARTESIAN_POINT ( 'NONE',  ( 17.75000000000000000, 84.07179676972448590, 12.00000000000000000 ) ) ;
#43296=COLOUR_RGB ( '', 0.72549020, 0.75294118, 0.79215686) ;
#43301=VERTEX_POINT ( 'NONE', #58730 ) ;
#43308=DIRECTION ( 'NONE',  ( 0.6246950475544238435, 0.7808688094430307203, 0.000000000000000000 ) ) ;
#43310=DIRECTION ( 'NONE',  ( 0.000000000000000000, 1.000000000000000000, 0.000000000000000000 ) ) ;
#43324=CARTESIAN_POINT ( 'NONE',  ( -7.232415441807423129, -88.12698951299773853, -4.000000000000000000 ) ) ;
#43328=AXIS2_PLACEMENT_3D ( 'NONE', #29375, #59876, #63803 ) ;
#43332=LINE ( 'NONE', #90301, #13208 ) ;
#43347=ORIENTED_EDGE ( 'NONE', *, *, #54627, .F. ) ;
#43350=DIRECTION ( 'NONE',  ( 1.000000000000000000, 0.000000000000000000, 0.000000000000000000 ) ) ;
#43353=FACE_OUTER_BOUND ( 'NONE', #20768, .T. ) ;
#43364=CIRCLE ( 'NONE', #16273, 0.2500000000000002220 ) ;
#43367=EDGE_LOOP ( 'NONE', ( #69066, #28640, #38671, #42824 ) ) ;
#43369=( NAMED_UNIT ( * ) PLANE_ANGLE_UNIT ( ) SI_UNIT ( $, .RADIAN. ) );
#43372=CARTESIAN_POINT ( 'NONE',  ( -7.754989057094396010, 84.52548903604051134, 4.000000000000000888 ) ) ;
#43375=ORIENTED_EDGE ( 'NONE', *, *, #94952, .T. ) ;
#43378=CARTESIAN_POINT ( 'NONE',  ( -6.822528426060553208, -84.39592987140930802, -2.500000000000000000 ) ) ;
#43398=DIRECTION ( 'NONE',  ( -1.000000000000000000, 0.000000000000000000, -0.000000000000000000 ) ) ;
#43401=DIRECTION ( 'NONE',  ( 0.000000000000000000, -1.000000000000000000, 0.000000000000000000 ) ) ;
#43403=VECTOR ( 'NONE', #92742, 1000.000000000000000 ) ;
#43409=VERTEX_POINT ( 'NONE', #67729 ) ;
#43410=DIRECTION ( 'NONE',  ( -1.000000000000000000, 0.000000000000000000, 0.000000000000000000 ) ) ;
#43427=FILL_AREA_STYLE ('',( #59906 ) ) ;
#43436=VECTOR ( 'NONE', #24632, 1000.000000000000000 ) ;
#43472=ADVANCED_FACE ( 'NONE', ( #15230 ), #91705, .T. ) ;
#43473=UNCERTAINTY_MEASURE_WITH_UNIT (LENGTH_MEASURE( 1.000000000000000082E-05 ), #33300, 'distance_accuracy_value', 'NONE');
#43480=CARTESIAN_POINT ( 'NONE',  ( 6.829574850499570360, -88.00372650123708240, -3.750000000000000888 ) ) ;
#43491=( GEOMETRIC_REPRESENTATION_CONTEXT ( 3 ) GLOBAL_UNCERTAINTY_ASSIGNED_CONTEXT ( ( #39255 ) ) GLOBAL_UNIT_ASSIGNED_CONTEXT ( ( #41171, #3163, #79642 ) ) REPRESENTATION_CONTEXT ( 'NONE', 'WORKASPACE' ) );
#43501=CIRCLE ( 'NONE', #70644, 2.999999999999997335 ) ;
#43505=DIRECTION ( 'NONE',  ( -1.000000000000000000, 0.000000000000000000, -0.000000000000000000 ) ) ;
#43515=DIRECTION ( 'NONE',  ( 0.000000000000000000, 0.000000000000000000, -1.000000000000000000 ) ) ;
#43516=CIRCLE ( 'NONE', #88200, 3.750000000000001776 ) ;
#43523=CARTESIAN_POINT ( 'NONE',  ( 17.74999999999999645, 91.00000000000000000, 8.000000000000000000 ) ) ;
#43531=CARTESIAN_POINT ( 'NONE',  ( -6.000000000000009770, 41.24999999999999289, -6.250000000000000000 ) ) ;
#43539=CARTESIAN_POINT ( 'NONE',  ( -3.836050625226794963, -2.701282487336928106, -4.000000000000000000 ) ) ;
#43540=ORIENTED_EDGE ( 'NONE', *, *, #77203, .T. ) ;
#43541=COLOUR_RGB ( '', 0.40784314, 0.44705882, 0.49803922) ;
#43555=EDGE_LOOP ( 'NONE', ( #83298, #41605, #22842 ) ) ;
#43563=CARTESIAN_POINT ( 'NONE',  ( -3.499999999999998668, 1.019547802438465434, 3.750000000000000000 ) ) ;
#43564=ADVANCED_FACE ( 'NONE', ( #60214 ), #39567, .T. ) ;
#43567=ORIENTED_EDGE ( 'NONE', *, *, #64664, .T. ) ;
#43586=EDGE_CURVE ( 'NONE', #49831, #24464, #22014, .T. ) ;
#43588=ORIENTED_EDGE ( 'NONE', *, *, #22580, .F. ) ;
#43596=CARTESIAN_POINT ( 'NONE',  ( -3.500000492100954652, 0.08994223334896143951, 3.750000000000000444 ) ) ;
#43597=( NAMED_UNIT ( * ) SI_UNIT ( $, .STERADIAN. ) SOLID_ANGLE_UNIT ( ) );
#43618=CARTESIAN_POINT ( 'NONE',  ( -3.500000000000000444, -0.04521315095527938394, -2.750000000000000444 ) ) ;
#43621=CARTESIAN_POINT ( 'NONE',  ( -4.250000000000000000, 78.07179676972445748, -6.250000000000000000 ) ) ;
#43627=CARTESIAN_POINT ( 'NONE',  ( -11.07532115276637086, -96.02567358741556802, -3.750000000000000000 ) ) ;
#43632=( LENGTH_UNIT ( ) NAMED_UNIT ( * ) SI_UNIT ( .MILLI., .METRE. ) );
#43643=( GEOMETRIC_REPRESENTATION_CONTEXT ( 3 ) GLOBAL_UNCERTAINTY_ASSIGNED_CONTEXT ( ( #30437 ) ) GLOBAL_UNIT_ASSIGNED_CONTEXT ( ( #9479, #24996, #63460 ) ) REPRESENTATION_CONTEXT ( 'NONE', 'WORKASPACE' ) );
#43652=AXIS2_PLACEMENT_3D ( 'NONE', #43531, #6526, #75021 ) ;
#43656=CARTESIAN_POINT ( 'NONE',  ( 4.129999999999999893, 0.09092508111800794157, 2.499999999999999112 ) ) ;
#43660=FILL_AREA_STYLE ('',( #97680 ) ) ;
#43677=VERTEX_POINT ( 'NONE', #46685 ) ;
#43678=EDGE_LOOP ( 'NONE', ( #61568, #95626, #89706, #16610 ) ) ;
#43684=EDGE_CURVE ( 'NONE', #53272, #36801, #75931, .T. ) ;
#43686=EDGE_CURVE ( 'NONE', #24464, #3878, #79459, .T. ) ;
#43689=ORIENTED_EDGE ( 'NONE', *, *, #24868, .F. ) ;
#43700=LINE ( 'NONE', #21711, #79923 ) ;
#43702=DIRECTION ( 'NONE',  ( -0.08715574274766037244, -0.9961946980917453232, -0.000000000000000000 ) ) ;
#43711=VECTOR ( 'NONE', #81126, 1000.000000000000000 ) ;
#43714=VERTEX_POINT ( 'NONE', #78169 ) ;
#43723=CARTESIAN_POINT ( 'NONE',  ( 6.579634127946650146, -87.99828267815715321, -2.750000000000000000 ) ) ;
#43740=DIRECTION ( 'NONE',  ( 1.000000000000000000, 0.000000000000000000, 0.000000000000000000 ) ) ;
#43744=CARTESIAN_POINT ( 'NONE',  ( 0.000000000000000000, 10.25000000000000000, 2.750000000000000000 ) ) ;
#43754=CARTESIAN_POINT ( 'NONE',  ( 17.75000000000001776, 4.561680251642722724E-15, 4.000000000000000000 ) ) ;
#43758=ORIENTED_EDGE ( 'NONE', *, *, #14272, .T. ) ;
#43775=CARTESIAN_POINT ( 'NONE',  ( -8.000000000000000000, 0.000000000000000000, -6.250000000000000000 ) ) ;
#43783=CARTESIAN_POINT ( 'NONE',  ( 6.660464271194198815, -84.28715080305920537, -2.500000000000000444 ) ) ;
#43811=DIRECTION ( 'NONE',  ( 0.000000000000000000, 0.000000000000000000, 1.000000000000000000 ) ) ;
#43823=DIRECTION ( 'NONE',  ( 0.000000000000000000, -0.000000000000000000, -1.000000000000000000 ) ) ;
#43839=SURFACE_SIDE_STYLE ('',( #34368 ) ) ;
#43862=VECTOR ( 'NONE', #68371, 1000.000000000000000 ) ;
#43865=DIRECTION ( 'NONE',  ( -1.000000000000000000, -0.000000000000000000, -0.000000000000000000 ) ) ;
#43872=SURFACE_SIDE_STYLE ('',( #21392 ) ) ;
#43873=DIRECTION ( 'NONE',  ( 0.06975647374412534407, 0.9975640502598241977, -0.000000000000000000 ) ) ;
#43878=CARTESIAN_POINT ( 'NONE',  ( -8.099999999999999645, 75.73428692542562146, 2.900000000000000355 ) ) ;
#43886=AXIS2_PLACEMENT_3D ( 'NONE', #34574, #26121, #66067 ) ;
#43911=EDGE_CURVE ( 'NONE', #14317, #66694, #40906, .T. ) ;
#43912=CARTESIAN_POINT ( 'NONE',  ( 4.630000000000001670, 1.019547802438464545, 4.000000000000000000 ) ) ;
#43913=( LENGTH_UNIT ( ) NAMED_UNIT ( * ) SI_UNIT ( .MILLI., .METRE. ) );
#43919=CIRCLE ( 'NONE', #40731, 0.2500000000000002220 ) ;
#43920=ADVANCED_FACE ( 'NONE', ( #50625 ), #87630, .F. ) ;
#43941=EDGE_CURVE ( 'NONE', #27291, #79587, #10566, .T. ) ;
#43951=DIRECTION ( 'NONE',  ( -0.1073935270325955676, -0.9942165912674659767, -0.000000000000000000 ) ) ;
#43952=CARTESIAN_POINT ( 'NONE',  ( 11.04805072375712705, -95.57913125338676252, 3.750000000000000000 ) ) ;
#43955=LINE ( 'NONE', #12484, #59766 ) ;
#43957=CIRCLE ( 'NONE', #894, 0.2500000000000002220 ) ;
#43976=CARTESIAN_POINT ( 'NONE',  ( 18.00000000000000355, 78.65116054140185042, 3.749999999999999112 ) ) ;
#43980=AXIS2_PLACEMENT_3D ( 'NONE', #93481, #70992, #32968 ) ;
#43987=CIRCLE ( 'NONE', #29640, 0.1000000000000001166 ) ;
#44028=CARTESIAN_POINT ( 'NONE',  ( -4.000000000000000000, 10.00000000000000000, 2.750000000000000000 ) ) ;
#44030=SURFACE_STYLE_FILL_AREA ( #73539 ) ;
#44050=DIRECTION ( 'NONE',  ( -0.000000000000000000, -0.000000000000000000, -1.000000000000000000 ) ) ;
#44079=CARTESIAN_POINT ( 'NONE',  ( -7.072466569316883778, -84.40185462517210624, 3.750000000000001776 ) ) ;
#44090=FACE_OUTER_BOUND ( 'NONE', #36197, .T. ) ;
#44094=ORIENTED_EDGE ( 'NONE', *, *, #92595, .T. ) ;
#44100=DIRECTION ( 'NONE',  ( -1.000000000000000000, 0.000000000000000000, 0.000000000000000000 ) ) ;
#44111=( GEOMETRIC_REPRESENTATION_CONTEXT ( 3 ) GLOBAL_UNCERTAINTY_ASSIGNED_CONTEXT ( ( #4182 ) ) GLOBAL_UNIT_ASSIGNED_CONTEXT ( ( #71788, #11772, #58747 ) ) REPRESENTATION_CONTEXT ( 'NONE', 'WORKASPACE' ) );
#44113=CARTESIAN_POINT ( 'NONE',  ( 14.99999999999997868, 80.07179676972448590, 6.250000000000000000 ) ) ;
#44125=ORIENTED_EDGE ( 'NONE', *, *, #46064, .F. ) ;
#44127=( NAMED_UNIT ( * ) SI_UNIT ( $, .STERADIAN. ) SOLID_ANGLE_UNIT ( ) );
#44140=VECTOR ( 'NONE', #76923, 1000.000000000000000 ) ;
#44145=AXIS2_PLACEMENT_3D ( 'NONE', #39080, #70556, #83593 ) ;
#44151=CARTESIAN_POINT ( 'NONE',  ( -11.42361443046363512, -90.30744058745631264, 3.999999999999998224 ) ) ;
#44157=FACE_OUTER_BOUND ( 'NONE', #51426, .T. ) ;
#44161=ORIENTED_EDGE ( 'NONE', *, *, #32879, .F. ) ;
#44180=ORIENTED_EDGE ( 'NONE', *, *, #22261, .T. ) ;
#44190=CARTESIAN_POINT ( 'NONE',  ( 11.34661744925197624, 54.08985607419764818, -2.899999999999999467 ) ) ;
#44195=FACE_BOUND ( 'NONE', #48344, .T. ) ;
#44207=( NAMED_UNIT ( * ) PLANE_ANGLE_UNIT ( ) SI_UNIT ( $, .RADIAN. ) );
#44213=AXIS2_PLACEMENT_3D ( 'NONE', #40044, #93031, #26027 ) ;
#44219=ORIENTED_EDGE ( 'NONE', *, *, #85750, .T. ) ;
#44231=CYLINDRICAL_SURFACE ( 'NONE', #84111, 0.2500000000000002220 ) ;
#44241=ORIENTED_EDGE ( 'NONE', *, *, #10969, .F. ) ;
#44247=CARTESIAN_POINT ( 'NONE',  ( -13.87912815710419068, 90.90967772850538609, -7.772688653987088969 ) ) ;
#44255=CARTESIAN_POINT ( 'NONE',  ( 11.35644985442049659, -65.08036738587416892, -3.750000000000000000 ) ) ;
#44265=ADVANCED_FACE ( 'NONE', ( #82100 ), #97631, .F. ) ;
#44277=STYLED_ITEM ( 'NONE', ( #35487 ), #89872 ) ;
#44286=ORIENTED_EDGE ( 'NONE', *, *, #18061, .F. ) ;
#44293=CIRCLE ( 'NONE', #25194, 0.2500000000000002220 ) ;
#44301=VERTEX_POINT ( 'NONE', #59100 ) ;
#44311=EDGE_CURVE ( 'NONE', #59298, #69763, #53085, .T. ) ;
#44312=( BOUNDED_SURFACE ( )  B_SPLINE_SURFACE ( 3, 2, ( 
 ( #32282, #47788, #62290 ),
 ( #86784, #85306, #47289 ),
 ( #25791, #93289, #70807 ),
 ( #1341, #2324, #9301 ),
 ( #93781, #46804, #48275 ),
 ( #41301, #64248, #78788 ),
 ( #56288, #39811, #70313 ),
 ( #55289, #10294, #71774 ),
 ( #94765, #40793, #18286 ),
 ( #48767, #1829, #79274 ),
 ( #16320, #84813, #77296 ),
 ( #39320, #69817, #31792 ),
 ( #19260, #65232, #87258 ),
 ( #18782, #3785, #65732 ),
 ( #56764, #95250, #96259 ),
 ( #79765, #64738, #4763 ),
 ( #20248, #73727, #20743 ),
 ( #4270, #81718, #28233 ) ),
 .UNSPECIFIED., .F., .F., .F. ) 
 B_SPLINE_SURFACE_WITH_KNOTS ( ( 4, 2, 2, 2, 2, 2, 2, 2, 4 ),
 ( 3, 3 ),
 ( 0.000000000000000000, 0.001371970262341174959, 0.002743940524682349918, 0.004115910787023524878, 0.005487881049364699837, 0.006859851311705874796, 0.008231821574047049755, 0.009603791836388224715, 0.01097576209872939967 ),
 ( 0.000000000000000000, 1.000000000000000000 ),
 .UNSPECIFIED. ) 
 GEOMETRIC_REPRESENTATION_ITEM ( )  RATIONAL_B_SPLINE_SURFACE ( (
 ( 1.000000000000000000, 0.7071067811865475727, 1.000000000000000000),
 ( 1.000000000000000000, 0.7072982590433614103, 1.000000000000000000),
 ( 1.000000000000000000, 0.7113498972295660971, 1.000000000000000000),
 ( 1.000000000000000000, 0.7257703676791772418, 1.000000000000000000),
 ( 1.000000000000000000, 0.7362840324263598690, 1.000000000000000000),
 ( 1.000000000000000000, 0.7606319170830569965, 1.000000000000000000),
 ( 1.000000000000000000, 0.7745485803766045674, 1.000000000000000000),
 ( 1.000000000000000000, 0.8036690257212466548, 1.000000000000000000),
 ( 1.000000000000000000, 0.8185245023542137011, 1.000000000000000000),
 ( 1.000000000000000000, 0.8475516512718134221, 1.000000000000000000),
 ( 1.000000000000000000, 0.8617420886046480710, 1.000000000000000000),
 ( 1.000000000000000000, 0.8886174597630145389, 1.000000000000000000),
 ( 1.000000000000000000, 0.9010211234293969973, 1.000000000000000000),
 ( 1.000000000000000000, 0.9233336449993967410, 1.000000000000000000),
 ( 1.000000000000000000, 0.9332564696566055806, 1.000000000000000000),
 ( 1.000000000000000000, 0.9500370447729021839, 1.000000000000000000),
 ( 1.000000000000000000, 0.9567390024732228548, 1.000000000000000000),
 ( 1.000000000000000000, 0.9611621933234234527, 1.000000000000000000) ) ) 
 REPRESENTATION_ITEM ( '' )  SURFACE ( )  );
#44313=ORIENTED_EDGE ( 'NONE', *, *, #24514, .F. ) ;
#44331=AXIS2_PLACEMENT_3D ( 'NONE', #28053, #29032, #52531 ) ;
#44333=FILL_AREA_STYLE_COLOUR ( '', #66182 ) ;
#44343=CARTESIAN_POINT ( 'NONE',  ( -9.886043635230025828, 89.00072246145502675, -5.688751881067946492 ) ) ;
#44356=VECTOR ( 'NONE', #29715, 1000.000000000000000 ) ;
#44363=ORIENTED_EDGE ( 'NONE', *, *, #5326, .T. ) ;
#44365=ADVANCED_FACE ( 'NONE', ( #76084 ), #38107, .T. ) ;
#44366=EDGE_CURVE ( 'NONE', #87849, #43677, #26028, .T. ) ;
#44377=LINE ( 'NONE', #94060, #79741 ) ;
#44379=( NAMED_UNIT ( * ) SI_UNIT ( $, .STERADIAN. ) SOLID_ANGLE_UNIT ( ) );
#44383=PRESENTATION_STYLE_ASSIGNMENT (( #13898 ) ) ;
#44397=LINE ( 'NONE', #6395, #86147 ) ;
#44408=FACE_OUTER_BOUND ( 'NONE', #91857, .T. ) ;
#44410=AXIS2_PLACEMENT_3D ( 'NONE', #10001, #26952, #33456 ) ;
#44414=CARTESIAN_POINT ( 'NONE',  ( 4.471658927162282637, -3.629165645957387554, 4.000000000000000000 ) ) ;
#44415=DIRECTION ( 'NONE',  ( 1.000000000000000000, 0.000000000000000000, 0.000000000000000000 ) ) ;
#44419=DIRECTION ( 'NONE',  ( -0.000000000000000000, -0.000000000000000000, 1.000000000000000000 ) ) ;
#44434=MECHANICAL_DESIGN_GEOMETRIC_PRESENTATION_REPRESENTATION('',(#10892),#73188);
#44437=VERTEX_POINT ( 'NONE', #25075 ) ;
#44441=CARTESIAN_POINT ( 'NONE',  ( 9.879999999999988347, 26.99999999999999645, 2.900000000000000355 ) ) ;
#44453=CARTESIAN_POINT ( 'NONE',  ( 10.64411726291637450, -97.62798956704561704, 4.000000000000000000 ) ) ;
#44455=ORIENTED_EDGE ( 'NONE', *, *, #5791, .F. ) ;
#44457=CARTESIAN_POINT ( 'NONE',  ( 4.721516313243696139, -3.620689210586678364, 4.000000000000000000 ) ) ;
#44467=CARTESIAN_POINT ( 'NONE',  ( -13.72545693419366764, 90.95708220729730442, -7.926564183086028059 ) ) ;
#44470=CIRCLE ( 'NONE', #20500, 0.5000000000000004441 ) ;
#44473=EDGE_CURVE ( 'NONE', #39466, #7185, #20722, .T. ) ;
#44484=EDGE_CURVE ( 'NONE', #72885, #93468, #36714, .T. ) ;
#44487=CARTESIAN_POINT ( 'NONE',  ( 17.99999999999999645, 91.28723161455539525, 8.000000000000000000 ) ) ;
#44488=EDGE_CURVE ( 'NONE', #50168, #27600, #33476, .T. ) ;
#44496=STYLED_ITEM ( 'NONE', ( #37099 ), #13790 ) ;
#44503=VERTEX_POINT ( 'NONE', #55557 ) ;
#44506=CIRCLE ( 'NONE', #57269, 0.2500000000000002220 ) ;
#44513=CARTESIAN_POINT ( 'NONE',  ( 6.432108699068924018, -88.20011490510430008, 2.500000000000000000 ) ) ;
#44514=DIRECTION ( 'NONE',  ( -0.000000000000000000, -0.000000000000000000, -1.000000000000000000 ) ) ;
#44520=EDGE_CURVE ( 'NONE', #76760, #96670, #9068, .T. ) ;
#44526=( NAMED_UNIT ( * ) PLANE_ANGLE_UNIT ( ) SI_UNIT ( $, .RADIAN. ) );
#44530=CARTESIAN_POINT ( 'NONE',  ( 8.992292137164646704, -4.149411823827444223, -3.749999999999999556 ) ) ;
#44531=EDGE_CURVE ( 'NONE', #20984, #83910, #18667, .T. ) ;
#44532=CARTESIAN_POINT ( 'NONE',  ( -6.857667818334720167, -50.95147662124758625, -4.000000000000000000 ) ) ;
#44540=CARTESIAN_POINT ( 'NONE',  ( 8.879999999999995453, 41.24999999999999289, 4.250000000000000000 ) ) ;
#44545=DIRECTION ( 'NONE',  ( 0.000000000000000000, -1.000000000000000000, 0.000000000000000000 ) ) ;
#44547=CARTESIAN_POINT ( 'NONE',  ( 8.879999999999991900, 69.99999999999998579, 4.000000000000000000 ) ) ;
#44551=LINE ( 'NONE', #52545, #92464 ) ;
#44571=EDGE_CURVE ( 'NONE', #64978, #76530, #88222, .T. ) ;
#44574=DIRECTION ( 'NONE',  ( 1.000000000000000000, -0.000000000000000000, -0.000000000000000000 ) ) ;
#44576=CARTESIAN_POINT ( 'NONE',  ( 8.630000000000000782, -0.01512149801896540274, 4.000000000000000000 ) ) ;
#44583=CYLINDRICAL_SURFACE ( 'NONE', #50848, 0.2500000000000002220 ) ;
#44584=FACE_OUTER_BOUND ( 'NONE', #52687, .T. ) ;
#44595=AXIS2_PLACEMENT_3D ( 'NONE', #15320, #37816, #45300 ) ;
#44599=CARTESIAN_POINT ( 'NONE',  ( 0.000000000000000000, -97.00000000000000000, 4.000000000000000000 ) ) ;
#44602=VERTEX_POINT ( 'NONE', #38588 ) ;
#44618=DIRECTION ( 'NONE',  ( 0.9961946980917462113, -0.08715574274765140739, 0.000000000000000000 ) ) ;
#44632=VERTEX_POINT ( 'NONE', #8579 ) ;
#44634=SURFACE_STYLE_USAGE ( .BOTH. , #29615 ) ;
#44644=ORIENTED_EDGE ( 'NONE', *, *, #63120, .T. ) ;
#44655=CARTESIAN_POINT ( 'NONE',  ( -10.85644721466729123, -98.10785618530077556, 3.999999999999093614 ) ) ;
#44664=VERTEX_POINT ( 'NONE', #62055 ) ;
#44670=DIRECTION ( 'NONE',  ( 1.483861936729427615E-16, -1.000000000000000000, 0.000000000000000000 ) ) ;
#44675=DIRECTION ( 'NONE',  ( 0.08715574274766037244, 0.9961946980917453232, -0.000000000000000000 ) ) ;
#44676=COLOUR_RGB ( '', 0.31764706, 0.68627451, 0.89019608) ;
#44692=CARTESIAN_POINT ( 'NONE',  ( -7.750000000000000000, 41.24999999999999289, -6.250000000000000000 ) ) ;
#44693=ORIENTED_EDGE ( 'NONE', *, *, #27032, .T. ) ;
#44697=DIRECTION ( 'NONE',  ( 0.000000000000000000, 0.000000000000000000, -1.000000000000000000 ) ) ;
#44707=( LENGTH_UNIT ( ) NAMED_UNIT ( * ) SI_UNIT ( .MILLI., .METRE. ) );
#44713=SHAPE_DEFINITION_REPRESENTATION ( #97154, #51695 ) ;
#44725=CARTESIAN_POINT ( 'NONE',  ( 6.879999999999995453, 43.00000000000000000, -6.250000000000000000 ) ) ;
#44733=AXIS2_PLACEMENT_3D ( 'NONE', #30168, #83683, #15198 ) ;
#44743=DIRECTION ( 'NONE',  ( 1.000000000000000000, 0.000000000000000000, 0.000000000000000000 ) ) ;
#44748=CARTESIAN_POINT ( 'NONE',  ( 11.18126922403858003, -92.99194761433179224, -3.750000000000000000 ) ) ;
#44773=LINE ( 'NONE', #13796, #29940 ) ;
#44776=DIRECTION ( 'NONE',  ( 0.000000000000000000, 1.000000000000000000, 0.000000000000000000 ) ) ;
#44792=EDGE_LOOP ( 'NONE', ( #76784, #96448, #2013, #8095, #92420, #7148, #60130, #93235 ) ) ;
#44793=ORIENTED_EDGE ( 'NONE', *, *, #33985, .F. ) ;
#44813=DIRECTION ( 'NONE',  ( 0.000000000000000000, -1.000000000000000000, 0.000000000000000000 ) ) ;
#44816=COLOUR_RGB ( '', 0.08235294, 0.09019608, 0.10196078) ;
#44817=SURFACE_SIDE_STYLE ('',( #21348 ) ) ;
#44823=VECTOR ( 'NONE', #96747, 1000.000000000000000 ) ;
#44825=CARTESIAN_POINT ( 'NONE',  ( 4.395712687474492952, -0.8323168403830496498, -2.500000000000000888 ) ) ;
#44829=EDGE_CURVE ( 'NONE', #23534, #6552, #84481, .T. ) ;
#44831=DIRECTION ( 'NONE',  ( -0.000000000000000000, -0.000000000000000000, -1.000000000000000000 ) ) ;
#44833=EDGE_CURVE ( 'NONE', #49656, #79731, #84963, .T. ) ;
#44860=ORIENTED_EDGE ( 'NONE', *, *, #90416, .T. ) ;
#44861=CARTESIAN_POINT ( 'NONE',  ( -13.69999999999999751, 99.99999999999998579, -8.000000000000000000 ) ) ;
#44862=VECTOR ( 'NONE', #32465, 1000.000000000000000 ) ;
#44868=CARTESIAN_POINT ( 'NONE',  ( -7.750000000000000000, 80.32179676972448590, -4.250000000000000000 ) ) ;
#44890=ORIENTED_EDGE ( 'NONE', *, *, #39564, .T. ) ;
#44896=SURFACE_SIDE_STYLE ('',( #60890 ) ) ;
#44901=CARTESIAN_POINT ( 'NONE',  ( 7.185087194272973932, -80.58596676771932721, 4.000000000000000000 ) ) ;
#44902=AXIS2_PLACEMENT_3D ( 'NONE', #78436, #48429, #10441 ) ;
#44903=( NAMED_UNIT ( * ) PLANE_ANGLE_UNIT ( ) SI_UNIT ( $, .RADIAN. ) );
#44904=CARTESIAN_POINT ( 'NONE',  ( 8.879999999999991900, 20.99999999999999645, 0.000000000000000000 ) ) ;
#44923=COLOUR_RGB ( '', 0.40784314, 0.44705882, 0.49803922) ;
#44924=CARTESIAN_POINT ( 'NONE',  ( 0.000000000000000000, 80.32179676972448590, -4.000000000000000000 ) ) ;
#44934=CIRCLE ( 'NONE', #75284, 0.2500000000000002220 ) ;
#44943=CARTESIAN_POINT ( 'NONE',  ( 8.629999999999995453, 40.99999999999999289, 6.500000000000000888 ) ) ;
#44945=ORIENTED_EDGE ( 'NONE', *, *, #14029, .T. ) ;
#44949=EDGE_CURVE ( 'NONE', #48124, #18106, #28803, .T. ) ;
#44959=CARTESIAN_POINT ( 'NONE',  ( -5.999999999999994671, 43.00000000000000000, -6.250000000000000000 ) ) ;
#44961=CARTESIAN_POINT ( 'NONE',  ( 6.533420211785746723, -50.31490269211863620, -2.750000000000000000 ) ) ;
#44969=( NAMED_UNIT ( * ) SI_UNIT ( $, .STERADIAN. ) SOLID_ANGLE_UNIT ( ) );
#44974=AXIS2_PLACEMENT_3D ( 'NONE', #86332, #17836, #33309 ) ;
#44993=EDGE_CURVE ( 'NONE', #33828, #75926, #40463, .T. ) ;
#45011=CARTESIAN_POINT ( 'NONE',  ( 4.219999999999999751, 37.00000000000000000, 3.750000000000000000 ) ) ;
#45014=CARTESIAN_POINT ( 'NONE',  ( -8.000000000000000000, 40.74999999999999289, -3.750000000000000000 ) ) ;
#45018=CARTESIAN_POINT ( 'NONE',  ( 8.880000000000002558, -0.01511739988658945127, -3.750000000000000888 ) ) ;
#45019=CARTESIAN_POINT ( 'NONE',  ( -7.124934413296625912, -78.83349193436581004, -3.750000000000000888 ) ) ;
#45038=ORIENTED_EDGE ( 'NONE', *, *, #74963, .T. ) ;
#45058=CYLINDRICAL_SURFACE ( 'NONE', #18441, 0.2500000000000002220 ) ;
#45063=CARTESIAN_POINT ( 'NONE',  ( 11.18664512644303599, -81.61943089664755746, 4.000000000000000888 ) ) ;
#45069=PRESENTATION_STYLE_ASSIGNMENT (( #46072 ) ) ;
#45078=CARTESIAN_POINT ( 'NONE',  ( 17.75000000000000355, 73.00000000000001421, -6.500000000000000888 ) ) ;
#45083=CARTESIAN_POINT ( 'NONE',  ( 17.74999999999999645, 91.00000000000000000, 8.000000000000000000 ) ) ;
#45103=LINE ( 'NONE', #6620, #70789 ) ;
#45129=ADVANCED_FACE ( 'NONE', ( #4437 ), #97493, .T. ) ;
#45141=CARTESIAN_POINT ( 'NONE',  ( -10.57481851842510778, -40.44832046089882738, 4.000000000000000000 ) ) ;
#45153=ORIENTED_EDGE ( 'NONE', *, *, #59281, .T. ) ;
#45154=DIRECTION ( 'NONE',  ( 0.000000000000000000, -0.000000000000000000, -1.000000000000000000 ) ) ;
#45157=SURFACE_SIDE_STYLE ('',( #29648 ) ) ;
#45159=VERTEX_POINT ( 'NONE', #79436 ) ;
#45170=ADVANCED_FACE ( 'NONE', ( #71926 ), #48436, .T. ) ;
#45171=ORIENTED_EDGE ( 'NONE', *, *, #49895, .F. ) ;
#45192=PRESENTATION_STYLE_ASSIGNMENT (( #91179 ) ) ;
#45196=DIRECTION ( 'NONE',  ( 0.08715574274765112983, 0.9961946980917461003, 0.000000000000000000 ) ) ;
#45198=EDGE_CURVE ( 'NONE', #41466, #11855, #60782, .T. ) ;
#45199=DIRECTION ( 'NONE',  ( 1.000000000000000000, 0.000000000000000000, 0.000000000000000000 ) ) ;
#45213=DIRECTION ( 'NONE',  ( -0.000000000000000000, 0.000000000000000000, 1.000000000000000000 ) ) ;
#45215=AXIS2_PLACEMENT_3D ( 'NONE', #1066, #31530, #70533 ) ;
#45231=FILL_AREA_STYLE ('',( #52728 ) ) ;
#45248=CARTESIAN_POINT ( 'NONE',  ( 10.64413412520849000, -97.62783346105426574, -4.000000000000000000 ) ) ;
#45257=( NAMED_UNIT ( * ) SI_UNIT ( $, .STERADIAN. ) SOLID_ANGLE_UNIT ( ) );
#45260=AXIS2_PLACEMENT_3D ( 'NONE', #25697, #70205, #17214 ) ;
#45263=UNCERTAINTY_MEASURE_WITH_UNIT (LENGTH_MEASURE( 1.000000000000000082E-05 ), #11799, 'distance_accuracy_value', 'NONE');
#45272=DIRECTION ( 'NONE',  ( -0.000000000000000000, -0.000000000000000000, 1.000000000000000000 ) ) ;
#45279=PRESENTATION_STYLE_ASSIGNMENT (( #45783 ) ) ;
#45280=ORIENTED_EDGE ( 'NONE', *, *, #74271, .T. ) ;
#45298=ORIENTED_EDGE ( 'NONE', *, *, #80851, .T. ) ;
#45300=DIRECTION ( 'NONE',  ( 0.000000000000000000, 0.000000000000000000, 1.000000000000000000 ) ) ;
#45307=ORIENTED_EDGE ( 'NONE', *, *, #13086, .F. ) ;
#45319=( NAMED_UNIT ( * ) PLANE_ANGLE_UNIT ( ) SI_UNIT ( $, .RADIAN. ) );
#45320=DIRECTION ( 'NONE',  ( 0.000000000000000000, 0.000000000000000000, -1.000000000000000000 ) ) ;
#45331=CARTESIAN_POINT ( 'NONE',  ( 4.669733657687698880, -13.81599790086176682, -2.499999999999999112 ) ) ;
#45340=CARTESIAN_POINT ( 'NONE',  ( -19.89999999999999858, 0.000000000000000000, 7.750000000000000000 ) ) ;
#45344=CARTESIAN_POINT ( 'NONE',  ( -7.750000000000000000, 83.99999999999994316, -4.000000000000000000 ) ) ;
#45346=CARTESIAN_POINT ( 'NONE',  ( -8.468261785982759804, -9.345432893194818291, -4.000000000000000000 ) ) ;
#45360=ORIENTED_EDGE ( 'NONE', *, *, #7540, .F. ) ;
#45368=DIRECTION ( 'NONE',  ( 1.000000000000000000, 1.257402221000611116E-16, -0.000000000000000000 ) ) ;
#45384=FACE_OUTER_BOUND ( 'NONE', #18502, .T. ) ;
#45397=CARTESIAN_POINT ( 'NONE',  ( 7.184035427668765017, -73.16388022040806050, 4.000000000000000000 ) ) ;
#45398=EDGE_CURVE ( 'NONE', #16419, #76530, #51397, .T. ) ;
#45407=EDGE_CURVE ( 'NONE', #65307, #88822, #11245, .T. ) ;
#45440=CARTESIAN_POINT ( 'NONE',  ( 7.079515573063599021, -88.00917032380691296, -4.000000000000000000 ) ) ;
#45449=CARTESIAN_POINT ( 'NONE',  ( -11.88860330016272471, 90.28199325633934791, 6.828299344291659523 ) ) ;
#45457=CARTESIAN_POINT ( 'NONE',  ( 4.380000000000000782, -0.01592157648205478476, -2.750000000000000000 ) ) ;
#45472=LINE ( 'NONE', #81994, #36371 ) ;
#45480=CYLINDRICAL_SURFACE ( 'NONE', #22862, 0.2500000000000002220 ) ;
#45492=DIRECTION ( 'NONE',  ( 1.000000000000000000, 0.000000000000000000, 0.000000000000000000 ) ) ;
#45500=DIRECTION ( 'NONE',  ( 0.000000000000000000, -1.000000000000000000, 0.000000000000000000 ) ) ;
#45503=ORIENTED_EDGE ( 'NONE', *, *, #63879, .F. ) ;
#45510=DIRECTION ( 'NONE',  ( 1.000000000000000000, 0.000000000000000000, 0.000000000000000000 ) ) ;
#45518=CARTESIAN_POINT ( 'NONE',  ( -7.116171662378945051, -80.69120418497870162, -3.749999999999193534 ) ) ;
#45519=VERTEX_POINT ( 'NONE', #75371 ) ;
#45523=TOROIDAL_SURFACE ( 'NONE', #90259, 2.250000000000001332, 0.2500000000000000000 ) ;
#45537=ORIENTED_EDGE ( 'NONE', *, *, #13242, .T. ) ;
#45539=ORIENTED_EDGE ( 'NONE', *, *, #81939, .F. ) ;
#45549=CIRCLE ( 'NONE', #18428, 0.09999999999999982514 ) ;
#45555=CARTESIAN_POINT ( 'NONE',  ( -8.000000000000000000, 40.99999999999999289, -6.500000000000000888 ) ) ;
#45557=ORIENTED_EDGE ( 'NONE', *, *, #40621, .T. ) ;
#45564=EDGE_CURVE ( 'NONE', #65197, #91549, #71919, .T. ) ;
#45566=CARTESIAN_POINT ( 'NONE',  ( 11.04397247052727238, -89.88416767676933716, 4.000000000000000888 ) ) ;
#45574=CARTESIAN_POINT ( 'NONE',  ( 9.050000000000002487, 99.99999999999998579, -8.525133428036873795 ) ) ;
#45577=DIRECTION ( 'NONE',  ( -2.107602052970795044E-16, 1.000000000000000000, 0.000000000000000000 ) ) ;
#45596=CARTESIAN_POINT ( 'NONE',  ( 6.879999999999995453, 79.82179676972448590, -6.500000000000000888 ) ) ;
#45598=LINE ( 'NONE', #92087, #19872 ) ;
#45605=ADVANCED_FACE ( 'NONE', ( #66388 ), #52870, .T. ) ;
#45609=DIRECTION ( 'NONE',  ( 0.000000000000000000, -1.000000000000000000, 0.000000000000000000 ) ) ;
#45616=EDGE_CURVE ( 'NONE', #40405, #35851, #63977, .T. ) ;
#45617=EDGE_CURVE ( 'NONE', #43266, #54617, #78407, .T. ) ;
#45622=ORIENTED_EDGE ( 'NONE', *, *, #93597, .F. ) ;
#45625=( LENGTH_UNIT ( ) NAMED_UNIT ( * ) SI_UNIT ( .MILLI., .METRE. ) );
#45636=ORIENTED_EDGE ( 'NONE', *, *, #43684, .F. ) ;
#45645=CARTESIAN_POINT ( 'NONE',  ( -8.647950603528085978, -15.58161425315045534, 4.000000000000000000 ) ) ;
#45652=( NAMED_UNIT ( * ) SI_UNIT ( $, .STERADIAN. ) SOLID_ANGLE_UNIT ( ) );
#45659=CARTESIAN_POINT ( 'NONE',  ( -6.000000000000014211, 79.82179676972448590, -6.500000000000000888 ) ) ;
#45686=DIRECTION ( 'NONE',  ( 1.000000000000000000, 0.000000000000000000, 0.000000000000000000 ) ) ;
#45687=DIRECTION ( 'NONE',  ( 1.000000000000000000, 3.828355257328124777E-15, 0.000000000000000000 ) ) ;
#45688=ORIENTED_EDGE ( 'NONE', *, *, #96782, .F. ) ;
#45689=FILL_AREA_STYLE ('',( #15210 ) ) ;
#45711=( GEOMETRIC_REPRESENTATION_CONTEXT ( 3 ) GLOBAL_UNCERTAINTY_ASSIGNED_CONTEXT ( ( #10210 ) ) GLOBAL_UNIT_ASSIGNED_CONTEXT ( ( #67804, #10253, #87216 ) ) REPRESENTATION_CONTEXT ( 'NONE', 'WORKASPACE' ) );
#45721=SURFACE_STYLE_FILL_AREA ( #30698 ) ;
#45723=CARTESIAN_POINT ( 'NONE',  ( -7.199999999999996625, 99.99999999999998579, 8.000000000000000000 ) ) ;
#45752=CARTESIAN_POINT ( 'NONE',  ( 10.72174155808380647, -40.27583460510356161, -3.999999999992825739 ) ) ;
#45756=( NAMED_UNIT ( * ) PLANE_ANGLE_UNIT ( ) SI_UNIT ( $, .RADIAN. ) );
#45769=DIRECTION ( 'NONE',  ( -0.9961946980917462113, 0.08715574274765114371, 0.000000000000000000 ) ) ;
#45774=CARTESIAN_POINT ( 'NONE',  ( 0.000000000000000000, 99.74999999999998579, 8.000000000000000000 ) ) ;
#45776=STYLED_ITEM ( 'NONE', ( #22427 ), #30522 ) ;
#45779=CARTESIAN_POINT ( 'NONE',  ( 4.323020469702378854, -6.401304200487259344, -2.500000000000000888 ) ) ;
#45781=EDGE_CURVE ( 'NONE', #67494, #44632, #56020, .T. ) ;
#45783=SURFACE_STYLE_USAGE ( .BOTH. , #15783 ) ;
#45794=VERTEX_POINT ( 'NONE', #93330 ) ;
#45796=VECTOR ( 'NONE', #39676, 1000.000000000000000 ) ;
#45800=EDGE_LOOP ( 'NONE', ( #11148, #42369, #75239, #26909 ) ) ;
#45830=EDGE_CURVE ( 'NONE', #86107, #69763, #40094, .T. ) ;
#45839=CARTESIAN_POINT ( 'NONE',  ( 4.572805492040462383, -6.390838093309134216, -2.750000000000000000 ) ) ;
#45852=CARTESIAN_POINT ( 'NONE',  ( -7.750000002551292511, -0.02148553728220452957, -4.000000000000000000 ) ) ;
#45870=FILL_AREA_STYLE_COLOUR ( '', #34065 ) ;
#45910=CARTESIAN_POINT ( 'NONE',  ( 6.910361961229144256, -84.29457034759302303, 3.999999999998390177 ) ) ;
#45914=CARTESIAN_POINT ( 'NONE',  ( -4.511864039100093926, -13.83704418182126972, -4.000000000000000888 ) ) ;
#45931=ORIENTED_EDGE ( 'NONE', *, *, #58025, .F. ) ;
#45936=AXIS2_PLACEMENT_3D ( 'NONE', #97698, #38170, #68657 ) ;
#45950=ORIENTED_EDGE ( 'NONE', *, *, #93444, .T. ) ;
#45952=B_SPLINE_CURVE_WITH_KNOTS ( 'NONE', 3,
 ( #94782, #27263, #57273, #88760, #42285, #48786, #19769, #27758, #34766, #88266, #79295, #4292, #33763, #26775, #41803, #87767, #64271, #49283, #73260, #26282, #56783, #86804 ),
 .UNSPECIFIED., .F., .F.,
 ( 4, 2, 2, 2, 2, 2, 2, 2, 2, 2, 4 ),
 ( 0.000000000000000000, 0.005577058028141766884, 0.01115411605628353377, 0.02230823211256706753, 0.04461646422513413507, 0.05577058028141766016, 0.06692469633770119219, 0.07807881239398470341, 0.08365587042212647984, 0.08644439943619736111, 0.08923292845026822850 ),
 .UNSPECIFIED. ) ;
#45962=CARTESIAN_POINT ( 'NONE',  ( -13.51649600052862610, 90.98605788696677621, -7.975941444417872894 ) ) ;
#45965=CARTESIAN_POINT ( 'NONE',  ( 6.599999999999995204, -97.00000000000000000, -4.000000000000000000 ) ) ;
#45977=EDGE_CURVE ( 'NONE', #35759, #8190, #85131, .T. ) ;
#45987=DIRECTION ( 'NONE',  ( 0.009903002720634835818, -0.9999509640662961329, 0.000000000000000000 ) ) ;
#46001=AXIS2_PLACEMENT_3D ( 'NONE', #42572, #48587, #26574 ) ;
#46009=ORIENTED_EDGE ( 'NONE', *, *, #18553, .T. ) ;
#46011=CARTESIAN_POINT ( 'NONE',  ( -16.94999999999999574, 99.74999999999998579, -8.000000000000000000 ) ) ;
#46018=EDGE_CURVE ( 'NONE', #92377, #35492, #41825, .T. ) ;
#46025=CARTESIAN_POINT ( 'NONE',  ( -7.287642027973244119, -86.26866148728002770, -4.000000000000000000 ) ) ;
#46026=( GEOMETRIC_REPRESENTATION_CONTEXT ( 3 ) GLOBAL_UNCERTAINTY_ASSIGNED_CONTEXT ( ( #70239 ) ) GLOBAL_UNIT_ASSIGNED_CONTEXT ( ( #33948, #25511, #86500 ) ) REPRESENTATION_CONTEXT ( 'NONE', 'WORKASPACE' ) );
#46061=CARTESIAN_POINT ( 'NONE',  ( -7.750000000000000000, 0.000000000000000000, 3.750000000000000000 ) ) ;
#46064=EDGE_CURVE ( 'NONE', #44503, #41466, #87300, .T. ) ;
#46066=DIRECTION ( 'NONE',  ( -1.000000000000000000, 0.000000000000000000, 0.000000000000000000 ) ) ;
#46068=ORIENTED_EDGE ( 'NONE', *, *, #98045, .T. ) ;
#46072=SURFACE_STYLE_USAGE ( .BOTH. , #61550 ) ;
#46074=CARTESIAN_POINT ( 'NONE',  ( -49.20731707317072079, 39.36585365853652974, -8.000000000000000000 ) ) ;
#46079=CARTESIAN_POINT ( 'NONE',  ( -11.64999999999999680, 98.49999999999998579, -8.000000000000000000 ) ) ;
#46083=COLOUR_RGB ( '', 0.09019608, 0.27058824, 0.51372549) ;
#46088=CARTESIAN_POINT ( 'NONE',  ( 8.879999999999991900, 27.04366094290857347, -2.958578643762691307 ) ) ;
#46091=VERTEX_POINT ( 'NONE', #33784 ) ;
#46098=CARTESIAN_POINT ( 'NONE',  ( -6.982525766139714207, -88.11956320875633253, -2.750000000000000444 ) ) ;
#46100=ADVANCED_FACE ( 'NONE', ( #56804 ), #38458, .F. ) ;
#46108=SURFACE_STYLE_FILL_AREA ( #22625 ) ;
#46115=LINE ( 'NONE', #21646, #58443 ) ;
#46130=CARTESIAN_POINT ( 'NONE',  ( -18.89999999999999147, 99.74999999999998579, 8.000000000000000000 ) ) ;
#46142=CARTESIAN_POINT ( 'NONE',  ( -11.33063469435185233, -84.07074358190932628, 4.000000000000000000 ) ) ;
#46157=CARTESIAN_POINT ( 'NONE',  ( -3.750000000000000000, 36.75000000000000000, 2.750000000000000000 ) ) ;
#46164=STYLED_ITEM ( 'NONE', ( #96589 ), #60234 ) ;
#46180=COLOUR_RGB ( '', 0.09019608, 0.27058824, 0.51372549) ;
#46182=CARTESIAN_POINT ( 'NONE',  ( 18.00000000000001776, 4.625929269271493211E-15, 6.250000000000000000 ) ) ;
#46183=ORIENTED_EDGE ( 'NONE', *, *, #60667, .T. ) ;
#46186=LINE ( 'NONE', #37223, #24438 ) ;
#46188=CARTESIAN_POINT ( 'NONE',  ( 8.880000001785997910, -0.01162444801712644513, 4.000000000009423573 ) ) ;
#46191=CARTESIAN_POINT ( 'NONE',  ( 3.969999999999999751, 36.75000000000000000, -2.500000000000000000 ) ) ;
#46195=ORIENTED_EDGE ( 'NONE', *, *, #11246, .F. ) ;
#46206=DIRECTION ( 'NONE',  ( -0.000000000000000000, -0.000000000000000000, -1.000000000000000000 ) ) ;
#46218=DIRECTION ( 'NONE',  ( -1.000000000000000000, 2.081668171172167567E-14, 0.000000000000000000 ) ) ;
#46226=DIRECTION ( 'NONE',  ( -0.5905099943842175847, -0.8070303256584298035, 0.000000000000000000 ) ) ;
#46232=ORIENTED_EDGE ( 'NONE', *, *, #5791, .T. ) ;
#46243=CARTESIAN_POINT ( 'NONE',  ( 11.18665108219126125, -81.61837458707562121, -4.000000000000000000 ) ) ;
#46245=AXIS2_PLACEMENT_3D ( 'NONE', #43878, #89881, #50400 ) ;
#46251=( NAMED_UNIT ( * ) SI_UNIT ( $, .STERADIAN. ) SOLID_ANGLE_UNIT ( ) );
#46257=VERTEX_POINT ( 'NONE', #43276 ) ;
#46260=DIRECTION ( 'NONE',  ( -1.000000000000000000, 0.000000000000000000, 0.000000000000000000 ) ) ;
#46272=CARTESIAN_POINT ( 'NONE',  ( -3.522141228719769757, -0.8488377518989214110, 4.000000000000402345 ) ) ;
#46275=ORIENTED_EDGE ( 'NONE', *, *, #87293, .T. ) ;
#46281=( NAMED_UNIT ( * ) PLANE_ANGLE_UNIT ( ) SI_UNIT ( $, .RADIAN. ) );
#46286=FACE_OUTER_BOUND ( 'NONE', #76406, .T. ) ;
#46296=ADVANCED_FACE ( 'NONE', ( #48068 ), #57631, .T. ) ;
#46303=EDGE_CURVE ( 'NONE', #40303, #46764, #17599, .T. ) ;
#46311=CARTESIAN_POINT ( 'NONE',  ( 50.81170089112749366, 69.44265788454083577, -8.000000000000000000 ) ) ;
#46312=CARTESIAN_POINT ( 'NONE',  ( -3.771484078448132937, -6.414704524388527673, -2.750000000000000444 ) ) ;
#46323=CARTESIAN_POINT ( 'NONE',  ( 4.919406150865614613, -13.80316667494924054, -2.749999999999999556 ) ) ;
#46328=EDGE_CURVE ( 'NONE', #89237, #94114, #25111, .T. ) ;
#46333=AXIS2_PLACEMENT_3D ( 'NONE', #15244, #60225, #23731 ) ;
#46338=CARTESIAN_POINT ( 'NONE',  ( -8.897294703381261272, -15.56348197610850725, -4.000000000000000000 ) ) ;
#46346=CARTESIAN_POINT ( 'NONE',  ( -4.249999999999994671, 43.00000000000000711, -6.250000000000000000 ) ) ;
#46360=PLANE ( 'NONE',  #67006 ) ;
#46366=DIRECTION ( 'NONE',  ( 1.000000000000000000, 0.000000000000000000, 0.000000000000000000 ) ) ;
#46370=AXIS2_PLACEMENT_3D ( 'NONE', #7145, #13650, #14661 ) ;
#46382=EDGE_CURVE ( 'NONE', #37612, #45159, #286, .T. ) ;
#46387=ORIENTED_EDGE ( 'NONE', *, *, #26671, .T. ) ;
#46392=ORIENTED_EDGE ( 'NONE', *, *, #91320, .F. ) ;
#46395=CARTESIAN_POINT ( 'NONE',  ( 3.969999999999999751, 10.00000000000000000, -3.750000000000000000 ) ) ;
#46412=CIRCLE ( 'NONE', #28833, 0.2500000000000002220 ) ;
#46433=CARTESIAN_POINT ( 'NONE',  ( 4.219999999999999751, 36.75000000000000000, -2.750000000000000000 ) ) ;
#46435=ADVANCED_FACE ( 'NONE', ( #94073 ), #41088, .T. ) ;
#46438=AXIS2_PLACEMENT_3D ( 'NONE', #53867, #62330, #84854 ) ;
#46447=CARTESIAN_POINT ( 'NONE',  ( 6.452519493965914954, -47.68837976023561964, -3.750000000000000888 ) ) ;
#46450=LINE ( 'NONE', #38959, #89770 ) ;
#46462=( NAMED_UNIT ( * ) SI_UNIT ( $, .STERADIAN. ) SOLID_ANGLE_UNIT ( ) );
#46463=FACE_OUTER_BOUND ( 'NONE', #61533, .T. ) ;
#46476=ORIENTED_EDGE ( 'NONE', *, *, #21654, .F. ) ;
#46478=COLOUR_RGB ( '', 0.08235294, 0.09019608, 0.10196078) ;
#46481=STYLED_ITEM ( 'NONE', ( #39473 ), #79694 ) ;
#46486=CARTESIAN_POINT ( 'NONE',  ( 4.629999999999995453, 43.00000000000000711, -4.250000000000000000 ) ) ;
#46501=CIRCLE ( 'NONE', #32136, 0.1000000000000001166 ) ;
#46528=EDGE_CURVE ( 'NONE', #13075, #77672, #20543, .T. ) ;
#46535=FACE_OUTER_BOUND ( 'NONE', #43678, .T. ) ;
#46537=ORIENTED_EDGE ( 'NONE', *, *, #52742, .T. ) ;
#46543=STYLED_ITEM ( 'NONE', ( #53838 ), #39083 ) ;
#46548=MECHANICAL_DESIGN_GEOMETRIC_PRESENTATION_REPRESENTATION('',(#88081),#62523);
#46553=CARTESIAN_POINT ( 'NONE',  ( 8.629999999999995453, 41.24999999999999289, -6.250000000000000000 ) ) ;
#46565=FILL_AREA_STYLE_COLOUR ( '', #34577 ) ;
#46567=DIRECTION ( 'NONE',  ( -0.000000000000000000, 0.000000000000000000, 1.000000000000000000 ) ) ;
#46578=DIRECTION ( 'NONE',  ( 1.000000000000000000, 0.000000000000000000, 0.000000000000000000 ) ) ;
#46580=DIRECTION ( 'NONE',  ( 1.000000000000000000, 0.000000000000000000, 0.000000000000000000 ) ) ;
#46589=LINE ( 'NONE', #94548, #30274 ) ;
#46602=DIRECTION ( 'NONE',  ( 1.000000000000000000, 0.000000000000000000, 0.000000000000000000 ) ) ;
#46610=ADVANCED_FACE ( 'NONE', ( #80550 ), #36026, .F. ) ;
#46614=ORIENTED_EDGE ( 'NONE', *, *, #73494, .F. ) ;
#46620=CARTESIAN_POINT ( 'NONE',  ( -10.07339213344192963, -32.14942050451718814, 3.750000000000000000 ) ) ;
#46630=DIRECTION ( 'NONE',  ( -0.000000000000000000, 0.000000000000000000, 1.000000000000000000 ) ) ;
#46632=ORIENTED_EDGE ( 'NONE', *, *, #74543, .F. ) ;
#46646=ADVANCED_FACE ( 'NONE', ( #95046 ), #89528, .F. ) ;
#46665=( NAMED_UNIT ( * ) PLANE_ANGLE_UNIT ( ) SI_UNIT ( $, .RADIAN. ) );
#46667=LINE ( 'NONE', #8673, #89963 ) ;
#46670=CARTESIAN_POINT ( 'NONE',  ( 6.880000000000009663, 41.24999999999999289, 6.250000000000000000 ) ) ;
#46685=CARTESIAN_POINT ( 'NONE',  ( -6.599999999999995204, -97.00000000000000000, 4.000000000000000000 ) ) ;
#46702=PLANE ( 'NONE',  #48467 ) ;
#46712=DIRECTION ( 'NONE',  ( 0.000000000000000000, -0.000000000000000000, -1.000000000000000000 ) ) ;
#46718=ORIENTED_EDGE ( 'NONE', *, *, #31371, .F. ) ;
#46752=CARTESIAN_POINT ( 'NONE',  ( -7.232415441807423129, -88.12698951299773853, 4.000000000000000000 ) ) ;
#46754=LINE ( 'NONE', #32233, #82611 ) ;
#46764=VERTEX_POINT ( 'NONE', #60989 ) ;
#46772=DIRECTION ( 'NONE',  ( 1.000000000000000000, 0.000000000000000000, 0.000000000000000000 ) ) ;
#46777=COLOUR_RGB ( '', 0.40784314, 0.44705882, 0.49803922) ;
#46794=FILL_AREA_STYLE_COLOUR ( '', #80345 ) ;
#46804=CARTESIAN_POINT ( 'NONE',  ( -8.331109669465192269, 86.16998870897720053, 4.268594137767635743 ) ) ;
#46817=FILL_AREA_STYLE ('',( #36869 ) ) ;
#46818=VECTOR ( 'NONE', #41683, 1000.000000000000000 ) ;
#46820=CARTESIAN_POINT ( 'NONE',  ( -8.000000000000000000, 1.019547802438466100, -3.750000000000000000 ) ) ;
#46822=CIRCLE ( 'NONE', #80377, 0.2500000000000002220 ) ;
#46835=ORIENTED_EDGE ( 'NONE', *, *, #58471, .T. ) ;
#46836=CARTESIAN_POINT ( 'NONE',  ( -3.750000000000000000, 10.25000000000000000, -4.000000000000000000 ) ) ;
#46872=ORIENTED_EDGE ( 'NONE', *, *, #22261, .F. ) ;
#46875=EDGE_LOOP ( 'NONE', ( #7106, #81107, #85543, #39665 ) ) ;
#46911=LINE ( 'NONE', #44943, #44140 ) ;
#46913=ORIENTED_EDGE ( 'NONE', *, *, #8602, .F. ) ;
#46916=CIRCLE ( 'NONE', #8604, 4.000000000000001776 ) ;
#46921=AXIS2_PLACEMENT_3D ( 'NONE', #80140, #3672, #74108 ) ;
#46926=CARTESIAN_POINT ( 'NONE',  ( 3.969999999999999751, 9.750000000000000000, -3.750000000000000000 ) ) ;
#46927=CARTESIAN_POINT ( 'NONE',  ( 4.903136312256997087, -13.39483660680936339, -3.750000000000000888 ) ) ;
#46946=PLANE ( 'NONE',  #88693 ) ;
#46949=DIRECTION ( 'NONE',  ( 0.000000000000000000, -0.000000000000000000, -1.000000000000000000 ) ) ;
#46951=CARTESIAN_POINT ( 'NONE',  ( 4.380000000000000782, 0.08775168532224617013, -3.750000000000000000 ) ) ;
#46961=DIRECTION ( 'NONE',  ( 0.06975647374410356982, 0.9975640502598257520, -0.000000000000000000 ) ) ;
#46974=CARTESIAN_POINT ( 'NONE',  ( 14.99999999999997868, 80.07179676972448590, 4.250000000000000000 ) ) ;
#46996=DIRECTION ( 'NONE',  ( -0.000000000000000000, 0.000000000000000000, 1.000000000000000000 ) ) ;
#47002=EDGE_CURVE ( 'NONE', #19346, #48651, #40482, .T. ) ;
#47029=FILL_AREA_STYLE ('',( #31533 ) ) ;
#47032=ORIENTED_EDGE ( 'NONE', *, *, #14001, .F. ) ;
#47034=VERTEX_POINT ( 'NONE', #65928 ) ;
#47044=FILL_AREA_STYLE_COLOUR ( '', #37096 ) ;
#47053=CARTESIAN_POINT ( 'NONE',  ( 15.00000000000000000, 77.07179676972447169, -4.000000000000000000 ) ) ;
#47057=EDGE_LOOP ( 'NONE', ( #29847, #56308, #72217, #74701 ) ) ;
#47063=CARTESIAN_POINT ( 'NONE',  ( -6.757332319902496387, -55.97232334539076959, -3.750000000000000000 ) ) ;
#47065=( LENGTH_UNIT ( ) NAMED_UNIT ( * ) SI_UNIT ( .MILLI., .METRE. ) );
#47074=DIRECTION ( 'NONE',  ( 0.000000000000000000, -0.000000000000000000, 1.000000000000000000 ) ) ;
#47075=CARTESIAN_POINT ( 'NONE',  ( -7.909656208964993773, -4.175824794491008518, 4.000000000000000000 ) ) ;
#47080=EDGE_CURVE ( 'NONE', #35357, #35809, #60990, .T. ) ;
#47081=AXIS2_PLACEMENT_3D ( 'NONE', #46346, #54324, #869 ) ;
#47084=ADVANCED_FACE ( 'NONE', ( #29404 ), #92215, .T. ) ;
#47113=CARTESIAN_POINT ( 'NONE',  ( -3.999999999999994671, 43.00000000000000711, -6.250000000000000000 ) ) ;
#47116=ORIENTED_EDGE ( 'NONE', *, *, #32860, .T. ) ;
#47118=CARTESIAN_POINT ( 'NONE',  ( -3.750000000000000000, 37.00000000000000000, 3.750000000000000000 ) ) ;
#47125=DIRECTION ( 'NONE',  ( -0.000000000000000000, 0.000000000000000000, 1.000000000000000000 ) ) ;
#47127=AXIS2_PLACEMENT_3D ( 'NONE', #62784, #74208, #96750 ) ;
#47144=AXIS2_PLACEMENT_3D ( 'NONE', #13470, #43951, #58460 ) ;
#47146=CARTESIAN_POINT ( 'NONE',  ( -3.770608837274703973, -6.399801140530443355, 2.500000000000806910 ) ) ;
#47150=FACE_OUTER_BOUND ( 'NONE', #82185, .T. ) ;
#47151=LINE ( 'NONE', #69677, #37963 ) ;
#47158=LINE ( 'NONE', #77662, #12852 ) ;
#47166=( GEOMETRIC_REPRESENTATION_CONTEXT ( 3 ) GLOBAL_UNCERTAINTY_ASSIGNED_CONTEXT ( ( #33313 ) ) GLOBAL_UNIT_ASSIGNED_CONTEXT ( ( #81747, #28262, #21265 ) ) REPRESENTATION_CONTEXT ( 'NONE', 'WORKASPACE' ) );
#47175=FILL_AREA_STYLE_COLOUR ( '', #57129 ) ;
#47188=AXIS2_PLACEMENT_3D ( 'NONE', #47484, #10964, #94456 ) ;
#47193=ORIENTED_EDGE ( 'NONE', *, *, #38922, .T. ) ;
#47195=EDGE_CURVE ( 'NONE', #93468, #2418, #369, .T. ) ;
#47222=CARTESIAN_POINT ( 'NONE',  ( -10.77730536144846596, -98.63085534186639336, 3.750000000000000000 ) ) ;
#47236=CARTESIAN_POINT ( 'NONE',  ( -6.982525766850296023, -88.11956318484570261, 4.000000000000000000 ) ) ;
#47238=ORIENTED_EDGE ( 'NONE', *, *, #95076, .F. ) ;
#47251=EDGE_LOOP ( 'NONE', ( #12770, #51867, #31607, #78217 ) ) ;
#47255=ORIENTED_EDGE ( 'NONE', *, *, #42921, .T. ) ;
#47268=CIRCLE ( 'NONE', #32927, 1.500000000000001332 ) ;
#47269=CARTESIAN_POINT ( 'NONE',  ( 8.629999999999995453, 40.99999999999999289, -6.250000000000000000 ) ) ;
#47278=FILL_AREA_STYLE ('',( #86280 ) ) ;
#47279=DIRECTION ( 'NONE',  ( -0.000000000000000000, -0.000000000000000000, -1.000000000000000000 ) ) ;
#47289=CARTESIAN_POINT ( 'NONE',  ( -8.004790597918161055, 84.51838969325523010, 3.750000002001242283 ) ) ;
#47304=CARTESIAN_POINT ( 'NONE',  ( -7.750000000000000000, 1.019547802438466100, -4.000000000000000000 ) ) ;
#47312=CARTESIAN_POINT ( 'NONE',  ( 6.879999999999995453, 43.00000000000000000, -6.250000000000000000 ) ) ;
#47315=( GEOMETRIC_REPRESENTATION_CONTEXT ( 3 ) GLOBAL_UNCERTAINTY_ASSIGNED_CONTEXT ( ( #56454 ) ) GLOBAL_UNIT_ASSIGNED_CONTEXT ( ( #43913, #44903, #59411 ) ) REPRESENTATION_CONTEXT ( 'NONE', 'WORKASPACE' ) );
#47333=SURFACE_SIDE_STYLE ('',( #86334 ) ) ;
#47355=CIRCLE ( 'NONE', #20240, 0.2500000000000002220 ) ;
#47360=VECTOR ( 'NONE', #11982, 1000.000000000000000 ) ;
#47368=FACE_OUTER_BOUND ( 'NONE', #31770, .T. ) ;
#47401=CARTESIAN_POINT ( 'NONE',  ( 9.779999999999990479, 20.99999999999999645, -3.000000000000000000 ) ) ;
#47403=ADVANCED_FACE ( 'NONE', ( #53291 ), #15806, .F. ) ;
#47406=CARTESIAN_POINT ( 'NONE',  ( 11.59936910322016423, 56.97882069866371069, 0.000000000000000000 ) ) ;
#47409=CARTESIAN_POINT ( 'NONE',  ( -13.80105244023572197, 90.89655890636302615, 7.750000000000543565 ) ) ;
#47410=CIRCLE ( 'NONE', #95311, 0.2500000000000002220 ) ;
#47439=EDGE_CURVE ( 'NONE', #74806, #81557, #54560, .T. ) ;
#47442=FILL_AREA_STYLE ('',( #32435 ) ) ;
#47448=FILL_AREA_STYLE_COLOUR ( '', #59624 ) ;
#47472=CARTESIAN_POINT ( 'NONE',  ( -6.982525766850298687, -88.11956318484570261, 2.750000000000000444 ) ) ;
#47484=CARTESIAN_POINT ( 'NONE',  ( 8.629999999999995453, 41.24999999999999289, 4.250000000000000000 ) ) ;
#47485=ORIENTED_EDGE ( 'NONE', *, *, #10178, .T. ) ;
#47514=ORIENTED_EDGE ( 'NONE', *, *, #78155, .F. ) ;
#47539=DIRECTION ( 'NONE',  ( 1.000000000000000000, 0.000000000000000000, 0.000000000000000000 ) ) ;
#47549=SURFACE_SIDE_STYLE ('',( #24075 ) ) ;
#47555=DIRECTION ( 'NONE',  ( 1.000000000000000000, 0.000000000000000000, 0.000000000000000000 ) ) ;
#47557=DIRECTION ( 'NONE',  ( -6.938893903907222067E-15, 1.000000000000000000, 0.000000000000000000 ) ) ;
#47558=COLOUR_RGB ( '', 0.40784314, 0.44705882, 0.49803922) ;
#47572=AXIS2_PLACEMENT_3D ( 'NONE', #29162, #90156, #69640 ) ;
#47579=DIRECTION ( 'NONE',  ( 1.000000000000000000, 0.000000000000000000, 0.000000000000000000 ) ) ;
#47581=CARTESIAN_POINT ( 'NONE',  ( -11.01435017114802406, -93.41041245699096862, 4.000000000000000000 ) ) ;
#47599=CARTESIAN_POINT ( 'NONE',  ( -7.750000000000000000, 80.07179676972448590, -6.250000000000000000 ) ) ;
#47605=FILL_AREA_STYLE ('',( #92603 ) ) ;
#47626=SURFACE_SIDE_STYLE ('',( #26113 ) ) ;
#47635=FACE_OUTER_BOUND ( 'NONE', #63668, .T. ) ;
#47636=VECTOR ( 'NONE', #63953, 1000.000000000000000 ) ;
#47642=ORIENTED_EDGE ( 'NONE', *, *, #56902, .F. ) ;
#47650=COLOUR_RGB ( '', 0.08235294, 0.09019608, 0.10196078) ;
#47657=DIRECTION ( 'NONE',  ( 1.000000000000000000, 0.000000000000000000, 0.000000000000000000 ) ) ;
#47661=FILL_AREA_STYLE ('',( #39685 ) ) ;
#47663=FACE_OUTER_BOUND ( 'NONE', #82092, .T. ) ;
#47668=ORIENTED_EDGE ( 'NONE', *, *, #78572, .F. ) ;
#47669=DIRECTION ( 'NONE',  ( 1.000000000000000000, 0.000000000000000000, 0.000000000000000000 ) ) ;
#47676=ORIENTED_EDGE ( 'NONE', *, *, #3989, .T. ) ;
#47682=DIRECTION ( 'NONE',  ( 0.000000000000000000, 0.000000000000000000, -1.000000000000000000 ) ) ;
#47709=CARTESIAN_POINT ( 'NONE',  ( 8.880000000000000782, 1.019547802438459216, -4.000000000000000000 ) ) ;
#47721=VERTEX_POINT ( 'NONE', #80625 ) ;
#47722=FACE_OUTER_BOUND ( 'NONE', #2406, .T. ) ;
#47736=CARTESIAN_POINT ( 'NONE',  ( -6.281594481404161989, -39.81112291747235332, 3.999999999999999112 ) ) ;
#47741=EDGE_LOOP ( 'NONE', ( #17288, #21930, #17987, #44180, #3496, #35103 ) ) ;
#47745=EDGE_CURVE ( 'NONE', #93854, #35809, #6757, .T. ) ;
#47746=DIRECTION ( 'NONE',  ( 0.000000000000000000, 1.000000000000000000, -0.000000000000000000 ) ) ;
#47751=VERTEX_POINT ( 'NONE', #65104 ) ;
#47753=ORIENTED_EDGE ( 'NONE', *, *, #24985, .T. ) ;
#47756=AXIS2_PLACEMENT_3D ( 'NONE', #46926, #84454, #92430 ) ;
#47778=CARTESIAN_POINT ( 'NONE',  ( -7.124967621222336511, -78.82395726652279677, -2.750000000000000888 ) ) ;
#47788=CARTESIAN_POINT ( 'NONE',  ( -8.000343251535923628, 84.06932101904432386, 4.000000000000000000 ) ) ;
#47791=DIRECTION ( 'NONE',  ( 0.000000000000000000, 0.000000000000000000, 1.000000000000000000 ) ) ;
#47800=EDGE_CURVE ( 'NONE', #59298, #86107, #57613, .T. ) ;
#47804=DIRECTION ( 'NONE',  ( 1.000000000000000000, 0.000000000000000000, 0.000000000000000000 ) ) ;
#47808=( LENGTH_UNIT ( ) NAMED_UNIT ( * ) SI_UNIT ( .MILLI., .METRE. ) );
#47823=VECTOR ( 'NONE', #7360, 1000.000000000000000 ) ;
#47827=CYLINDRICAL_SURFACE ( 'NONE', #92156, 0.2500000000000002220 ) ;
#47828=CARTESIAN_POINT ( 'NONE',  ( -4.000000000000000000, 37.25000000000000000, 3.750000000000000000 ) ) ;
#47847=EDGE_LOOP ( 'NONE', ( #60555, #40652, #54533, #77526 ) ) ;
#47865=CIRCLE ( 'NONE', #17557, 0.5000000000000004441 ) ;
#47872=AXIS2_PLACEMENT_3D ( 'NONE', #2788, #24293, #32749 ) ;
#47889=CARTESIAN_POINT ( 'NONE',  ( -11.02747836460322084, -96.55788089094548354, 3.750000000000000444 ) ) ;
#47891=DIRECTION ( 'NONE',  ( -0.1073935270325955676, -0.9942165912674659767, 0.000000000000000000 ) ) ;
#47895=FACE_OUTER_BOUND ( 'NONE', #42128, .T. ) ;
#47897=ORIENTED_EDGE ( 'NONE', *, *, #1883, .T. ) ;
#47926=CARTESIAN_POINT ( 'NONE',  ( -5.559677335903118411, -36.09286816789838781, -2.500000000000000888 ) ) ;
#47927=CARTESIAN_POINT ( 'NONE',  ( 8.880000000000020322, 79.82179676972448590, 6.250000000000000000 ) ) ;
#47930=CARTESIAN_POINT ( 'NONE',  ( -8.124115902427741176, 75.04369783535875627, 3.000000000000000000 ) ) ;
#47934=SURFACE_SIDE_STYLE ('',( #34899 ) ) ;
#47968=EDGE_CURVE ( 'NONE', #61498, #49656, #43501, .T. ) ;
#47986=CARTESIAN_POINT ( 'NONE',  ( -8.000000000000000000, 80.32179676972448590, 4.250000000000000000 ) ) ;
#47998=COLOUR_RGB ( '', 0.31764706, 0.68627451, 0.89019608) ;
#48010=( LENGTH_UNIT ( ) NAMED_UNIT ( * ) SI_UNIT ( .MILLI., .METRE. ) );
#48012=DIRECTION ( 'NONE',  ( 1.000000000000000000, 0.000000000000000000, 0.000000000000000000 ) ) ;
#48015=ORIENTED_EDGE ( 'NONE', *, *, #84933, .F. ) ;
#48016=DIRECTION ( 'NONE',  ( -1.257402221000611116E-16, 1.000000000000000000, -0.000000000000000000 ) ) ;
#48040=ORIENTED_EDGE ( 'NONE', *, *, #19256, .F. ) ;
#48046=LINE ( 'NONE', #78560, #65583 ) ;
#48056=AXIS2_PLACEMENT_3D ( 'NONE', #58722, #58209, #88726 ) ;
#48057=CARTESIAN_POINT ( 'NONE',  ( -11.38910255664659310, -77.84149852289132809, 4.000000000000000000 ) ) ;
#48058=CARTESIAN_POINT ( 'NONE',  ( -3.999999999999999112, 78.07179676972445748, 6.500000000000000888 ) ) ;
#48063=LINE ( 'NONE', #71084, #50797 ) ;
#48068=FACE_OUTER_BOUND ( 'NONE', #90, .T. ) ;
#48069=AXIS2_PLACEMENT_3D ( 'NONE', #84260, #94561, #26079 ) ;
#48071=ORIENTED_EDGE ( 'NONE', *, *, #38181, .T. ) ;
#48081=SURFACE_STYLE_FILL_AREA ( #35040 ) ;
#48083=EDGE_CURVE ( 'NONE', #47721, #59353, #29570, .T. ) ;
#48094=CARTESIAN_POINT ( 'NONE',  ( -8.000000000000000000, 1.019547802438466100, 3.750000000000000000 ) ) ;
#48114=FACE_OUTER_BOUND ( 'NONE', #27822, .T. ) ;
#48117=AXIS2_PLACEMENT_3D ( 'NONE', #77935, #18922, #56429 ) ;
#48121=ORIENTED_EDGE ( 'NONE', *, *, #21004, .T. ) ;
#48124=VERTEX_POINT ( 'NONE', #45078 ) ;
#48129=CONICAL_SURFACE ( 'NONE', #5036, 1.249999999999987121, 1.029744258676652979 ) ;
#48137=DIRECTION ( 'NONE',  ( -0.000000000000000000, -0.000000000000000000, 1.000000000000000000 ) ) ;
#48142=CARTESIAN_POINT ( 'NONE',  ( -3.500000000000000444, -0.04521315095527938394, 3.750000000000000444 ) ) ;
#48143=DIRECTION ( 'NONE',  ( 0.000000000000000000, 0.000000000000000000, -1.000000000000000000 ) ) ;
#48144=DIRECTION ( 'NONE',  ( 0.000000000000000000, 0.000000000000000000, 1.000000000000000000 ) ) ;
#48148=EDGE_LOOP ( 'NONE', ( #89563, #97092, #57813, #97777 ) ) ;
#48149=CARTESIAN_POINT ( 'NONE',  ( -7.750000000000000000, 79.82179676972448590, -6.500000000000000888 ) ) ;
#48164=LINE ( 'NONE', #64999, #17270 ) ;
#48166=DIRECTION ( 'NONE',  ( 0.9961946980917462113, -0.08715574274765140739, 0.000000000000000000 ) ) ;
#48186=DIRECTION ( 'NONE',  ( 0.7808688094430307203, -0.6246950475544238435, 0.000000000000000000 ) ) ;
#48187=UNCERTAINTY_MEASURE_WITH_UNIT (LENGTH_MEASURE( 1.000000000000000082E-05 ), #24067, 'distance_accuracy_value', 'NONE');
#48209=DIRECTION ( 'NONE',  ( 0.000000000000000000, 0.000000000000000000, 1.000000000000000000 ) ) ;
#48222=CARTESIAN_POINT ( 'NONE',  ( 17.78441314508140891, 78.67289652296261693, 4.000000000000000000 ) ) ;
#48226=FACE_OUTER_BOUND ( 'NONE', #78382, .T. ) ;
#48264=SURFACE_STYLE_USAGE ( .BOTH. , #86774 ) ;
#48275=CARTESIAN_POINT ( 'NONE',  ( -8.352412229647901754, 86.23350694210130030, 4.048761466749791538 ) ) ;
#48277=ORIENTED_EDGE ( 'NONE', *, *, #97473, .F. ) ;
#48292=ADVANCED_FACE ( 'NONE', ( #8082 ), #81748, .T. ) ;
#48300=CARTESIAN_POINT ( 'NONE',  ( -18.00000000000000355, 80.99999999999994316, -3.000000000000000000 ) ) ;
#48301=CARTESIAN_POINT ( 'NONE',  ( -8.819573739049973327, 87.31373983715974418, -4.675023147224794506 ) ) ;
#48316=CARTESIAN_POINT ( 'NONE',  ( 8.742108547223832460, -4.148811688994628710, -4.000000000000000000 ) ) ;
#48318=SURFACE_SIDE_STYLE ('',( #71335 ) ) ;
#48320=CARTESIAN_POINT ( 'NONE',  ( -16.94999999999999574, 99.99999999999998579, 8.000000000000000000 ) ) ;
#48321=( NAMED_UNIT ( * ) PLANE_ANGLE_UNIT ( ) SI_UNIT ( $, .RADIAN. ) );
#48325=UNCERTAINTY_MEASURE_WITH_UNIT (LENGTH_MEASURE( 1.000000000000000082E-05 ), #60221, 'distance_accuracy_value', 'NONE');
#48333=DIRECTION ( 'NONE',  ( 0.06975647374412534407, 0.9975640502598241977, 0.000000000000000000 ) ) ;
#48337=EDGE_CURVE ( 'NONE', #18880, #70662, #38666, .T. ) ;
#48344=EDGE_LOOP ( 'NONE', ( #76052, #86991 ) ) ;
#48357=( GEOMETRIC_REPRESENTATION_CONTEXT ( 3 ) GLOBAL_UNCERTAINTY_ASSIGNED_CONTEXT ( ( #70359 ) ) GLOBAL_UNIT_ASSIGNED_CONTEXT ( ( #48522, #41046, #33508 ) ) REPRESENTATION_CONTEXT ( 'NONE', 'WORKASPACE' ) );
#48363=CYLINDRICAL_SURFACE ( 'NONE', #44595, 0.2500000000000002220 ) ;
#48367=CARTESIAN_POINT ( 'NONE',  ( -8.000000000000000000, 80.99999999999994316, 0.000000000000000000 ) ) ;
#48380=( BOUNDED_CURVE ( )  B_SPLINE_CURVE ( 3, ( #86094, #17605, #39122, #10100 ),
 .UNSPECIFIED., .F., .T. ) 
 B_SPLINE_CURVE_WITH_KNOTS ( ( 4, 4 ),
 ( 4.712388980384695891, 6.283185307179586232 ),
 .UNSPECIFIED. ) 
 CURVE ( )  GEOMETRIC_REPRESENTATION_ITEM ( )  RATIONAL_B_SPLINE_CURVE ( ( 1.000000000000000000, 0.8047378541243663808, 0.8047378541243663808, 1.000000000000000000 ) ) 
 REPRESENTATION_ITEM ( '' )  );
#48384=CARTESIAN_POINT ( 'NONE',  ( -9.208448955093622601, -19.73347625016914719, 3.750000000000001332 ) ) ;
#48387=CARTESIAN_POINT ( 'NONE',  ( 6.579634127946647482, -87.99828267815715321, 2.750000000000000000 ) ) ;
#48388=CARTESIAN_POINT ( 'NONE',  ( -7.750000000000000000, 79.82179676972448590, -6.500000000000000888 ) ) ;
#48389=CIRCLE ( 'NONE', #96309, 2.899999999999999911 ) ;
#48392=FILL_AREA_STYLE ('',( #33374 ) ) ;
#48413=CARTESIAN_POINT ( 'NONE',  ( -7.750000000000000000, 79.82179676972448590, 4.000000000000000000 ) ) ;
#48414=CARTESIAN_POINT ( 'NONE',  ( 9.512310014786894641, -15.51178930340558360, 3.750000000000001332 ) ) ;
#48417=CARTESIAN_POINT ( 'NONE',  ( 6.579634127946608402, -87.99828267815712479, -2.500000000000000000 ) ) ;
#48424=CARTESIAN_POINT ( 'NONE',  ( -5.809210876173503735, -36.07757871006351991, -2.499999999998389288 ) ) ;
#48429=DIRECTION ( 'NONE',  ( 1.697280217195517047E-15, 1.285704996138754495E-15, -1.000000000000000000 ) ) ;
#48434=CARTESIAN_POINT ( 'NONE',  ( -13.77612262535527954, 90.93158326518027934, -7.883772450803742338 ) ) ;
#48436=CYLINDRICAL_SURFACE ( 'NONE', #63910, 0.2500000000000002220 ) ;
#48448=UNCERTAINTY_MEASURE_WITH_UNIT (LENGTH_MEASURE( 1.000000000000000082E-05 ), #23599, 'distance_accuracy_value', 'NONE');
#48456=ORIENTED_EDGE ( 'NONE', *, *, #27032, .F. ) ;
#48457=DIRECTION ( 'NONE',  ( -0.9975640502598257520, 0.06975647374410356982, 0.000000000000000000 ) ) ;
#48467=AXIS2_PLACEMENT_3D ( 'NONE', #8230, #46226, #83730 ) ;
#48471=VERTEX_POINT ( 'NONE', #70061 ) ;
#48475=LINE ( 'NONE', #10484, #47636 ) ;
#48480=CARTESIAN_POINT ( 'NONE',  ( -8.332123631136926889, -7.291398214258985711, -3.750000000000000888 ) ) ;
#48485=ADVANCED_FACE ( 'NONE', ( #62536 ), #33845, .T. ) ;
#48492=EDGE_CURVE ( 'NONE', #37577, #63243, #24576, .T. ) ;
#48500=ORIENTED_EDGE ( 'NONE', *, *, #27363, .F. ) ;
#48514=CARTESIAN_POINT ( 'NONE',  ( 6.579634127946657252, -87.99828267815705374, -2.750000000000000000 ) ) ;
#48522=( LENGTH_UNIT ( ) NAMED_UNIT ( * ) SI_UNIT ( .MILLI., .METRE. ) );
#48523=EDGE_LOOP ( 'NONE', ( #39762, #5081, #5346, #82052 ) ) ;
#48528=CARTESIAN_POINT ( 'NONE',  ( -8.000000000000000000, 80.99999999999994316, 3.000000000000000000 ) ) ;
#48537=EDGE_CURVE ( 'NONE', #19902, #37612, #98490, .T. ) ;
#48545=CARTESIAN_POINT ( 'NONE',  ( 11.49999999999999645, 75.00000000000000000, -8.525133428036872019 ) ) ;
#48552=CARTESIAN_POINT ( 'NONE',  ( -10.91022435255008283, -52.91485255063000182, 4.000000000000000000 ) ) ;
#48557=FILL_AREA_STYLE ('',( #63559 ) ) ;
#48559=CIRCLE ( 'NONE', #96479, 2.000000000000000888 ) ;
#48565=ORIENTED_EDGE ( 'NONE', *, *, #17312, .F. ) ;
#48567=EDGE_CURVE ( 'NONE', #30525, #40405, #27583, .T. ) ;
#48580=DIRECTION ( 'NONE',  ( 0.000000000000000000, 1.000000000000000000, 0.000000000000000000 ) ) ;
#48582=ORIENTED_EDGE ( 'NONE', *, *, #57475, .T. ) ;
#48583=ORIENTED_EDGE ( 'NONE', *, *, #57903, .F. ) ;
#48587=DIRECTION ( 'NONE',  ( -0.000000000000000000, -0.000000000000000000, 1.000000000000000000 ) ) ;
#48606=( NAMED_UNIT ( * ) PLANE_ANGLE_UNIT ( ) SI_UNIT ( $, .RADIAN. ) );
#48611=EDGE_LOOP ( 'NONE', ( #2559, #27189, #78969, #95005 ) ) ;
#48613=ORIENTED_EDGE ( 'NONE', *, *, #70780, .F. ) ;
#48620=CARTESIAN_POINT ( 'NONE',  ( -8.000000000000000000, 41.24999999999999289, 4.000000000000000000 ) ) ;
#48622=STYLED_ITEM ( 'NONE', ( #87864 ), #95471 ) ;
#48624=CARTESIAN_POINT ( 'NONE',  ( -3.770608837557422710, -6.399801140515898545, 2.750000000000403677 ) ) ;
#48626=CARTESIAN_POINT ( 'NONE',  ( 11.33984840998195054, -87.82327540140187239, 3.750000000000000000 ) ) ;
#48631=ADVANCED_FACE ( 'NONE', ( #56046 ), #96513, .T. ) ;
#48632=CARTESIAN_POINT ( 'NONE',  ( -6.445967608602039434, -48.01283281809150338, 2.750000000000000000 ) ) ;
#48651=VERTEX_POINT ( 'NONE', #21991 ) ;
#48653=CARTESIAN_POINT ( 'NONE',  ( -18.89999999999999503, 92.00000000000000000, 8.000000000000000000 ) ) ;
#48666=( GEOMETRIC_REPRESENTATION_CONTEXT ( 3 ) GLOBAL_UNCERTAINTY_ASSIGNED_CONTEXT ( ( #74264 ) ) GLOBAL_UNIT_ASSIGNED_CONTEXT ( ( #4608, #48606, #34087 ) ) REPRESENTATION_CONTEXT ( 'NONE', 'WORKASPACE' ) );
#48687=CARTESIAN_POINT ( 'NONE',  ( 4.380000000000000782, 1.019547802438464545, 3.750000000000001776 ) ) ;
#48693=CARTESIAN_POINT ( 'NONE',  ( 4.219999999999999751, 36.75000000000000000, 2.750000000000000000 ) ) ;
#48710=( GEOMETRIC_REPRESENTATION_CONTEXT ( 3 ) GLOBAL_UNCERTAINTY_ASSIGNED_CONTEXT ( ( #51475 ) ) GLOBAL_UNIT_ASSIGNED_CONTEXT ( ( #67841, #14345, #13847 ) ) REPRESENTATION_CONTEXT ( 'NONE', 'WORKASPACE' ) );
#48716=CARTESIAN_POINT ( 'NONE',  ( -7.121448108906508700, -73.25984652122873797, 3.750000000000000888 ) ) ;
#48719=ORIENTED_EDGE ( 'NONE', *, *, #7294, .T. ) ;
#48721=ORIENTED_EDGE ( 'NONE', *, *, #14032, .F. ) ;
#48729=ORIENTED_EDGE ( 'NONE', *, *, #80448, .T. ) ;
#48767=CARTESIAN_POINT ( 'NONE',  ( -9.884188733557275341, 88.99910865660901038, 5.687374854485731213 ) ) ;
#48770=EDGE_CURVE ( 'NONE', #11363, #41505, #5008, .T. ) ;
#48775=SURFACE_STYLE_FILL_AREA ( #16818 ) ;
#48786=CARTESIAN_POINT ( 'NONE',  ( -7.121364477235284873, -73.24716134357460362, 2.750000000000000444 ) ) ;
#48787=ORIENTED_EDGE ( 'NONE', *, *, #6341, .F. ) ;
#48788=MECHANICAL_DESIGN_GEOMETRIC_PRESENTATION_REPRESENTATION('',(#10482),#37687);
#48792=CARTESIAN_POINT ( 'NONE',  ( -8.000343251535923628, 84.06932101904432386, -4.000000000000000000 ) ) ;
#48800=ADVANCED_FACE ( 'NONE', ( #28489 ), #58982, .F. ) ;
#48809=FACE_OUTER_BOUND ( 'NONE', #85138, .T. ) ;
#48811=DIRECTION ( 'NONE',  ( 0.8070303256584299145, -0.5905099943842175847, 0.000000000000000000 ) ) ;
#48836=ORIENTED_EDGE ( 'NONE', *, *, #77434, .F. ) ;
#48837=CIRCLE ( 'NONE', #23316, 0.2500000000000002220 ) ;
#48841=LINE ( 'NONE', #63833, #26925 ) ;
#48845=AXIS2_PLACEMENT_3D ( 'NONE', #58406, #65913, #36415 ) ;
#48860=EDGE_CURVE ( 'NONE', #79829, #14094, #80256, .T. ) ;
#48863=ORIENTED_EDGE ( 'NONE', *, *, #21031, .F. ) ;
#48870=CARTESIAN_POINT ( 'NONE',  ( -8.108506836784059146, -3.139057133285344303, 3.750000000000000888 ) ) ;
#48872=DIRECTION ( 'NONE',  ( 1.000000000000000000, 0.000000000000000000, 0.000000000000000000 ) ) ;
#48874=AXIS2_PLACEMENT_3D ( 'NONE', #61676, #31675, #40176 ) ;
#48881=DIRECTION ( 'NONE',  ( -2.569960705150826877E-16, 1.000000000000000000, 0.000000000000000000 ) ) ;
#48882=EDGE_CURVE ( 'NONE', #21081, #12912, #72257, .T. ) ;
#48888=ADVANCED_FACE ( 'NONE', ( #12984 ), #51379, .T. ) ;
#48890=LINE ( 'NONE', #28362, #20083 ) ;
#48899=PLANE ( 'NONE',  #86765 ) ;
#48912=( GEOMETRIC_REPRESENTATION_CONTEXT ( 3 ) GLOBAL_UNCERTAINTY_ASSIGNED_CONTEXT ( ( #94510 ) ) GLOBAL_UNIT_ASSIGNED_CONTEXT ( ( #13087, #49596, #80105 ) ) REPRESENTATION_CONTEXT ( 'NONE', 'WORKASPACE' ) );
#48914=CARTESIAN_POINT ( 'NONE',  ( -6.867320125558078914, -58.36821204062274404, -2.750000000000000000 ) ) ;
#48918=DIRECTION ( 'NONE',  ( 0.000000000000000000, 0.000000000000000000, 1.000000000000000000 ) ) ;
#48945=DIRECTION ( 'NONE',  ( -1.000000000000000000, -0.000000000000000000, -0.000000000000000000 ) ) ;
#48994=CARTESIAN_POINT ( 'NONE',  ( -3.271887613349916180, -0.8417457659429956607, 2.500000000000000888 ) ) ;
#48995=CARTESIAN_POINT ( 'NONE',  ( 8.879999999999991900, 27.04366094290857347, 2.900000000000000355 ) ) ;
#49007=( GEOMETRIC_REPRESENTATION_CONTEXT ( 3 ) GLOBAL_UNCERTAINTY_ASSIGNED_CONTEXT ( ( #71465 ) ) GLOBAL_UNIT_ASSIGNED_CONTEXT ( ( #89494, #14498, #44969 ) ) REPRESENTATION_CONTEXT ( 'NONE', 'WORKASPACE' ) );
#49008=EDGE_CURVE ( 'NONE', #84748, #59823, #92920, .T. ) ;
#49027=DIRECTION ( 'NONE',  ( -0.000000000000000000, -1.000000000000000000, -4.683753385137374737E-14 ) ) ;
#49032=STYLED_ITEM ( 'NONE', ( #70958 ), #40953 ) ;
#49059=FACE_OUTER_BOUND ( 'NONE', #53771, .T. ) ;
#49067=( NAMED_UNIT ( * ) PLANE_ANGLE_UNIT ( ) SI_UNIT ( $, .RADIAN. ) );
#49081=AXIS2_PLACEMENT_3D ( 'NONE', #63865, #64847, #70417 ) ;
#49083=DIRECTION ( 'NONE',  ( 0.06975647374412544122, 0.9975640502598241977, -0.000000000000000000 ) ) ;
#49089=DIRECTION ( 'NONE',  ( -0.000000000000000000, 0.000000000000000000, -1.000000000000000000 ) ) ;
#49090=CARTESIAN_POINT ( 'NONE',  ( -8.000000000000000000, 1.019547802438466100, 4.000000000000000000 ) ) ;
#49110=CIRCLE ( 'NONE', #61879, 0.5000000000000004441 ) ;
#49119=CARTESIAN_POINT ( 'NONE',  ( -10.09048698379360687, 46.92328126389585208, 0.000000000000000000 ) ) ;
#49126=CARTESIAN_POINT ( 'NONE',  ( 11.01504402823088213, -96.09667835297135241, 4.000000000000000000 ) ) ;
#49133=LINE ( 'NONE', #11623, #58769 ) ;
#49134=FILL_AREA_STYLE_COLOUR ( '', #83347 ) ;
#49138=DIRECTION ( 'NONE',  ( -1.000000000000000000, 0.000000000000000000, 0.000000000000000000 ) ) ;
#49140=AXIS2_PLACEMENT_3D ( 'NONE', #50882, #51372, #5877 ) ;
#49141=FILL_AREA_STYLE_COLOUR ( '', #80250 ) ;
#49145=SURFACE_SIDE_STYLE ('',( #79646 ) ) ;
#49148=CARTESIAN_POINT ( 'NONE',  ( 0.4400000000000020006, 1.019547802438468986, 2.750000000000000000 ) ) ;
#49157=FACE_OUTER_BOUND ( 'NONE', #78924, .T. ) ;
#49162=CARTESIAN_POINT ( 'NONE',  ( -11.37644997975658612, -81.99697149686846842, -4.000000000000000000 ) ) ;
#49181=VERTEX_POINT ( 'NONE', #55425 ) ;
#49182=CARTESIAN_POINT ( 'NONE',  ( -7.750000000000000000, 41.24999999999999289, 6.250000000000000000 ) ) ;
#49194=EDGE_LOOP ( 'NONE', ( #49228, #33881, #88814, #87263 ) ) ;
#49213=ORIENTED_EDGE ( 'NONE', *, *, #11408, .F. ) ;
#49215=ORIENTED_EDGE ( 'NONE', *, *, #14952, .T. ) ;
#49221=EDGE_CURVE ( 'NONE', #15093, #95449, #93034, .T. ) ;
#49228=ORIENTED_EDGE ( 'NONE', *, *, #76771, .T. ) ;
#49230=VERTEX_POINT ( 'NONE', #18413 ) ;
#49244=CARTESIAN_POINT ( 'NONE',  ( -8.000000000000000000, 40.74999999999999289, -4.250000000000000000 ) ) ;
#49248=SURFACE_SIDE_STYLE ('',( #43215 ) ) ;
#49257=CARTESIAN_POINT ( 'NONE',  ( -4.000000000000000000, 78.07179676972445748, -6.250000000000000000 ) ) ;
#49263=AXIS2_PLACEMENT_3D ( 'NONE', #44904, #44415, #74919 ) ;
#49279=DIRECTION ( 'NONE',  ( -1.000000000000000000, 0.000000000000000000, 0.000000000000000000 ) ) ;
#49283=CARTESIAN_POINT ( 'NONE',  ( -3.627897631252527511, -3.626520420884125517, 2.750000000000000000 ) ) ;
#49287=SURFACE_SIDE_STYLE ('',( #71318 ) ) ;
#49301=SURFACE_STYLE_FILL_AREA ( #95294 ) ;
#49339=EDGE_CURVE ( 'NONE', #93548, #70269, #62920, .T. ) ;
#49346=DIRECTION ( 'NONE',  ( -0.000000000000000000, 0.000000000000000000, 1.000000000000000000 ) ) ;
#49354=AXIS2_PLACEMENT_3D ( 'NONE', #34079, #64571, #81555 ) ;
#49369=DIRECTION ( 'NONE',  ( 1.000000000000000000, 0.000000000000000000, -6.938893903907221278E-15 ) ) ;
#49373=CARTESIAN_POINT ( 'NONE',  ( -8.000000000000000000, 40.74999999999999289, 4.250000000000000000 ) ) ;
#49379=LINE ( 'NONE', #62908, #74384 ) ;
#49389=AXIS2_PLACEMENT_3D ( 'NONE', #52952, #16448, #76451 ) ;
#49393=DIRECTION ( 'NONE',  ( 1.000000000000000000, 0.000000000000000000, 0.000000000000000000 ) ) ;
#49399=ORIENTED_EDGE ( 'NONE', *, *, #87589, .F. ) ;
#49402=CARTESIAN_POINT ( 'NONE',  ( -4.285674571758069540, -17.54407107684652445, -2.500000000000000000 ) ) ;
#49408=VERTEX_POINT ( 'NONE', #49879 ) ;
#49409=CARTESIAN_POINT ( 'NONE',  ( 4.573751236499521866, -6.413519960490759786, -4.000000000000000000 ) ) ;
#49431=DIRECTION ( 'NONE',  ( 0.000000000000000000, -1.000000000000000000, 0.000000000000000000 ) ) ;
#49432=CARTESIAN_POINT ( 'NONE',  ( 8.629999999999995453, 40.74999999999999289, 4.250000000000000000 ) ) ;
#49440=ORIENTED_EDGE ( 'NONE', *, *, #73827, .T. ) ;
#49450=DIRECTION ( 'NONE',  ( 1.000000000000000000, 0.000000000000000000, 0.000000000000000000 ) ) ;
#49457=CARTESIAN_POINT ( 'NONE',  ( -11.26206397713064256, -93.45673894084376343, -3.749999999999999556 ) ) ;
#49479=CARTESIAN_POINT ( 'NONE',  ( -6.617298650316659980, -58.37178459782695228, 2.500000000000000000 ) ) ;
#49491=VERTEX_POINT ( 'NONE', #58353 ) ;
#49492=ORIENTED_EDGE ( 'NONE', *, *, #58216, .F. ) ;
#49495=UNCERTAINTY_MEASURE_WITH_UNIT (LENGTH_MEASURE( 1.000000000000000082E-05 ), #75690, 'distance_accuracy_value', 'NONE');
#49502=EDGE_LOOP ( 'NONE', ( #92888, #1060, #9661, #22178 ) ) ;
#49521=CARTESIAN_POINT ( 'NONE',  ( -8.646548597236174416, 87.41340560412834293, 4.720830526302458807 ) ) ;
#49523=CARTESIAN_POINT ( 'NONE',  ( 0.000000000000000000, 99.74999999999998579, -7.750000000000000000 ) ) ;
#49524=VECTOR ( 'NONE', #74224, 1000.000000000000000 ) ;
#49535=CARTESIAN_POINT ( 'NONE',  ( 18.00000000000000000, 78.09931407715666296, -3.985200473436270485 ) ) ;
#49541=( NAMED_UNIT ( * ) SI_UNIT ( $, .STERADIAN. ) SOLID_ANGLE_UNIT ( ) );
#49551=DIRECTION ( 'NONE',  ( -6.938893903907222067E-15, 0.000000000000000000, 1.000000000000000000 ) ) ;
#49553=CARTESIAN_POINT ( 'NONE',  ( -3.750000001621983436, 0.08803144853716619866, -4.000000000000000000 ) ) ;
#49555=ORIENTED_EDGE ( 'NONE', *, *, #22702, .F. ) ;
#49569=STYLED_ITEM ( 'NONE', ( #44383 ), #45605 ) ;
#49581=FACE_OUTER_BOUND ( 'NONE', #98866, .T. ) ;
#49591=DIRECTION ( 'NONE',  ( -0.06975647374412567714, -0.9975640502598243087, 0.000000000000000000 ) ) ;
#49596=( NAMED_UNIT ( * ) PLANE_ANGLE_UNIT ( ) SI_UNIT ( $, .RADIAN. ) );
#49600=CARTESIAN_POINT ( 'NONE',  ( 11.33984840991517373, -87.82327540140084920, 4.000000000000000000 ) ) ;
#49602=CARTESIAN_POINT ( 'NONE',  ( -9.000000000000003553, 80.99999999999994316, -1.249999999999987121 ) ) ;
#49604=CARTESIAN_POINT ( 'NONE',  ( -6.841090228438033272, -58.65898919720570603, 2.750000000000000000 ) ) ;
#49605=ORIENTED_EDGE ( 'NONE', *, *, #84272, .T. ) ;
#49607=CARTESIAN_POINT ( 'NONE',  ( -7.750000000000000000, 40.99999999999999289, -6.250000000000000000 ) ) ;
#49612=CARTESIAN_POINT ( 'NONE',  ( 14.35000000000000142, 98.49999999999998579, -8.525133428036873795 ) ) ;
#49614=PRESENTATION_STYLE_ASSIGNMENT (( #94144 ) ) ;
#49620=DIRECTION ( 'NONE',  ( 0.000000000000000000, -1.000000000000000000, 0.000000000000000000 ) ) ;
#49622=ORIENTED_EDGE ( 'NONE', *, *, #5326, .F. ) ;
#49627=VECTOR ( 'NONE', #78582, 999.9999999999998863 ) ;
#49633=DIRECTION ( 'NONE',  ( -1.000000000000000000, 0.000000000000000000, 0.000000000000000000 ) ) ;
#49656=VERTEX_POINT ( 'NONE', #26289 ) ;
#49669=VECTOR ( 'NONE', #69831, 1000.000000000000000 ) ;
#49671=CARTESIAN_POINT ( 'NONE',  ( -18.89999999999999503, 92.00000000000000000, -7.750000000000000000 ) ) ;
#49695=VERTEX_POINT ( 'NONE', #2347 ) ;
#49712=VECTOR ( 'NONE', #32594, 1000.000000000000000 ) ;
#49719=SURFACE_STYLE_FILL_AREA ( #20222 ) ;
#49725=( LENGTH_UNIT ( ) NAMED_UNIT ( * ) SI_UNIT ( .MILLI., .METRE. ) );
#49734=FACE_OUTER_BOUND ( 'NONE', #44792, .T. ) ;
#49744=CARTESIAN_POINT ( 'NONE',  ( 18.00000000000000355, 77.07179676972445748, -6.500000000000000888 ) ) ;
#49756=DIRECTION ( 'NONE',  ( -0.000000000000000000, -0.000000000000000000, 1.000000000000000000 ) ) ;
#49760=FILL_AREA_STYLE ('',( #12261 ) ) ;
#49761=PRESENTATION_STYLE_ASSIGNMENT (( #72753 ) ) ;
#49768=DIRECTION ( 'NONE',  ( -0.000000000000000000, -0.000000000000000000, 1.000000000000000000 ) ) ;
#49774=CARTESIAN_POINT ( 'NONE',  ( -9.884188733557275341, 88.99910865660910986, -5.687374854485797826 ) ) ;
#49778=AXIS2_PLACEMENT_3D ( 'NONE', #54267, #75300, #46772 ) ;
#49783=PLANE ( 'NONE',  #87580 ) ;
#49789=CARTESIAN_POINT ( 'NONE',  ( 8.705944879818165560, -3.115743166029874889, -4.000000000000000888 ) ) ;
#49791=SURFACE_STYLE_FILL_AREA ( #13276 ) ;
#49798=EDGE_CURVE ( 'NONE', #78252, #49181, #36766, .T. ) ;
#49810=ADVANCED_FACE ( 'NONE', ( #27270 ), #51762, .T. ) ;
#49816=ORIENTED_EDGE ( 'NONE', *, *, #69112, .F. ) ;
#49819=ORIENTED_EDGE ( 'NONE', *, *, #35698, .T. ) ;
#49831=VERTEX_POINT ( 'NONE', #29248 ) ;
#49842=VECTOR ( 'NONE', #18760, 1000.000000000000000 ) ;
#49852=VECTOR ( 'NONE', #59542, 999.9999999999998863 ) ;
#49858=FACE_OUTER_BOUND ( 'NONE', #97906, .T. ) ;
#49870=EDGE_LOOP ( 'NONE', ( #56697, #87223, #37952, #23722 ) ) ;
#49879=CARTESIAN_POINT ( 'NONE',  ( 6.829574850505126804, -88.00372650098204019, 2.750000000000002665 ) ) ;
#49885=FILL_AREA_STYLE_COLOUR ( '', #75234 ) ;
#49891=VECTOR ( 'NONE', #84426, 1000.000000000000000 ) ;
#49894=ADVANCED_FACE ( 'NONE', ( #5775 ), #65260, .T. ) ;
#49895=EDGE_CURVE ( 'NONE', #20729, #16419, #77508, .T. ) ;
#49897=CARTESIAN_POINT ( 'NONE',  ( -3.500000000000000444, 1.019547802438453887, -2.499999999999999556 ) ) ;
#49898=CARTESIAN_POINT ( 'NONE',  ( -8.099999999999999645, 80.99999999999994316, 3.000000000000000000 ) ) ;
#49905=CARTESIAN_POINT ( 'NONE',  ( 6.575338752131433040, -50.90849809618014632, -3.750000000000000000 ) ) ;
#49909=CARTESIAN_POINT ( 'NONE',  ( -6.281451360760613944, -39.80862496263594608, 4.000000000000000000 ) ) ;
#49911=DIRECTION ( 'NONE',  ( 0.000000000000000000, -1.000000000000000000, 0.000000000000000000 ) ) ;
#49928=AXIS2_PLACEMENT_3D ( 'NONE', #28967, #73982, #96010 ) ;
#49929=ORIENTED_EDGE ( 'NONE', *, *, #10623, .T. ) ;
#49935=ADVANCED_FACE ( 'NONE', ( #42783 ), #16865, .F. ) ;
#49941=AXIS2_PLACEMENT_3D ( 'NONE', #50072, #95579, #27066 ) ;
#49951=CARTESIAN_POINT ( 'NONE',  ( 8.879999999999991900, 18.00000000000000355, 3.000000000000000000 ) ) ;
#49957=CARTESIAN_POINT ( 'NONE',  ( -11.58474105865894010, -69.55891867961692299, -3.750000000000000444 ) ) ;
#49989=( GEOMETRIC_REPRESENTATION_CONTEXT ( 3 ) GLOBAL_UNCERTAINTY_ASSIGNED_CONTEXT ( ( #45263 ) ) GLOBAL_UNIT_ASSIGNED_CONTEXT ( ( #11799, #88784, #65277 ) ) REPRESENTATION_CONTEXT ( 'NONE', 'WORKASPACE' ) );
#49990=ORIENTED_EDGE ( 'NONE', *, *, #52742, .F. ) ;
#49993=ORIENTED_EDGE ( 'NONE', *, *, #61875, .T. ) ;
#49995=DIRECTION ( 'NONE',  ( 0.000000000000000000, 0.000000000000000000, 1.000000000000000000 ) ) ;
#50000=MECHANICAL_DESIGN_GEOMETRIC_PRESENTATION_REPRESENTATION('',(#6909),#5344);
#50008=VECTOR ( 'NONE', #42859, 1000.000000000000114 ) ;
#50009=ADVANCED_FACE ( 'NONE', ( #38251 ), #23256, .F. ) ;
#50019=EDGE_CURVE ( 'NONE', #71601, #70379, #83879, .T. ) ;
#50022=DIRECTION ( 'NONE',  ( -0.000000000000000000, -1.000000000000000000, 0.000000000000000000 ) ) ;
#50023=EDGE_CURVE ( 'NONE', #93536, #93548, #67759, .T. ) ;
#50038=AXIS2_PLACEMENT_3D ( 'NONE', #68941, #61909, #92903 ) ;
#50040=CARTESIAN_POINT ( 'NONE',  ( 17.87804611792018150, 78.26090218833560641, -4.039389165979423879 ) ) ;
#50046=CARTESIAN_POINT ( 'NONE',  ( -3.627897627657490798, -3.626520239197509987, -3.750000000000000444 ) ) ;
#50047=FILL_AREA_STYLE_COLOUR ( '', #75278 ) ;
#50053=EDGE_CURVE ( 'NONE', #69049, #59353, #10434, .T. ) ;
#50062=FACE_OUTER_BOUND ( 'NONE', #6536, .T. ) ;
#50065=ORIENTED_EDGE ( 'NONE', *, *, #73587, .T. ) ;
#50070=CARTESIAN_POINT ( 'NONE',  ( -13.68576102233676295, 90.96604444080064411, 7.941738159297530686 ) ) ;
#50072=CARTESIAN_POINT ( 'NONE',  ( -3.250000000000000444, 1.019547802438465656, -2.750000000000000000 ) ) ;
#50074=VECTOR ( 'NONE', #5613, 1000.000000000000000 ) ;
#50077=VECTOR ( 'NONE', #2503, 1000.000000000000000 ) ;
#50080=CARTESIAN_POINT ( 'NONE',  ( 3.969999999999999751, 10.00000000000000000, 2.500000000000000000 ) ) ;
#50100=DIRECTION ( 'NONE',  ( -1.000000000000000000, 0.000000000000000000, 0.000000000000000000 ) ) ;
#50109=CARTESIAN_POINT ( 'NONE',  ( -7.127794346849581686, -80.93619716733995517, 2.750000000000000000 ) ) ;
#50121=DIRECTION ( 'NONE',  ( 0.000000000000000000, 0.000000000000000000, -1.000000000000000000 ) ) ;
#50128=EDGE_CURVE ( 'NONE', #43266, #13075, #45549, .T. ) ;
#50135=CARTESIAN_POINT ( 'NONE',  ( -8.000000000000000000, 80.99999999999994316, 1.249999999999987121 ) ) ;
#50142=CARTESIAN_POINT ( 'NONE',  ( -10.53011945866295029, -98.59345040283277228, -3.999999999999994671 ) ) ;
#50153=DIRECTION ( 'NONE',  ( 0.000000000000000000, -1.000000000000000000, 0.000000000000000000 ) ) ;
#50160=CARTESIAN_POINT ( 'NONE',  ( 6.533420211785746723, -50.31490269211863620, 3.750000000000001776 ) ) ;
#50166=LINE ( 'NONE', #80675, #8052 ) ;
#50168=VERTEX_POINT ( 'NONE', #84728 ) ;
#50179=CARTESIAN_POINT ( 'NONE',  ( -10.85644721913293154, -98.10785618599911118, 3.750000000000000000 ) ) ;
#50189=CARTESIAN_POINT ( 'NONE',  ( 0.000000000000000000, -97.00000000000000000, 4.000000000000000000 ) ) ;
#50191=ORIENTED_EDGE ( 'NONE', *, *, #44949, .T. ) ;
#50197=AXIS2_PLACEMENT_3D ( 'NONE', #62905, #3401, #71413 ) ;
#50212=EDGE_CURVE ( 'NONE', #25656, #35357, #4091, .T. ) ;
#50215=DIRECTION ( 'NONE',  ( 0.000000000000000000, 1.000000000000000000, 0.000000000000000000 ) ) ;
#50221=LINE ( 'NONE', #42739, #64954 ) ;
#50229=COLOUR_RGB ( '', 0.66274510, 0.83137255, 0.94901961) ;
#50238=ORIENTED_EDGE ( 'NONE', *, *, #59192, .F. ) ;
#50250=CARTESIAN_POINT ( 'NONE',  ( 4.380000000000002558, 1.019547802438462547, 3.750000000000000000 ) ) ;
#50260=CARTESIAN_POINT ( 'NONE',  ( -10.94840535726567943, 89.72140148746872512, -6.176821657850955383 ) ) ;
#50268=FACE_BOUND ( 'NONE', #24763, .T. ) ;
#50276=CARTESIAN_POINT ( 'NONE',  ( 10.76917535773492141, -96.07946373138615570, -4.000000000000000000 ) ) ;
#50280=SURFACE_STYLE_FILL_AREA ( #95807 ) ;
#50285=UNCERTAINTY_MEASURE_WITH_UNIT (LENGTH_MEASURE( 1.000000000000000082E-05 ), #76156, 'distance_accuracy_value', 'NONE');
#50286=VERTEX_POINT ( 'NONE', #15264 ) ;
#50301=CARTESIAN_POINT ( 'NONE',  ( 0.000000000000000000, -97.00000000000000000, -3.750000000000000000 ) ) ;
#50308=CYLINDRICAL_SURFACE ( 'NONE', #13812, 0.2500000000000002220 ) ;
#50322=AXIS2_PLACEMENT_3D ( 'NONE', #1320, #15812, #39788 ) ;
#50330=ADVANCED_FACE ( 'NONE', ( #87167 ), #62200, .F. ) ;
#50344=CARTESIAN_POINT ( 'NONE',  ( -13.78092363094822304, 90.91979277574868945, -7.864123332961985291 ) ) ;
#50356=DIRECTION ( 'NONE',  ( 1.000000000000000000, 0.000000000000000000, 0.000000000000000000 ) ) ;
#50359=EDGE_CURVE ( 'NONE', #39257, #63305, #11175, .T. ) ;
#50387=CARTESIAN_POINT ( 'NONE',  ( -6.866255446112624838, -80.67934795256483937, -2.500000000000000000 ) ) ;
#50398=CARTESIAN_POINT ( 'NONE',  ( -7.287667432647796595, -86.26780665046146623, 4.000000000000000000 ) ) ;
#50400=DIRECTION ( 'NONE',  ( 0.000000000000000000, 0.000000000000000000, -1.000000000000000000 ) ) ;
#50408=PRESENTATION_STYLE_ASSIGNMENT (( #19917 ) ) ;
#50411=AXIS2_PLACEMENT_3D ( 'NONE', #4400, #34868, #27371 ) ;
#50420=CARTESIAN_POINT ( 'NONE',  ( 14.99999999999997691, 80.32179676972448590, -4.000000000000000000 ) ) ;
#50428=ORIENTED_EDGE ( 'NONE', *, *, #55560, .F. ) ;
#50433=CARTESIAN_POINT ( 'NONE',  ( -4.250000000000000000, 10.25000000000000000, -4.000000000000000000 ) ) ;
#50438=LINE ( 'NONE', #35929, #22854 ) ;
#50439=CARTESIAN_POINT ( 'NONE',  ( -5.149999999999996803, 98.49999999999998579, -8.525133428036873795 ) ) ;
#50488=VECTOR ( 'NONE', #59689, 1000.000000000000000 ) ;
#50490=UNCERTAINTY_MEASURE_WITH_UNIT (LENGTH_MEASURE( 1.000000000000000082E-05 ), #65354, 'distance_accuracy_value', 'NONE');
#50492=EDGE_CURVE ( 'NONE', #59916, #37810, #33664, .T. ) ;
#50533=CARTESIAN_POINT ( 'NONE',  ( 18.00000000000000000, 77.35022402049111179, -4.131279366365265382 ) ) ;
#50536=MECHANICAL_DESIGN_GEOMETRIC_PRESENTATION_REPRESENTATION('',(#45776),#47315);
#50540=DIRECTION ( 'NONE',  ( 0.000000000000000000, 0.000000000000000000, -1.000000000000000000 ) ) ;
#50554=COLOUR_RGB ( '', 0.08235294, 0.09019608, 0.10196078) ;
#50555=CARTESIAN_POINT ( 'NONE',  ( 11.20711848508407016, -56.83082008004717522, -3.750000000000000000 ) ) ;
#50556=CARTESIAN_POINT ( 'NONE',  ( -4.021995598253403692, -6.415937870592102854, -4.000000000000000000 ) ) ;
#50557=MECHANICAL_DESIGN_GEOMETRIC_PRESENTATION_REPRESENTATION('',(#37808),#45711);
#50564=CARTESIAN_POINT ( 'NONE',  ( -7.750000000000000000, 83.99999999999994316, 4.000000000000000000 ) ) ;
#50567=AXIS2_PLACEMENT_3D ( 'NONE', #9657, #32637, #18148 ) ;
#50575=( NAMED_UNIT ( * ) PLANE_ANGLE_UNIT ( ) SI_UNIT ( $, .RADIAN. ) );
#50594=ORIENTED_EDGE ( 'NONE', *, *, #53716, .F. ) ;
#50600=LINE ( 'NONE', #88588, #26721 ) ;
#50601=DIRECTION ( 'NONE',  ( -1.000000000000000000, 0.000000000000000000, 0.000000000000000000 ) ) ;
#50604=ORIENTED_EDGE ( 'NONE', *, *, #85750, .F. ) ;
#50625=FACE_OUTER_BOUND ( 'NONE', #55214, .T. ) ;
#50633=CARTESIAN_POINT ( 'NONE',  ( -5.112373461513591621, -25.53775085953292390, -3.750000000000000000 ) ) ;
#50635=DIRECTION ( 'NONE',  ( 1.000000000000000000, 0.000000000000000000, -0.000000000000000000 ) ) ;
#50643=CARTESIAN_POINT ( 'NONE',  ( -11.62646502397220871, -81.99905065409890881, -4.000000000003602452 ) ) ;
#50648=AXIS2_PLACEMENT_3D ( 'NONE', #27846, #73346, #23208 ) ;
#50650=AXIS2_PLACEMENT_3D ( 'NONE', #60016, #20556, #13041 ) ;
#50671=PLANE ( 'NONE',  #82506 ) ;
#50674=DIRECTION ( 'NONE',  ( 1.000000000000000000, -0.000000000000000000, -0.000000000000000000 ) ) ;
#50685=CARTESIAN_POINT ( 'NONE',  ( -10.95094547707107502, -94.44763431416964750, 4.000000000000000000 ) ) ;
#50697=EDGE_LOOP ( 'NONE', ( #10712, #37168, #76986, #82289 ) ) ;
#50709=EDGE_LOOP ( 'NONE', ( #93979, #20281, #22374, #63506, #66564 ) ) ;
#50713=ORIENTED_EDGE ( 'NONE', *, *, #19665, .F. ) ;
#50715=CIRCLE ( 'NONE', #45936, 0.2500000000000002220 ) ;
#50722=MECHANICAL_DESIGN_GEOMETRIC_PRESENTATION_REPRESENTATION('',(#71513),#34793);
#50727=EDGE_CURVE ( 'NONE', #20156, #47721, #43957, .T. ) ;
#50757=LINE ( 'NONE', #26764, #21714 ) ;
#50770=ORIENTED_EDGE ( 'NONE', *, *, #16284, .T. ) ;
#50773=CARTESIAN_POINT ( 'NONE',  ( -13.83909701985791152, 90.94176541299273708, -7.900788997805661573 ) ) ;
#50797=VECTOR ( 'NONE', #2609, 1000.000000000000114 ) ;
#50799=ORIENTED_EDGE ( 'NONE', *, *, #94629, .F. ) ;
#50821=ORIENTED_EDGE ( 'NONE', *, *, #84582, .F. ) ;
#50822=FACE_OUTER_BOUND ( 'NONE', #84765, .T. ) ;
#50825=DIRECTION ( 'NONE',  ( -1.000000000000000000, -0.000000000000000000, -0.000000000000000000 ) ) ;
#50830=ORIENTED_EDGE ( 'NONE', *, *, #43941, .F. ) ;
#50832=EDGE_LOOP ( 'NONE', ( #44286, #71241, #13563, #81684, #97679 ) ) ;
#50843=DIRECTION ( 'NONE',  ( -0.000000000000000000, 1.000000000000000000, 0.000000000000000000 ) ) ;
#50847=ORIENTED_EDGE ( 'NONE', *, *, #17533, .F. ) ;
#50848=AXIS2_PLACEMENT_3D ( 'NONE', #25435, #40921, #40430 ) ;
#50851=LINE ( 'NONE', #42371, #50008 ) ;
#50855=FACE_OUTER_BOUND ( 'NONE', #54976, .T. ) ;
#50856=ADVANCED_FACE ( 'NONE', ( #80160, #24377 ), #9861, .F. ) ;
#50862=CARTESIAN_POINT ( 'NONE',  ( 6.879999999999995453, 43.00000000000000000, 6.250000000000000000 ) ) ;
#50870=CARTESIAN_POINT ( 'NONE',  ( -7.754989057094395122, 84.52548903604052555, -4.000000000000000000 ) ) ;
#50882=CARTESIAN_POINT ( 'NONE',  ( -3.749999999999999112, 78.07179676972445748, -4.250000000000000000 ) ) ;
#50883=CARTESIAN_POINT ( 'NONE',  ( 3.969999999999999751, 36.75000000000000000, -2.750000000000000000 ) ) ;
#50893=ORIENTED_EDGE ( 'NONE', *, *, #14032, .T. ) ;
#50894=CARTESIAN_POINT ( 'NONE',  ( -10.60841941975015601, -98.07601481626471696, -4.000000000000000000 ) ) ;
#50897=CARTESIAN_POINT ( 'NONE',  ( -3.772056942336352581, -0.8420495280537244609, 4.000000000000000000 ) ) ;
#50908=ADVANCED_FACE ( 'NONE', ( #55850 ), #24866, .F. ) ;
#50914=ORIENTED_EDGE ( 'NONE', *, *, #40282, .T. ) ;
#50916=DIRECTION ( 'NONE',  ( 1.000000000000000000, -0.000000000000000000, -0.000000000000000000 ) ) ;
#50921=MECHANICAL_DESIGN_GEOMETRIC_PRESENTATION_REPRESENTATION('',(#14244),#20598);
#50926=AXIS2_PLACEMENT_3D ( 'NONE', #46157, #5333, #60157 ) ;
#50968=CARTESIAN_POINT ( 'NONE',  ( -7.072497013479695838, -84.40007040885043921, 2.500000000001209255 ) ) ;
#50969=ADVANCED_FACE ( 'NONE', ( #25364 ), #55349, .F. ) ;
#50971=CYLINDRICAL_SURFACE ( 'NONE', #41987, 2.000000000000000000 ) ;
#50987=DIRECTION ( 'NONE',  ( -0.000000000000000000, 0.000000000000000000, 1.000000000000000000 ) ) ;
#51008=CARTESIAN_POINT ( 'NONE',  ( -3.271887613349915735, -0.8417457659429951056, -2.500000000000000444 ) ) ;
#51009=VECTOR ( 'NONE', #8649, 1000.000000000000000 ) ;
#51015=DIRECTION ( 'NONE',  ( 1.000000000000000000, -3.469446951953623261E-15, 0.000000000000000000 ) ) ;
#51016=ORIENTED_EDGE ( 'NONE', *, *, #74405, .F. ) ;
#51018=EDGE_CURVE ( 'NONE', #91827, #3599, #93838, .T. ) ;
#51027=DIRECTION ( 'NONE',  ( 0.000000000000000000, 0.000000000000000000, -1.000000000000000000 ) ) ;
#51028=SURFACE_STYLE_FILL_AREA ( #35533 ) ;
#51030=ORIENTED_EDGE ( 'NONE', *, *, #83876, .T. ) ;
#51041=DIRECTION ( 'NONE',  ( 0.000000000000000000, 0.000000000000000000, -1.000000000000000000 ) ) ;
#51045=FILL_AREA_STYLE_COLOUR ( '', #2557 ) ;
#51047=EDGE_LOOP ( 'NONE', ( #90436, #32881, #62891, #96205 ) ) ;
#51059=EDGE_CURVE ( 'NONE', #74593, #96688, #750, .T. ) ;
#51062=ORIENTED_EDGE ( 'NONE', *, *, #69537, .T. ) ;
#51064=( NAMED_UNIT ( * ) PLANE_ANGLE_UNIT ( ) SI_UNIT ( $, .RADIAN. ) );
#51076=ORIENTED_EDGE ( 'NONE', *, *, #20955, .T. ) ;
#51079=ORIENTED_EDGE ( 'NONE', *, *, #41939, .F. ) ;
#51081=ORIENTED_EDGE ( 'NONE', *, *, #81450, .T. ) ;
#51086=CARTESIAN_POINT ( 'NONE',  ( 18.00000000000000711, 77.36199599866324661, -4.193285603388146043 ) ) ;
#51090=EDGE_CURVE ( 'NONE', #93614, #62473, #8707, .T. ) ;
#51091=DIRECTION ( 'NONE',  ( 0.000000000000000000, -0.000000000000000000, 1.000000000000000000 ) ) ;
#51122=FILL_AREA_STYLE ('',( #21129 ) ) ;
#51125=PRESENTATION_STYLE_ASSIGNMENT (( #11156 ) ) ;
#51131=CARTESIAN_POINT ( 'NONE',  ( -11.07532115247915883, -96.02567358739618442, -3.999999999999774403 ) ) ;
#51135=CYLINDRICAL_SURFACE ( 'NONE', #96113, 0.2500000000000002220 ) ;
#51136=EDGE_CURVE ( 'NONE', #55108, #32731, #78944, .T. ) ;
#51149=AXIS2_PLACEMENT_3D ( 'NONE', #9957, #68986, #76965 ) ;
#51162=CARTESIAN_POINT ( 'NONE',  ( -7.750000000000000000, 80.07179676972448590, 6.250000000000000000 ) ) ;
#51165=CARTESIAN_POINT ( 'NONE',  ( 4.145753578648191606, -0.8370341202481567100, 2.499999999999999556 ) ) ;
#51168=EDGE_LOOP ( 'NONE', ( #57356, #10203, #6566, #88086 ) ) ;
#51176=CARTESIAN_POINT ( 'NONE',  ( -11.07542066933276992, -96.02453755662239132, 3.750000000000000000 ) ) ;
#51184=EDGE_CURVE ( 'NONE', #60118, #2137, #69374, .T. ) ;
#51187=CARTESIAN_POINT ( 'NONE',  ( -11.64999999999999680, 98.49999999999998579, 8.000000000000000000 ) ) ;
#51189=ORIENTED_EDGE ( 'NONE', *, *, #30160, .F. ) ;
#51203=VERTEX_POINT ( 'NONE', #34801 ) ;
#51213=DIRECTION ( 'NONE',  ( -1.000000000000000000, 0.000000000000000000, 0.000000000000000000 ) ) ;
#51219=AXIS2_PLACEMENT_3D ( 'NONE', #46486, #39978, #92963 ) ;
#51237=DIRECTION ( 'NONE',  ( 0.000000000000000000, 1.000000000000000000, 0.000000000000000000 ) ) ;
#51251=CARTESIAN_POINT ( 'NONE',  ( 15.00000000000000178, 73.00000000000000000, 4.000000000000000000 ) ) ;
#51262=CARTESIAN_POINT ( 'NONE',  ( 8.880000000000000782, 1.116573172248542834E-15, 6.250000000000000000 ) ) ;
#51263=SURFACE_SIDE_STYLE ('',( #96787 ) ) ;
#51276=CARTESIAN_POINT ( 'NONE',  ( -7.750000000000000000, 79.82179676972448590, 6.500000000000000888 ) ) ;
#51284=UNCERTAINTY_MEASURE_WITH_UNIT (LENGTH_MEASURE( 1.000000000000000082E-05 ), #1583, 'distance_accuracy_value', 'NONE');
#51285=AXIS2_PLACEMENT_3D ( 'NONE', #28999, #67515, #22517 ) ;
#51293=DIRECTION ( 'NONE',  ( 0.000000000000000000, 0.000000000000000000, 1.000000000000000000 ) ) ;
#51301=( NAMED_UNIT ( * ) SI_UNIT ( $, .STERADIAN. ) SOLID_ANGLE_UNIT ( ) );
#51327=AXIS2_PLACEMENT_3D ( 'NONE', #30829, #98878, #31805 ) ;
#51372=DIRECTION ( 'NONE',  ( 0.000000000000000000, 1.000000000000000000, -0.000000000000000000 ) ) ;
#51379=B_SPLINE_SURFACE_WITH_KNOTS ( 'NONE', 3, 1, ( 
 ( #97503, #43480 ),
 ( #67479, #97011 ),
 ( #42509, #4523 ),
 ( #27495, #89485 ),
 ( #57988, #88493 ),
 ( #20996, #51483 ),
 ( #83955, #24451 ),
 ( #44961, #37485 ),
 ( #52954, #46447 ),
 ( #83465, #16449 ),
 ( #22479, #54429 ),
 ( #91944, #46927 ),
 ( #1463, #23475 ),
 ( #14986, #31914 ),
 ( #84938, #77419 ),
 ( #69446, #91455 ),
 ( #45457, #68959 ),
 ( #7485, #53446 ) ),
 .UNSPECIFIED., .F., .F., .F.,
 ( 4, 2, 2, 2, 2, 2, 2, 2, 4 ),
 ( 2, 2 ),
 ( 0.1401766717507622051, 0.2499999999999989453, 0.3749999999999986122, 0.4374999999999986677, 0.4999999999999986677, 0.7499999999999992228, 0.8749999999999996669, 0.9374999999999997780, 1.000000000000000000 ),
 ( 0.000000000000000000, 1.000000000000000000 ),
 .UNSPECIFIED. ) ;
#51382=DIRECTION ( 'NONE',  ( -1.000000000000000000, 0.000000000000000000, 0.000000000000000000 ) ) ;
#51385=EDGE_CURVE ( 'NONE', #5021, #20454, #15311, .T. ) ;
#51390=FACE_OUTER_BOUND ( 'NONE', #78480, .T. ) ;
#51391=CARTESIAN_POINT ( 'NONE',  ( -10.54707717933094813, -44.61285707880912810, -4.000000000000000000 ) ) ;
#51397=LINE ( 'NONE', #82376, #57569 ) ;
#51401=CARTESIAN_POINT ( 'NONE',  ( 6.880000000000009663, 40.99999999999999289, 6.250000000000000000 ) ) ;
#51405=CIRCLE ( 'NONE', #53040, 0.2500000000000002220 ) ;
#51411=( BOUNDED_SURFACE ( )  B_SPLINE_SURFACE ( 3, 2, ( 
 ( #33214, #23781, #76754 ),
 ( #48222, #38769, #61740 ),
 ( #24754, #86234, #54247 ),
 ( #1287, #1771, #63709 ),
 ( #24267, #9743, #84759 ),
 ( #94212, #84280, #25743 ),
 ( #31244, #85252, #32228 ),
 ( #9247, #62728, #40244 ) ),
 .UNSPECIFIED., .F., .F., .F. ) 
 B_SPLINE_SURFACE_WITH_KNOTS ( ( 4, 2, 2, 4 ),
 ( 3, 3 ),
 ( 0.000000000000000000, 0.0004516266542298917803, 0.0009032533084597835606, 0.001806506616919567121 ),
 ( 0.000000000000000000, 1.000000000000000000 ),
 .UNSPECIFIED. ) 
 GEOMETRIC_REPRESENTATION_ITEM ( )  RATIONAL_B_SPLINE_SURFACE ( (
 ( 1.000000000000000000, 0.7071067811865475727, 1.000000000000000000),
 ( 1.000000000000000000, 0.7557133596827383393, 1.000000000000000000),
 ( 1.000000000000000000, 0.7976722695483360326, 1.000000000000000000),
 ( 1.000000000000000000, 0.8702934545469085403, 1.000000000000000000),
 ( 1.000000000000000000, 0.9009816261292108441, 1.000000000000000000),
 ( 1.000000000000000000, 0.9749059260391067516, 1.000000000000000000),
 ( 1.000000000000000000, 1.000014990205005949, 1.000000000000000000),
 ( 1.000000000000000000, 1.000000000000000000, 1.000000000000000000) ) ) 
 REPRESENTATION_ITEM ( '' )  SURFACE ( )  );
#51426=EDGE_LOOP ( 'NONE', ( #34603, #24002, #45503, #66842 ) ) ;
#51457=CARTESIAN_POINT ( 'NONE',  ( 12.50465990577749409, 56.99999999999999289, 2.900000000000000355 ) ) ;
#51465=ADVANCED_FACE ( 'NONE', ( #80311 ), #81295, .T. ) ;
#51467=DIRECTION ( 'NONE',  ( -0.000000000000000000, -0.000000000000000000, 1.000000000000000000 ) ) ;
#51468=CARTESIAN_POINT ( 'NONE',  ( 11.04805072354886875, -95.57913125337492488, 4.000000000000000000 ) ) ;
#51470=ORIENTED_EDGE ( 'NONE', *, *, #8291, .T. ) ;
#51475=UNCERTAINTY_MEASURE_WITH_UNIT (LENGTH_MEASURE( 1.000000000000000082E-05 ), #67841, 'distance_accuracy_value', 'NONE');
#51483=CARTESIAN_POINT ( 'NONE',  ( 6.732888861736110009, -58.30752899003807954, -3.750000000000000888 ) ) ;
#51484=ORIENTED_EDGE ( 'NONE', *, *, #47080, .F. ) ;
#51491=CARTESIAN_POINT ( 'NONE',  ( 8.630000000000000782, 1.085138116723527427E-15, 3.750000000000000000 ) ) ;
#51500=DIRECTION ( 'NONE',  ( -0.08715574274765112983, -0.9961946980917461003, -0.000000000000000000 ) ) ;
#51519=SURFACE_STYLE_FILL_AREA ( #21028 ) ;
#51526=CARTESIAN_POINT ( 'NONE',  ( 5.129999999999995453, 43.00000000000000000, -6.500000000000000888 ) ) ;
#51541=CARTESIAN_POINT ( 'NONE',  ( -7.750000000000000000, 79.82179676972448590, -6.250000000000000000 ) ) ;
#51544=EDGE_CURVE ( 'NONE', #92036, #65098, #69385, .T. ) ;
#51545=CARTESIAN_POINT ( 'NONE',  ( 11.10711265426551897, -52.69644047981464041, -3.750000000000001776 ) ) ;
#51554=SURFACE_STYLE_FILL_AREA ( #90522 ) ;
#51582=CIRCLE ( 'NONE', #83564, 2.999999999999999112 ) ;
#51593=EDGE_CURVE ( 'NONE', #16419, #53779, #91723, .T. ) ;
#51594=DIRECTION ( 'NONE',  ( -0.000000000000000000, -0.000000000000000000, -1.000000000000000000 ) ) ;
#51595=ORIENTED_EDGE ( 'NONE', *, *, #90184, .T. ) ;
#51602=EDGE_LOOP ( 'NONE', ( #64540, #19480, #780, #49440 ) ) ;
#51603=FACE_OUTER_BOUND ( 'NONE', #94228, .T. ) ;
#51604=CARTESIAN_POINT ( 'NONE',  ( -5.329638162525626832, -28.67157456369669788, 3.750000000000001332 ) ) ;
#51610=DIRECTION ( 'NONE',  ( 0.000000000000000000, 1.000000000000000000, -1.734723475976805517E-15 ) ) ;
#51620=AXIS2_PLACEMENT_3D ( 'NONE', #64108, #2182, #24670 ) ;
#51622=ORIENTED_EDGE ( 'NONE', *, *, #87940, .F. ) ;
#51628=FACE_BOUND ( 'NONE', #97700, .T. ) ;
#51630=EDGE_CURVE ( 'NONE', #63243, #55430, #40634, .T. ) ;
#51632=DIRECTION ( 'NONE',  ( 0.000000000000000000, 0.000000000000000000, -1.000000000000000000 ) ) ;
#51653=MECHANICAL_DESIGN_GEOMETRIC_PRESENTATION_REPRESENTATION('',(#70869),#43643);
#51666=CARTESIAN_POINT ( 'NONE',  ( 4.406177045959971394, -8.255047197857166452, 2.500000000000000000 ) ) ;
#51668=ORIENTED_EDGE ( 'NONE', *, *, #21004, .F. ) ;
#51695=SHAPE_REPRESENTATION ( '1.0 Fixed Jaw', ( #27931 ), #34259 ) ;
#51712=VERTEX_POINT ( 'NONE', #15292 ) ;
#51714=VECTOR ( 'NONE', #27173, 1000.000000000000000 ) ;
#51720=EDGE_CURVE ( 'NONE', #37917, #67494, #60758, .T. ) ;
#51722=VECTOR ( 'NONE', #59608, 1000.000000000000000 ) ;
#51731=FILL_AREA_STYLE_COLOUR ( '', #33703 ) ;
#51761=LINE ( 'NONE', #43754, #69434 ) ;
#51762=PLANE ( 'NONE',  #20060 ) ;
#51766=ORIENTED_EDGE ( 'NONE', *, *, #75792, .T. ) ;
#51768=CARTESIAN_POINT ( 'NONE',  ( 11.10647200087231568, -65.08385396170790216, -4.000000000000000000 ) ) ;
#51776=CARTESIAN_POINT ( 'NONE',  ( 6.879999999999995453, 43.00000000000000000, -4.000000000000000000 ) ) ;
#51794=AXIS2_PLACEMENT_3D ( 'NONE', #9453, #85955, #76961 ) ;
#51796=CARTESIAN_POINT ( 'NONE',  ( -3.878348535191012303, -3.630205232349507760, 4.000000000000000000 ) ) ;
#51797=EDGE_LOOP ( 'NONE', ( #75215, #37689, #53537, #87010 ) ) ;
#51799=ORIENTED_EDGE ( 'NONE', *, *, #51956, .F. ) ;
#51813=ORIENTED_EDGE ( 'NONE', *, *, #39123, .F. ) ;
#51824=ORIENTED_EDGE ( 'NONE', *, *, #90290, .T. ) ;
#51839=PRESENTATION_STYLE_ASSIGNMENT (( #82326 ) ) ;
#51852=AXIS2_PLACEMENT_3D ( 'NONE', #17939, #39468, #55446 ) ;
#51855=TOROIDAL_SURFACE ( 'NONE', #8753, 0.5000000000000000000, 0.2500000000000000000 ) ;
#51864=VECTOR ( 'NONE', #33746, 1000.000000000000000 ) ;
#51867=ORIENTED_EDGE ( 'NONE', *, *, #25686, .T. ) ;
#51868=FACE_OUTER_BOUND ( 'NONE', #86175, .T. ) ;
#51894=SURFACE_SIDE_STYLE ('',( #7394 ) ) ;
#51917=ORIENTED_EDGE ( 'NONE', *, *, #34321, .F. ) ;
#51924=EDGE_LOOP ( 'NONE', ( #48721, #39393, #8084, #95438 ) ) ;
#51927=CARTESIAN_POINT ( 'NONE',  ( 4.691428608706885051, -2.693193260553968127, 4.000000000000000000 ) ) ;
#51929=FILL_AREA_STYLE_COLOUR ( '', #27603 ) ;
#51952=CARTESIAN_POINT ( 'NONE',  ( 6.432108699068925795, -88.20011490510430008, -3.750000000000000000 ) ) ;
#51953=EDGE_LOOP ( 'NONE', ( #46872, #24424, #34669, #42975, #29138 ) ) ;
#51956=EDGE_CURVE ( 'NONE', #59823, #32731, #82215, .T. ) ;
#51958=DIRECTION ( 'NONE',  ( -0.08715574274765112983, -0.9961946980917461003, -0.000000000000000000 ) ) ;
#51966=CARTESIAN_POINT ( 'NONE',  ( -6.606690058644155705, -50.93246948813188624, 2.500000000001612044 ) ) ;
#51969=CARTESIAN_POINT ( 'NONE',  ( 9.511407825468095822, -15.49433182432920120, 4.000000000000000000 ) ) ;
#51975=AXIS2_PLACEMENT_3D ( 'NONE', #63814, #8375, #48333 ) ;
#51986=VERTEX_POINT ( 'NONE', #15776 ) ;
#51993=CARTESIAN_POINT ( 'NONE',  ( 18.00000000000000000, 78.50170875210521615, 3.769097870606325174 ) ) ;
#52002=AXIS2_PLACEMENT_3D ( 'NONE', #43723, #82214, #57732 ) ;
#52025=LINE ( 'NONE', #7021, #36817 ) ;
#52027=VERTEX_POINT ( 'NONE', #8267 ) ;
#52038=AXIS2_PLACEMENT_3D ( 'NONE', #28242, #42273, #88746 ) ;
#52041=CARTESIAN_POINT ( 'NONE',  ( -6.607869636366940469, -50.96183896326462559, -4.000000000000000000 ) ) ;
#52043=ORIENTED_EDGE ( 'NONE', *, *, #44520, .T. ) ;
#52048=DIRECTION ( 'NONE',  ( -0.06975647374412534407, -0.9975640502598241977, 0.000000000000000000 ) ) ;
#52054=CARTESIAN_POINT ( 'NONE',  ( 8.629999999999995453, 41.24999999999999289, -6.500000000000000888 ) ) ;
#52056=LINE ( 'NONE', #5078, #73728 ) ;
#52073=ORIENTED_EDGE ( 'NONE', *, *, #15680, .F. ) ;
#52085=CARTESIAN_POINT ( 'NONE',  ( 10.76914169791313292, -96.07995077553798069, 4.000000000000000000 ) ) ;
#52117=DIRECTION ( 'NONE',  ( 0.8070303256584298035, -0.5905099943842175847, 0.000000000000000000 ) ) ;
#52126=CARTESIAN_POINT ( 'NONE',  ( 6.757727703329182489, -58.31565150548815524, -3.750000000000000444 ) ) ;
#52132=AXIS2_PLACEMENT_3D ( 'NONE', #91058, #51594, #46066 ) ;
#52137=VERTEX_POINT ( 'NONE', #97706 ) ;
#52147=ADVANCED_FACE ( 'NONE', ( #83668 ), #98701, .F. ) ;
#52148=CIRCLE ( 'NONE', #24983, 2.999999999999999112 ) ;
#52157=CIRCLE ( 'NONE', #44145, 0.2500000000000002220 ) ;
#52183=EDGE_CURVE ( 'NONE', #38304, #37672, #56666, .T. ) ;
#52187=ADVANCED_FACE ( 'NONE', ( #30150 ), #38178, .T. ) ;
#52202=CARTESIAN_POINT ( 'NONE',  ( -15.00000000000000000, 83.99999999999998579, 8.000000000000000000 ) ) ;
#52204=CARTESIAN_POINT ( 'NONE',  ( -3.499999999999998668, 1.019547802438465434, -3.750000000000000000 ) ) ;
#52210=CYLINDRICAL_SURFACE ( 'NONE', #5886, 3.000000000000000888 ) ;
#52222=CIRCLE ( 'NONE', #80979, 0.2500000000000002220 ) ;
#52226=ORIENTED_EDGE ( 'NONE', *, *, #76361, .F. ) ;
#52231=FILL_AREA_STYLE_COLOUR ( '', #5719 ) ;
#52257=CARTESIAN_POINT ( 'NONE',  ( 11.43665875882196481, -81.61983315978024223, -3.750000000000000000 ) ) ;
#52267=SURFACE_STYLE_USAGE ( .BOTH. , #66270 ) ;
#52271=ORIENTED_EDGE ( 'NONE', *, *, #74093, .T. ) ;
#52287=( LENGTH_UNIT ( ) NAMED_UNIT ( * ) SI_UNIT ( .MILLI., .METRE. ) );
#52297=CONICAL_SURFACE ( 'NONE', #98652, 1.249999999999987121, 1.029744258676652979 ) ;
#52300=AXIS2_PLACEMENT_3D ( 'NONE', #76271, #36797, #28786 ) ;
#52302=ADVANCED_FACE ( 'NONE', ( #85636 ), #31634, .T. ) ;
#52306=ORIENTED_EDGE ( 'NONE', *, *, #44311, .F. ) ;
#52312=DIRECTION ( 'NONE',  ( 1.000000000000000000, 0.000000000000000000, 0.000000000000000000 ) ) ;
#52325=CARTESIAN_POINT ( 'NONE',  ( 4.441305562537879226, -2.692695313950745017, -3.749999999999999556 ) ) ;
#52327=FACE_OUTER_BOUND ( 'NONE', #94827, .T. ) ;
#52334=EDGE_CURVE ( 'NONE', #95619, #14052, #86132, .T. ) ;
#52340=CARTESIAN_POINT ( 'NONE',  ( 6.829574850505125028, -88.00372650098202598, -2.750000000000000888 ) ) ;
#52343=FACE_OUTER_BOUND ( 'NONE', #54599, .T. ) ;
#52349=CARTESIAN_POINT ( 'NONE',  ( -3.750000000000000000, 10.25000000000000000, 2.750000000000000000 ) ) ;
#52354=LINE ( 'NONE', #37371, #16155 ) ;
#52358=CARTESIAN_POINT ( 'NONE',  ( -6.732636091893173358, -88.11213685669363826, 2.750000000000000000 ) ) ;
#52363=CARTESIAN_POINT ( 'NONE',  ( -6.787853370348170934, -86.25412202734862888, -2.500000000000000888 ) ) ;
#52388=EDGE_CURVE ( 'NONE', #18642, #82286, #11927, .T. ) ;
#52391=ADVANCED_FACE ( 'NONE', ( #48114 ), #1173, .T. ) ;
#52403=ORIENTED_EDGE ( 'NONE', *, *, #52708, .F. ) ;
#52415=DIRECTION ( 'NONE',  ( -1.000000000000000000, 0.000000000000000000, 0.000000000000000000 ) ) ;
#52416=CARTESIAN_POINT ( 'NONE',  ( -8.399999999999998579, 98.49999999999998579, 8.000000000000000000 ) ) ;
#52424=ADVANCED_FACE ( 'NONE', ( #49581 ), #74209, .T. ) ;
#52427=AXIS2_PLACEMENT_3D ( 'NONE', #12077, #33584, #10613 ) ;
#52438=DIRECTION ( 'NONE',  ( 6.938893903907222067E-15, -1.000000000000000000, 0.000000000000000000 ) ) ;
#52459=UNCERTAINTY_MEASURE_WITH_UNIT (LENGTH_MEASURE( 1.000000000000000082E-05 ), #25346, 'distance_accuracy_value', 'NONE');
#52460=CARTESIAN_POINT ( 'NONE',  ( -8.350463100005470096, 86.22728700194058149, 4.047063141920189899 ) ) ;
#52473=EDGE_CURVE ( 'NONE', #26894, #30756, #41134, .T. ) ;
#52480=EDGE_LOOP ( 'NONE', ( #95602, #81314, #64499, #61627 ) ) ;
#52496=ORIENTED_EDGE ( 'NONE', *, *, #97772, .F. ) ;
#52507=CARTESIAN_POINT ( 'NONE',  ( -8.900000000000002132, 75.76920769491746910, -3.000000000000000000 ) ) ;
#52524=CARTESIAN_POINT ( 'NONE',  ( 11.01442511525662482, -96.10567886042495900, -3.749999999999999112 ) ) ;
#52525=CARTESIAN_POINT ( 'NONE',  ( -7.121448108955550360, -73.25984652122872376, -4.000000000000001776 ) ) ;
#52531=DIRECTION ( 'NONE',  ( 1.000000000000000000, 0.000000000000000000, 0.000000000000000000 ) ) ;
#52532=CARTESIAN_POINT ( 'NONE',  ( -11.88860330017057443, 90.28199325634325589, -6.828299344296716811 ) ) ;
#52542=ORIENTED_EDGE ( 'NONE', *, *, #69083, .F. ) ;
#52545=CARTESIAN_POINT ( 'NONE',  ( 8.879999999999995453, 41.24999999999999289, 4.000000000000000000 ) ) ;
#52563=CIRCLE ( 'NONE', #97265, 1.750000000000001554 ) ;
#52571=ORIENTED_EDGE ( 'NONE', *, *, #48882, .F. ) ;
#52575=CARTESIAN_POINT ( 'NONE',  ( 3.969999999999999751, 9.750000000000000000, -4.000000000000000000 ) ) ;
#52589=VECTOR ( 'NONE', #50916, 1000.000000000000000 ) ;
#52590=DIRECTION ( 'NONE',  ( 0.000000000000000000, 0.000000000000000000, -1.000000000000000000 ) ) ;
#52600=CARTESIAN_POINT ( 'NONE',  ( -4.247994584727555534, -13.56436116443237516, -2.750000000000000444 ) ) ;
#52604=CIRCLE ( 'NONE', #35036, 10.00000000000000178 ) ;
#52627=LINE ( 'NONE', #22143, #12629 ) ;
#52639=ORIENTED_EDGE ( 'NONE', *, *, #78155, .T. ) ;
#52647=CARTESIAN_POINT ( 'NONE',  ( -8.028887233583267502, -1.053223610202706162, 4.000000000000000000 ) ) ;
#52653=CARTESIAN_POINT ( 'NONE',  ( 0.000000000000000000, -97.00000000000000000, 3.750000000000000000 ) ) ;
#52662=EDGE_LOOP ( 'NONE', ( #97188, #39544, #10882, #61200, #14237, #7187, #87594, #39421 ) ) ;
#52673=ORIENTED_EDGE ( 'NONE', *, *, #30930, .T. ) ;
#52682=CARTESIAN_POINT ( 'NONE',  ( 8.880000000000020322, 80.07179676972448590, 6.500000000000000888 ) ) ;
#52686=DIRECTION ( 'NONE',  ( 1.000000000000000000, 0.000000000000000000, 0.000000000000000000 ) ) ;
#52687=EDGE_LOOP ( 'NONE', ( #27805, #70994, #31627, #48836 ) ) ;
#52708=EDGE_CURVE ( 'NONE', #38399, #79527, #19976, .T. ) ;
#52726=AXIS2_PLACEMENT_3D ( 'NONE', #30661, #9154, #92645 ) ;
#52728=FILL_AREA_STYLE_COLOUR ( '', #94779 ) ;
#52732=VERTEX_POINT ( 'NONE', #73362 ) ;
#52742=EDGE_CURVE ( 'NONE', #9920, #40011, #79079, .T. ) ;
#52743=EDGE_LOOP ( 'NONE', ( #59681, #17475, #4237, #71840 ) ) ;
#52745=CARTESIAN_POINT ( 'NONE',  ( 7.079515573063599021, -88.00917032380691296, 4.000000000000000000 ) ) ;
#52750=( GEOMETRIC_REPRESENTATION_CONTEXT ( 3 ) GLOBAL_UNCERTAINTY_ASSIGNED_CONTEXT ( ( #65148 ) ) GLOBAL_UNIT_ASSIGNED_CONTEXT ( ( #87270, #1350, #34754 ) ) REPRESENTATION_CONTEXT ( 'NONE', 'WORKASPACE' ) );
#52758=ORIENTED_EDGE ( 'NONE', *, *, #72137, .T. ) ;
#52766=DIRECTION ( 'NONE',  ( -0.000000000000000000, -0.000000000000000000, -1.000000000000000000 ) ) ;
#52774=CARTESIAN_POINT ( 'NONE',  ( -3.750000001621175638, 0.08803144853710938300, 4.000000000000000000 ) ) ;
#52775=EDGE_CURVE ( 'NONE', #15093, #5021, #4402, .T. ) ;
#52785=AXIS2_PLACEMENT_3D ( 'NONE', #3214, #79196, #95680 ) ;
#52793=VERTEX_POINT ( 'NONE', #57377 ) ;
#52802=ORIENTED_EDGE ( 'NONE', *, *, #67725, .F. ) ;
#52818=DIRECTION ( 'NONE',  ( 1.000000000000000000, 0.000000000000000000, 0.000000000000000000 ) ) ;
#52824=B_SPLINE_CURVE_WITH_KNOTS ( 'NONE', 3,
 ( #19399, #71900, #33883, #39939, #3424, #86430, #2948, #48414, #25921, #78917, #10428, #11402, #79418, #64387, #79895, #94898, #41924, #3914, #64871, #9437, #95395, #90338, #73868, #42402 ),
 .UNSPECIFIED., .F., .F.,
 ( 4, 2, 2, 2, 2, 2, 2, 2, 2, 2, 2, 4 ),
 ( 6.505213034913026604E-19, 0.003101839872476766513, 0.006203679744953532159, 0.01240735948990705911, 0.02481471897981411823, 0.04962943795962823645, 0.06203679744953529557, 0.07444415693944235468, 0.08685151642934942073, 0.09305519617430298152, 0.09615703604677973415, 0.09925887591925647291 ),
 .UNSPECIFIED. ) ;
#52827=CARTESIAN_POINT ( 'NONE',  ( 4.471066085427381154, -3.611416924293318953, -2.750000000000000000 ) ) ;
#52831=CARTESIAN_POINT ( 'NONE',  ( -10.98829462902744858, 46.98606209026556968, 2.900000000000000355 ) ) ;
#52837=CARTESIAN_POINT ( 'NONE',  ( -6.000000000000014211, 80.07179676972448590, 6.500000000000000888 ) ) ;
#52842=( NAMED_UNIT ( * ) PLANE_ANGLE_UNIT ( ) SI_UNIT ( $, .RADIAN. ) );
#52858=VECTOR ( 'NONE', #71333, 1000.000000000000000 ) ;
#52861=EDGE_CURVE ( 'NONE', #51203, #10110, #97223, .T. ) ;
#52870=CYLINDRICAL_SURFACE ( 'NONE', #46438, 0.2500000000000002220 ) ;
#52890=AXIS2_PLACEMENT_3D ( 'NONE', #30836, #97390, #66872 ) ;
#52897=ORIENTED_EDGE ( 'NONE', *, *, #14142, .F. ) ;
#52900=MECHANICAL_DESIGN_GEOMETRIC_PRESENTATION_REPRESENTATION('',(#46481),#62454);
#52905=CARTESIAN_POINT ( 'NONE',  ( -8.900000000000000355, 75.76920769491746910, 2.900000000000000355 ) ) ;
#52919=AXIS2_PLACEMENT_3D ( 'NONE', #16491, #86463, #85970 ) ;
#52926=CARTESIAN_POINT ( 'NONE',  ( 9.838578643762680542, 27.00180849546987716, 3.000000000000000000 ) ) ;
#52938=CARTESIAN_POINT ( 'NONE',  ( 4.645843784090633477, -0.8374430341443380721, -4.000000000000000888 ) ) ;
#52941=FACE_OUTER_BOUND ( 'NONE', #31857, .T. ) ;
#52947=CARTESIAN_POINT ( 'NONE',  ( -10.31693093662312144, 89.21683745890891259, 5.695017665638099302 ) ) ;
#52952=CARTESIAN_POINT ( 'NONE',  ( -7.232415441807424017, -88.12698951299773853, 3.750000000000000000 ) ) ;
#52954=CARTESIAN_POINT ( 'NONE',  ( 6.452519493965914954, -47.68837976023561964, -2.750000000000000000 ) ) ;
#52960=CARTESIAN_POINT ( 'NONE',  ( 2.550000000000003819, 99.99999999999998579, 8.000000000000000000 ) ) ;
#52968=VERTEX_POINT ( 'NONE', #75336 ) ;
#53008=CARTESIAN_POINT ( 'NONE',  ( 0.4400000000000020006, 1.019547802438468986, -2.500000000000000000 ) ) ;
#53011=DIRECTION ( 'NONE',  ( -1.000000000000000000, -0.000000000000000000, 0.000000000000000000 ) ) ;
#53013=CARTESIAN_POINT ( 'NONE',  ( -5.070949216135518967, -24.98410106518212714, -4.000000000003224088 ) ) ;
#53019=CARTESIAN_POINT ( 'NONE',  ( -9.024359497401759356, 75.07164295747612925, -2.900000000000000799 ) ) ;
#53025=DIRECTION ( 'NONE',  ( 1.000000000000000000, 0.000000000000000000, 0.000000000000000000 ) ) ;
#53031=DIRECTION ( 'NONE',  ( 1.000000000000000000, 0.000000000000000000, 0.000000000000000000 ) ) ;
#53040=AXIS2_PLACEMENT_3D ( 'NONE', #70255, #9742, #32721 ) ;
#53058=EDGE_LOOP ( 'NONE', ( #75558, #69067, #33569 ) ) ;
#53061=ORIENTED_EDGE ( 'NONE', *, *, #51018, .T. ) ;
#53062=DIRECTION ( 'NONE',  ( 0.9975640502598243087, -0.06975647374412452528, -0.000000000000000000 ) ) ;
#53063=SURFACE_STYLE_FILL_AREA ( #23088 ) ;
#53064=EDGE_CURVE ( 'NONE', #32841, #50286, #13630, .T. ) ;
#53081=FILL_AREA_STYLE ('',( #46565 ) ) ;
#53085=LINE ( 'NONE', #82599, #73903 ) ;
#53104=SURFACE_STYLE_USAGE ( .BOTH. , #76102 ) ;
#53115=UNCERTAINTY_MEASURE_WITH_UNIT (LENGTH_MEASURE( 1.000000000000000082E-05 ), #82735, 'distance_accuracy_value', 'NONE');
#53140=CARTESIAN_POINT ( 'NONE',  ( -11.26387636256299274, -65.37812658113601572, 4.000000000000000000 ) ) ;
#53145=AXIS2_PLACEMENT_3D ( 'NONE', #97242, #28710, #59698 ) ;
#53147=CARTESIAN_POINT ( 'NONE',  ( -7.750000000000000000, 40.74999999999999289, 4.250000000000000000 ) ) ;
#53149=AXIS2_PLACEMENT_3D ( 'NONE', #96400, #14376, #67363 ) ;
#53156=CYLINDRICAL_SURFACE ( 'NONE', #86056, 0.09999999999999982514 ) ;
#53172=AXIS2_PLACEMENT_3D ( 'NONE', #32360, #24890, #77865 ) ;
#53183=CIRCLE ( 'NONE', #10084, 7.250000000000002665 ) ;
#53185=CARTESIAN_POINT ( 'NONE',  ( 0.000000000000000000, -97.00000000000000000, 4.000000000000000000 ) ) ;
#53201=CARTESIAN_POINT ( 'NONE',  ( 0.000000000000000000, 80.32179676972448590, -4.000000000000000000 ) ) ;
#53216=CARTESIAN_POINT ( 'NONE',  ( 8.879999999999991900, 21.00000000000000000, -2.899999999999999911 ) ) ;
#53217=AXIS2_PLACEMENT_3D ( 'NONE', #29599, #24598, #55063 ) ;
#53218=DIRECTION ( 'NONE',  ( 0.000000000000000000, 0.000000000000000000, -1.000000000000000000 ) ) ;
#53236=( NAMED_UNIT ( * ) SI_UNIT ( $, .STERADIAN. ) SOLID_ANGLE_UNIT ( ) );
#53237=DIRECTION ( 'NONE',  ( 1.000000000000000000, 0.000000000000000000, 0.000000000000000000 ) ) ;
#53243=CARTESIAN_POINT ( 'NONE',  ( 10.89310702335901482, -97.65080521010446546, -3.750000000000675016 ) ) ;
#53244=CARTESIAN_POINT ( 'NONE',  ( -3.750000000000000000, 9.750000000000000000, 4.000000000000000000 ) ) ;
#53258=CARTESIAN_POINT ( 'NONE',  ( 12.14357320772536575, 54.02013147999952736, 0.000000000000000000 ) ) ;
#53269=( NAMED_UNIT ( * ) PLANE_ANGLE_UNIT ( ) SI_UNIT ( $, .RADIAN. ) );
#53270=ORIENTED_EDGE ( 'NONE', *, *, #18233, .T. ) ;
#53272=VERTEX_POINT ( 'NONE', #78292 ) ;
#53274=ORIENTED_EDGE ( 'NONE', *, *, #19256, .T. ) ;
#53282=AXIS2_PLACEMENT_3D ( 'NONE', #23771, #39258, #30742 ) ;
#53287=VECTOR ( 'NONE', #43410, 1000.000000000000000 ) ;
#53291=FACE_OUTER_BOUND ( 'NONE', #14290, .T. ) ;
#53296=ADVANCED_FACE ( 'NONE', ( #10303 ), #69824, .T. ) ;
#53310=CARTESIAN_POINT ( 'NONE',  ( -6.867502633528057565, -58.37509997445500431, -2.750000000000000000 ) ) ;
#53317=EDGE_LOOP ( 'NONE', ( #35570, #33176, #82284, #45539 ) ) ;
#53320=CARTESIAN_POINT ( 'NONE',  ( 4.145754220388979228, -0.8370734722079299361, -2.500000000000000888 ) ) ;
#53325=CARTESIAN_POINT ( 'NONE',  ( -19.00000000000000000, 75.76920769491739804, 3.000000000000000000 ) ) ;
#53335=FACE_OUTER_BOUND ( 'NONE', #83586, .T. ) ;
#53336=CARTESIAN_POINT ( 'NONE',  ( -11.51381718487193417, -65.37259455513435569, -3.999999999996394884 ) ) ;
#53339=PRESENTATION_STYLE_ASSIGNMENT (( #7374 ) ) ;
#53341=TOROIDAL_SURFACE ( 'NONE', #85321, 8.250000000000000000, 0.2500000000000000000 ) ;
#53361=( NAMED_UNIT ( * ) SI_UNIT ( $, .STERADIAN. ) SOLID_ANGLE_UNIT ( ) );
#53383=AXIS2_PLACEMENT_3D ( 'NONE', #17848, #17368, #62844 ) ;
#53391=CARTESIAN_POINT ( 'NONE',  ( 4.657035931881701174, -8.268334176800257396, 3.999999999999194866 ) ) ;
#53397=CARTESIAN_POINT ( 'NONE',  ( -3.772056942336352137, -0.8420495280537267924, -4.000000000000000000 ) ) ;
#53415=TOROIDAL_SURFACE ( 'NONE', #91762, 2.250000000000001332, 0.2500000000000000000 ) ;
#53426=DIRECTION ( 'NONE',  ( 1.000000000000000000, 0.000000000000000000, 0.000000000000000000 ) ) ;
#53430=CARTESIAN_POINT ( 'NONE',  ( 5.930053198192434039, -28.64714083316721371, -3.999999999999999112 ) ) ;
#53434=DIRECTION ( 'NONE',  ( 0.000000000000000000, 0.000000000000000000, -1.000000000000000000 ) ) ;
#53446=CARTESIAN_POINT ( 'NONE',  ( 4.380000000000000782, 1.019547802438464545, -3.750000000000000888 ) ) ;
#53460=ORIENTED_EDGE ( 'NONE', *, *, #64756, .F. ) ;
#53464=CARTESIAN_POINT ( 'NONE',  ( 0.6289242262155387841, 20.99999999999999289, 0.000000000000000000 ) ) ;
#53483=CARTESIAN_POINT ( 'NONE',  ( 0.000000000000000000, -97.00000000000000000, 3.750000000000000000 ) ) ;
#53487=VECTOR ( 'NONE', #94872, 1000.000000000000000 ) ;
#53492=CARTESIAN_POINT ( 'NONE',  ( 6.579634127946655475, -87.99828267815715321, -3.250000000000000888 ) ) ;
#53506=LINE ( 'NONE', #37542, #23442 ) ;
#53509=CARTESIAN_POINT ( 'NONE',  ( 8.629999999999995453, 40.99999999999999289, -4.250000000000000000 ) ) ;
#53525=EDGE_LOOP ( 'NONE', ( #58076, #93254, #45537, #65303, #6778 ) ) ;
#53526=ORIENTED_EDGE ( 'NONE', *, *, #6400, .F. ) ;
#53534=EDGE_CURVE ( 'NONE', #2183, #43301, #96731, .T. ) ;
#53537=ORIENTED_EDGE ( 'NONE', *, *, #19126, .T. ) ;
#53543=ORIENTED_EDGE ( 'NONE', *, *, #68204, .F. ) ;
#53547=VECTOR ( 'NONE', #64492, 1000.000000000000000 ) ;
#53551=CARTESIAN_POINT ( 'NONE',  ( 10.58840669699852199, -98.14374106289703548, 4.000000000000000000 ) ) ;
#53561=CARTESIAN_POINT ( 'NONE',  ( -8.399999999999998579, 98.49999999999998579, -8.525133428036873795 ) ) ;
#53566=ORIENTED_EDGE ( 'NONE', *, *, #1785, .F. ) ;
#53574=( NAMED_UNIT ( * ) SI_UNIT ( $, .STERADIAN. ) SOLID_ANGLE_UNIT ( ) );
#53579=ORIENTED_EDGE ( 'NONE', *, *, #47080, .T. ) ;
#53585=CARTESIAN_POINT ( 'NONE',  ( -7.127794346849581686, -80.93619716733994096, -2.750000000000000444 ) ) ;
#53595=CARTESIAN_POINT ( 'NONE',  ( -4.000000000000000000, 10.25000000000000000, 2.750000000000000000 ) ) ;
#53596=VECTOR ( 'NONE', #91205, 1000.000000000000000 ) ;
#53603=DIRECTION ( 'NONE',  ( -1.000000000000000000, -0.000000000000000000, -0.000000000000000000 ) ) ;
#53612=FILL_AREA_STYLE ('',( #91623 ) ) ;
#53621=STYLED_ITEM ( 'NONE', ( #57621 ), #37372 ) ;
#53624=EDGE_CURVE ( 'NONE', #55108, #11363, #50757, .T. ) ;
#53626=ORIENTED_EDGE ( 'NONE', *, *, #56040, .F. ) ;
#53633=CARTESIAN_POINT ( 'NONE',  ( -8.957287532613966263, -19.72663685366264019, 4.000000000000000000 ) ) ;
#53639=ADVANCED_FACE ( 'NONE', ( #66232 ), #87753, .F. ) ;
#53648=ORIENTED_EDGE ( 'NONE', *, *, #70024, .T. ) ;
#53650=ORIENTED_EDGE ( 'NONE', *, *, #83758, .F. ) ;
#53668=CARTESIAN_POINT ( 'NONE',  ( -6.866275848337654253, -80.67678253189122017, 2.500000000000001332 ) ) ;
#53672=CARTESIAN_POINT ( 'NONE',  ( 14.35000000000000142, 98.49999999999998579, -8.525133428036873795 ) ) ;
#53677=CARTESIAN_POINT ( 'NONE',  ( 8.630000000000000782, 1.019547802438459216, 4.000000000000000000 ) ) ;
#53679=COLOUR_RGB ( '', 0.31764706, 0.68627451, 0.89019608) ;
#53694=CIRCLE ( 'NONE', #66397, 1.500000000000001332 ) ;
#53699=CARTESIAN_POINT ( 'NONE',  ( -3.949999999999997069, 99.99999999999998579, -8.525133428036873795 ) ) ;
#53703=CARTESIAN_POINT ( 'NONE',  ( -18.89999999999999147, 99.99999999999998579, 8.000000000000000000 ) ) ;
#53709=ADVANCED_FACE ( 'NONE', ( #27249 ), #34461, .T. ) ;
#53716=EDGE_CURVE ( 'NONE', #44632, #51712, #74221, .T. ) ;
#53731=CARTESIAN_POINT ( 'NONE',  ( 48.54513754358777788, 66.34502130956990129, -8.000000000000000000 ) ) ;
#53737=CARTESIAN_POINT ( 'NONE',  ( 10.34945593955694498, -32.01313548011169985, -3.750000000000000000 ) ) ;
#53752=ORIENTED_EDGE ( 'NONE', *, *, #23064, .F. ) ;
#53768=SPHERICAL_SURFACE ( 'NONE', #68567, 0.2500000000000000000 ) ;
#53771=EDGE_LOOP ( 'NONE', ( #7817, #21704, #36183 ) ) ;
#53779=VERTEX_POINT ( 'NONE', #53216 ) ;
#53786=( LENGTH_UNIT ( ) NAMED_UNIT ( * ) SI_UNIT ( .MILLI., .METRE. ) );
#53798=ORIENTED_EDGE ( 'NONE', *, *, #97214, .T. ) ;
#53803=LINE ( 'NONE', #84314, #35623 ) ;
#53813=CARTESIAN_POINT ( 'NONE',  ( -3.499999999999998668, 1.019547802438465434, -2.750000000000000444 ) ) ;
#53824=CARTESIAN_POINT ( 'NONE',  ( 6.757497259963602509, -58.30388498733370284, -2.500000000000000000 ) ) ;
#53828=DIRECTION ( 'NONE',  ( -0.06975647374410356982, -0.9975640502598257520, -0.000000000000000000 ) ) ;
#53838=PRESENTATION_STYLE_ASSIGNMENT (( #91336 ) ) ;
#53842=CARTESIAN_POINT ( 'NONE',  ( -10.07341714981312109, -32.14978703225555989, -3.750000000000000000 ) ) ;
#53846=( NAMED_UNIT ( * ) SI_UNIT ( $, .STERADIAN. ) SOLID_ANGLE_UNIT ( ) );
#53867=CARTESIAN_POINT ( 'NONE',  ( 17.75000000000001776, 4.561680251642721935E-15, -6.250000000000000000 ) ) ;
#53877=AXIS2_PLACEMENT_3D ( 'NONE', #27356, #20854, #76193 ) ;
#53891=ORIENTED_EDGE ( 'NONE', *, *, #42921, .F. ) ;
#53898=CARTESIAN_POINT ( 'NONE',  ( 6.829574850505124139, -88.00372650098208283, 4.000000000000000000 ) ) ;
#53903=CARTESIAN_POINT ( 'NONE',  ( -7.374944882893555764, -78.83129233208414632, -4.000000000000000888 ) ) ;
#53930=CARTESIAN_POINT ( 'NONE',  ( -7.750000000000000000, 79.82179676972448590, 6.250000000000000000 ) ) ;
#53932=VECTOR ( 'NONE', #27018, 1000.000000000000000 ) ;
#53937=CIRCLE ( 'NONE', #39605, 0.2500000000000002220 ) ;
#53962=EDGE_LOOP ( 'NONE', ( #86090, #71394, #10388, #24778 ) ) ;
#53984=ADVANCED_FACE ( 'NONE', ( #74728 ), #75718, .F. ) ;
#53992=FILL_AREA_STYLE ('',( #61486 ) ) ;
#54001=CARTESIAN_POINT ( 'NONE',  ( -19.64999999999999858, 98.99999999999998579, -7.750000000000000000 ) ) ;
#54005=CARTESIAN_POINT ( 'NONE',  ( -4.511928667086301914, -13.83795187542450122, -4.000000000000000888 ) ) ;
#54006=CIRCLE ( 'NONE', #28454, 0.09999999999999982514 ) ;
#54014=CARTESIAN_POINT ( 'NONE',  ( -8.223478179881800187, 85.80780507572961824, -3.936430718245989002 ) ) ;
#54030=EDGE_CURVE ( 'NONE', #34483, #105, #88707, .T. ) ;
#54048=STYLED_ITEM ( 'NONE', ( #69891 ), #16638 ) ;
#54057=DIRECTION ( 'NONE',  ( 1.000000000000000000, 0.000000000000000000, 0.000000000000000000 ) ) ;
#54068=ORIENTED_EDGE ( 'NONE', *, *, #91988, .F. ) ;
#54078=CARTESIAN_POINT ( 'NONE',  ( -3.749999999999988010, -5.564482262735336175E-16, -4.000000000000000000 ) ) ;
#54088=( LENGTH_UNIT ( ) NAMED_UNIT ( * ) SI_UNIT ( .MILLI., .METRE. ) );
#54107=SPHERICAL_SURFACE ( 'NONE', #84143, 0.2500000000000000000 ) ;
#54112=VERTEX_POINT ( 'NONE', #54675 ) ;
#54113=ORIENTED_EDGE ( 'NONE', *, *, #70780, .T. ) ;
#54119=CARTESIAN_POINT ( 'NONE',  ( -11.30179204364036849, -57.06033576790798634, 3.750000000000000000 ) ) ;
#54125=LINE ( 'NONE', #86118, #61917 ) ;
#54131=FACE_OUTER_BOUND ( 'NONE', #64595, .T. ) ;
#54141=EDGE_CURVE ( 'NONE', #51203, #60398, #10671, .T. ) ;
#54145=EDGE_LOOP ( 'NONE', ( #60776, #71626, #3301, #86039 ) ) ;
#54157=DIRECTION ( 'NONE',  ( -0.000000000000000000, -0.000000000000000000, 1.000000000000000000 ) ) ;
#54158=CARTESIAN_POINT ( 'NONE',  ( -8.000000000000000000, 80.32179676972448590, -3.750000000000000000 ) ) ;
#54162=( NAMED_UNIT ( * ) SI_UNIT ( $, .STERADIAN. ) SOLID_ANGLE_UNIT ( ) );
#54169=CARTESIAN_POINT ( 'NONE',  ( 6.879999999999995453, 43.00000000000000000, 6.500000000000000888 ) ) ;
#54174=SURFACE_STYLE_USAGE ( .BOTH. , #86166 ) ;
#54210=SURFACE_STYLE_FILL_AREA ( #23255 ) ;
#54215=EDGE_LOOP ( 'NONE', ( #56683, #96586, #35585, #78119 ) ) ;
#54218=CARTESIAN_POINT ( 'NONE',  ( 8.900267061460978013, -1.043551099215020317, -3.750000000000000000 ) ) ;
#54227=DIRECTION ( 'NONE',  ( -1.000000000000000000, 0.000000000000000000, 0.000000000000000000 ) ) ;
#54233=ADVANCED_FACE ( 'NONE', ( #73119 ), #96146, .T. ) ;
#54235=ORIENTED_EDGE ( 'NONE', *, *, #94864, .T. ) ;
#54237=CARTESIAN_POINT ( 'NONE',  ( -8.000000000000001776, -7.313785530895824394, 3.750000000000000000 ) ) ;
#54247=CARTESIAN_POINT ( 'NONE',  ( 18.00000000000000000, 78.50170875364594281, 3.769097879697934861 ) ) ;
#54250=CARTESIAN_POINT ( 'NONE',  ( -6.607869636406700664, -50.96183896326240159, 3.750000000001612044 ) ) ;
#54251=VERTEX_POINT ( 'NONE', #28122 ) ;
#54252=B_SPLINE_CURVE_WITH_KNOTS ( 'NONE', 3,
 ( #41076, #85585, #2604, #72045, #47075, #26067, #3574, #26543, #93565, #40581, #86571, #33057, #25098, #48552, #71078, #9581, #79053, #48057, #78571, #17098, #39603, #47581, #71573, #2109, #78077, #18563, #3084, #32063 ),
 .UNSPECIFIED., .F., .F.,
 ( 4, 2, 2, 2, 2, 2, 2, 2, 2, 2, 2, 2, 2, 4 ),
 ( 0.000000000000000000, 0.003117168999339133169, 0.006234337998678266338, 0.01246867599735653268, 0.02493735199471306535, 0.03740602799206958068, 0.04987470398942610988, 0.06234337998678262521, 0.07481205598413914748, 0.08728073198149567669, 0.09351506998017390659, 0.09663223897951304930, 0.09819082347918259290, 0.09974940797885215038 ),
 .UNSPECIFIED. ) ;
#54253=CARTESIAN_POINT ( 'NONE',  ( 3.969999999999999751, 0.000000000000000000, -2.500000000000000000 ) ) ;
#54260=ORIENTED_EDGE ( 'NONE', *, *, #43268, .T. ) ;
#54267=CARTESIAN_POINT ( 'NONE',  ( -3.750000000000000000, 36.75000000000000000, 4.000000000000000000 ) ) ;
#54271=EDGE_CURVE ( 'NONE', #11027, #28677, #7302, .T. ) ;
#54275=DIRECTION ( 'NONE',  ( -0.06975647374412535795, -0.9975640502598243087, 0.000000000000000000 ) ) ;
#54281=AXIS2_PLACEMENT_3D ( 'NONE', #22393, #23875, #91362 ) ;
#54287=SURFACE_STYLE_FILL_AREA ( #21846 ) ;
#54288=CARTESIAN_POINT ( 'NONE',  ( -3.585811749738964771, -2.700663748499701367, -2.750000000000000888 ) ) ;
#54292=FILL_AREA_STYLE_COLOUR ( '', #95018 ) ;
#54301=( NAMED_UNIT ( * ) SI_UNIT ( $, .STERADIAN. ) SOLID_ANGLE_UNIT ( ) );
#54310=LINE ( 'NONE', #52837, #94135 ) ;
#54313=CARTESIAN_POINT ( 'NONE',  ( 18.00000000000000000, 78.80384757729335377, -3.750000000000000000 ) ) ;
#54316=CARTESIAN_POINT ( 'NONE',  ( -10.57486859796104994, -40.44919682093461688, -3.750000000000000000 ) ) ;
#54320=ORIENTED_EDGE ( 'NONE', *, *, #63452, .T. ) ;
#54323=DIRECTION ( 'NONE',  ( -0.000000000000000000, -0.000000000000000000, 1.000000000000000000 ) ) ;
#54324=DIRECTION ( 'NONE',  ( 0.000000000000000000, -1.000000000000000000, 0.000000000000000000 ) ) ;
#54332=LINE ( 'NONE', #92830, #67639 ) ;
#54341=DIRECTION ( 'NONE',  ( 0.000000000000000000, 0.000000000000000000, 1.000000000000000000 ) ) ;
#54346=SURFACE_STYLE_USAGE ( .BOTH. , #47333 ) ;
#54350=UNCERTAINTY_MEASURE_WITH_UNIT (LENGTH_MEASURE( 1.000000000000000082E-05 ), #21620, 'distance_accuracy_value', 'NONE');
#54354=DIRECTION ( 'NONE',  ( -0.000000000000000000, 0.000000000000000000, -1.000000000000000000 ) ) ;
#54374=CARTESIAN_POINT ( 'NONE',  ( 14.99999999999997691, 80.32179676972448590, -4.250000000000000000 ) ) ;
#54379=DIRECTION ( 'NONE',  ( 0.000000000000000000, 0.000000000000000000, -1.000000000000000000 ) ) ;
#54388=CARTESIAN_POINT ( 'NONE',  ( 15.00000000000000178, 73.00000000000000000, 6.500000000000000888 ) ) ;
#54396=ORIENTED_EDGE ( 'NONE', *, *, #74093, .F. ) ;
#54411=CARTESIAN_POINT ( 'NONE',  ( 7.184033521041851778, -73.16344059793529198, -4.000000000000002665 ) ) ;
#54416=EDGE_CURVE ( 'NONE', #79731, #20729, #46115, .T. ) ;
#54429=CARTESIAN_POINT ( 'NONE',  ( 5.510795456469524289, -25.29786701974074603, -3.750000000000000888 ) ) ;
#54430=CARTESIAN_POINT ( 'NONE',  ( 4.471066085428756942, -3.611416924335026479, 2.750000000000000000 ) ) ;
#54449=SURFACE_SIDE_STYLE ('',( #62436 ) ) ;
#54463=AXIS2_PLACEMENT_3D ( 'NONE', #9823, #40325, #71313 ) ;
#54468=CIRCLE ( 'NONE', #36929, 0.2500000000000002220 ) ;
#54473=LINE ( 'NONE', #69004, #38461 ) ;
#54485=CARTESIAN_POINT ( 'NONE',  ( 0.000000000000000000, 99.99999999999998579, 8.000000000000000000 ) ) ;
#54502=( GEOMETRIC_REPRESENTATION_CONTEXT ( 3 ) GLOBAL_UNCERTAINTY_ASSIGNED_CONTEXT ( ( #90372 ) ) GLOBAL_UNIT_ASSIGNED_CONTEXT ( ( #73522, #49067, #49541 ) ) REPRESENTATION_CONTEXT ( 'NONE', 'WORKASPACE' ) );
#54521=EDGE_LOOP ( 'NONE', ( #905, #7911, #50594, #29968 ) ) ;
#54529=( GEOMETRIC_REPRESENTATION_CONTEXT ( 3 ) GLOBAL_UNCERTAINTY_ASSIGNED_CONTEXT ( ( #96504 ) ) GLOBAL_UNIT_ASSIGNED_CONTEXT ( ( #80794, #35779, #27285 ) ) REPRESENTATION_CONTEXT ( 'NONE', 'WORKASPACE' ) );
#54530=EDGE_CURVE ( 'NONE', #32093, #44664, #10572, .T. ) ;
#54532=ORIENTED_EDGE ( 'NONE', *, *, #8840, .F. ) ;
#54533=ORIENTED_EDGE ( 'NONE', *, *, #32843, .F. ) ;
#54551=AXIS2_PLACEMENT_3D ( 'NONE', #94062, #1614, #63065 ) ;
#54555=ORIENTED_EDGE ( 'NONE', *, *, #92397, .F. ) ;
#54560=CIRCLE ( 'NONE', #49778, 0.5000000000000000000 ) ;
#54562=CARTESIAN_POINT ( 'NONE',  ( -6.841090228438033272, -58.65898919720570603, -3.750000000000000000 ) ) ;
#54564=DIRECTION ( 'NONE',  ( 0.000000000000000000, 0.000000000000000000, -1.000000000000000000 ) ) ;
#54576=PRESENTATION_STYLE_ASSIGNMENT (( #62074 ) ) ;
#54586=ORIENTED_EDGE ( 'NONE', *, *, #94487, .T. ) ;
#54599=EDGE_LOOP ( 'NONE', ( #96498, #58451, #35270, #679 ) ) ;
#54600=CIRCLE ( 'NONE', #72160, 0.2500000000000002220 ) ;
#54605=CARTESIAN_POINT ( 'NONE',  ( -10.79671963678341484, -44.59934526487723616, 3.750000000000000000 ) ) ;
#54617=VERTEX_POINT ( 'NONE', #33062 ) ;
#54627=EDGE_CURVE ( 'NONE', #32382, #18106, #85094, .T. ) ;
#54640=COLOUR_RGB ( '', 0.09019608, 0.27058824, 0.51372549) ;
#54646=EDGE_CURVE ( 'NONE', #38899, #96234, #12124, .T. ) ;
#54647=CARTESIAN_POINT ( 'NONE',  ( -6.732636091893173358, -88.11213685669365248, 2.750000000000000000 ) ) ;
#54649=CARTESIAN_POINT ( 'NONE',  ( 9.112672642476784546, -7.236390792806629335, 4.000000000000000000 ) ) ;
#54655=DIRECTION ( 'NONE',  ( 0.000000000000000000, 0.000000000000000000, -1.000000000000000000 ) ) ;
#54656=ORIENTED_EDGE ( 'NONE', *, *, #96782, .T. ) ;
#54675=CARTESIAN_POINT ( 'NONE',  ( -6.982525766850298687, -88.11956318484570261, -2.750000000000000444 ) ) ;
#54679=LINE ( 'NONE', #77683, #16909 ) ;
#54698=DIRECTION ( 'NONE',  ( -0.000000000000000000, 0.000000000000000000, 1.000000000000000000 ) ) ;
#54720=DIRECTION ( 'NONE',  ( -1.000000000000000000, -0.000000000000000000, -0.000000000000000000 ) ) ;
#54721=CARTESIAN_POINT ( 'NONE',  ( -11.88139889192316900, -91.33459011216928047, -3.750000000000000000 ) ) ;
#54732=DIRECTION ( 'NONE',  ( 0.5901017155109078427, 0.8073289077885689169, 0.000000000000000000 ) ) ;
#54736=CARTESIAN_POINT ( 'NONE',  ( -7.037696229836970296, -86.26312365674226612, 4.000000000000000000 ) ) ;
#54740=ORIENTED_EDGE ( 'NONE', *, *, #2891, .T. ) ;
#54744=SURFACE_STYLE_USAGE ( .BOTH. , #69772 ) ;
#54753=VERTEX_POINT ( 'NONE', #42068 ) ;
#54755=FILL_AREA_STYLE_COLOUR ( '', #78076 ) ;
#54759=DIRECTION ( 'NONE',  ( -0.000000000000000000, 0.000000000000000000, 1.000000000000000000 ) ) ;
#54765=LINE ( 'NONE', #2300, #19634 ) ;
#54773=CARTESIAN_POINT ( 'NONE',  ( -3.750000000000000000, 36.75000000000000000, 2.750000000000000000 ) ) ;
#54778=( GEOMETRIC_REPRESENTATION_CONTEXT ( 3 ) GLOBAL_UNCERTAINTY_ASSIGNED_CONTEXT ( ( #12275 ) ) GLOBAL_UNIT_ASSIGNED_CONTEXT ( ( #83322, #71763, #40783 ) ) REPRESENTATION_CONTEXT ( 'NONE', 'WORKASPACE' ) );
#54789=CARTESIAN_POINT ( 'NONE',  ( -4.000000000000000000, 78.07179676972445748, 4.250000000000000000 ) ) ;
#54805=PRESENTATION_STYLE_ASSIGNMENT (( #31320 ) ) ;
#54807=CIRCLE ( 'NONE', #67613, 3.750000000000001776 ) ;
#54821=ORIENTED_EDGE ( 'NONE', *, *, #45617, .F. ) ;
#54822=FACE_OUTER_BOUND ( 'NONE', #81188, .T. ) ;
#54830=DIRECTION ( 'NONE',  ( -6.938893903907222067E-15, 0.000000000000000000, 1.000000000000000000 ) ) ;
#54839=VECTOR ( 'NONE', #7875, 1000.000000000000000 ) ;
#54842=CARTESIAN_POINT ( 'NONE',  ( -4.250000000000000000, 78.07179676972445748, -6.250000000000000000 ) ) ;
#54850=AXIS2_PLACEMENT_3D ( 'NONE', #92968, #40484, #2004 ) ;
#54859=ADVANCED_FACE ( 'NONE', ( #49059 ), #1119, .T. ) ;
#54866=SURFACE_STYLE_FILL_AREA ( #30891 ) ;
#54871=CARTESIAN_POINT ( 'NONE',  ( -7.330068351210572430, -69.53589943318687006, -4.000000000000000888 ) ) ;
#54880=DIRECTION ( 'NONE',  ( 0.000000000000000000, 0.000000000000000000, 1.000000000000000000 ) ) ;
#54884=VERTEX_POINT ( 'NONE', #18567 ) ;
#54894=CARTESIAN_POINT ( 'NONE',  ( -8.160053284515589311, -4.177241847651679052, 3.750000000000001332 ) ) ;
#54898=DIRECTION ( 'NONE',  ( -0.000000000000000000, 1.000000000000000000, -0.000000000000000000 ) ) ;
#54901=PLANE ( 'NONE',  #82486 ) ;
#54906=CIRCLE ( 'NONE', #82041, 0.2500000000000002220 ) ;
#54908=CARTESIAN_POINT ( 'NONE',  ( 4.380000000000002558, 1.019547802438462547, -2.750000000000000000 ) ) ;
#54912=( GEOMETRIC_REPRESENTATION_CONTEXT ( 3 ) GLOBAL_UNCERTAINTY_ASSIGNED_CONTEXT ( ( #26506 ) ) GLOBAL_UNIT_ASSIGNED_CONTEXT ( ( #91207, #23233, #14243 ) ) REPRESENTATION_CONTEXT ( 'NONE', 'WORKASPACE' ) );
#54917=CARTESIAN_POINT ( 'NONE',  ( -5.999999999999994671, 79.82179676972448590, -6.500000000000000888 ) ) ;
#54918=CARTESIAN_POINT ( 'NONE',  ( 4.572805491842157011, -6.390838093384605401, 2.500000000000000000 ) ) ;
#54936=FILL_AREA_STYLE_COLOUR ( '', #16158 ) ;
#54962=CARTESIAN_POINT ( 'NONE',  ( 9.879999999999990123, 20.99999999999999645, -3.000000000000000000 ) ) ;
#54963=CARTESIAN_POINT ( 'NONE',  ( -3.499999999999998668, 1.019547802438465434, 2.750000000000000444 ) ) ;
#54970=CYLINDRICAL_SURFACE ( 'NONE', #71436, 4.000000000000001776 ) ;
#54975=DIRECTION ( 'NONE',  ( -0.000000000000000000, -0.000000000000000000, 1.000000000000000000 ) ) ;
#54976=EDGE_LOOP ( 'NONE', ( #528, #10690, #73050, #64619 ) ) ;
#54977=ORIENTED_EDGE ( 'NONE', *, *, #29682, .F. ) ;
#54992=VECTOR ( 'NONE', #85576, 1000.000000000000000 ) ;
#55004=EDGE_CURVE ( 'NONE', #74689, #35385, #91741, .T. ) ;
#55007=ORIENTED_EDGE ( 'NONE', *, *, #56544, .F. ) ;
#55012=VERTEX_POINT ( 'NONE', #83238 ) ;
#55018=FACE_OUTER_BOUND ( 'NONE', #15857, .T. ) ;
#55026=ORIENTED_EDGE ( 'NONE', *, *, #80701, .T. ) ;
#55032=CYLINDRICAL_SURFACE ( 'NONE', #31070, 0.2500000000000002220 ) ;
#55036=CARTESIAN_POINT ( 'NONE',  ( -8.900000000000002132, 80.99999999999994316, 0.000000000000000000 ) ) ;
#55057=( NAMED_UNIT ( * ) PLANE_ANGLE_UNIT ( ) SI_UNIT ( $, .RADIAN. ) );
#55063=DIRECTION ( 'NONE',  ( 1.000000000000000000, 0.000000000000000000, 0.000000000000000000 ) ) ;
#55065=CARTESIAN_POINT ( 'NONE',  ( -10.20000000000000107, 43.92361346574197256, 3.000000000000000000 ) ) ;
#55072=CIRCLE ( 'NONE', #47081, 0.2500000000000002220 ) ;
#55073=( NAMED_UNIT ( * ) PLANE_ANGLE_UNIT ( ) SI_UNIT ( $, .RADIAN. ) );
#55082=DIRECTION ( 'NONE',  ( 0.000000000000000000, 0.000000000000000000, 1.000000000000000000 ) ) ;
#55091=( NAMED_UNIT ( * ) PLANE_ANGLE_UNIT ( ) SI_UNIT ( $, .RADIAN. ) );
#55092=CARTESIAN_POINT ( 'NONE',  ( 4.469999999999999751, 10.25000000000000000, 4.000000000000000000 ) ) ;
#55099=CARTESIAN_POINT ( 'NONE',  ( 17.75000000000000355, 77.07179676972445748, -6.500000000000000888 ) ) ;
#55105=CARTESIAN_POINT ( 'NONE',  ( -0.5000000000000073275, 80.99999999999994316, 1.249999999999987121 ) ) ;
#55108=VERTEX_POINT ( 'NONE', #16739 ) ;
#55140=CARTESIAN_POINT ( 'NONE',  ( -4.818768077838453401, -24.96217769840858125, 2.500000000000000888 ) ) ;
#55142=DIRECTION ( 'NONE',  ( 1.000000000000000000, 0.000000000000000000, 0.000000000000000000 ) ) ;
#55150=DIRECTION ( 'NONE',  ( 1.000000000000000000, -0.000000000000000000, -0.000000000000000000 ) ) ;
#55158=AXIS2_PLACEMENT_3D ( 'NONE', #57747, #5754, #19758 ) ;
#55162=AXIS2_PLACEMENT_3D ( 'NONE', #37762, #46712, #44743 ) ;
#55169=DIRECTION ( 'NONE',  ( 1.000000000000000000, 0.000000000000000000, -0.000000000000000000 ) ) ;
#55203=CARTESIAN_POINT ( 'NONE',  ( 9.209312257404453916, -9.300771453418956725, -4.000000000000000000 ) ) ;
#55214=EDGE_LOOP ( 'NONE', ( #76555, #94965, #3219, #94614 ) ) ;
#55231=CARTESIAN_POINT ( 'NONE',  ( -8.000000000000000000, 79.82179676972448590, 6.500000000000000888 ) ) ;
#55235=CARTESIAN_POINT ( 'NONE',  ( -7.121448108955550360, -73.25984652122872376, 4.000000000000000888 ) ) ;
#55236=VERTEX_POINT ( 'NONE', #51162 ) ;
#55240=ORIENTED_EDGE ( 'NONE', *, *, #22608, .F. ) ;
#55245=DIRECTION ( 'NONE',  ( -0.000000000000000000, 0.000000000000000000, 1.000000000000000000 ) ) ;
#55259=CARTESIAN_POINT ( 'NONE',  ( 8.879999999999991900, 21.00000000000000000, 2.899999999999999911 ) ) ;
#55279=CYLINDRICAL_SURFACE ( 'NONE', #81980, 0.2500000000000002220 ) ;
#55280=CARTESIAN_POINT ( 'NONE',  ( -5.810136766783611684, -36.09274195109910721, -2.750000000000000444 ) ) ;
#55283=DIRECTION ( 'NONE',  ( 0.000000000000000000, -0.000000000000000000, -1.000000000000000000 ) ) ;
#55289=CARTESIAN_POINT ( 'NONE',  ( -9.093709202272499681, 88.10000367580643399, 5.077063215882387404 ) ) ;
#55293=DIRECTION ( 'NONE',  ( -1.000000000000000000, 0.000000000000000000, -0.000000000000000000 ) ) ;
#55315=ADVANCED_FACE ( 'NONE', ( #19185 ), #13846, .F. ) ;
#55327=CARTESIAN_POINT ( 'NONE',  ( -8.000000000000000000, 0.000000000000000000, 6.250000000000000000 ) ) ;
#55332=CARTESIAN_POINT ( 'NONE',  ( -4.000000000000000000, 36.75000000000000000, -2.750000000000000000 ) ) ;
#55333=DIRECTION ( 'NONE',  ( 0.000000000000000000, 0.000000000000000000, 1.000000000000000000 ) ) ;
#55335=CARTESIAN_POINT ( 'NONE',  ( 14.99999999999998224, 70.25000000000000000, 6.250000000000000000 ) ) ;
#55338=FACE_OUTER_BOUND ( 'NONE', #68072, .T. ) ;
#55344=UNCERTAINTY_MEASURE_WITH_UNIT (LENGTH_MEASURE( 1.000000000000000082E-05 ), #13017, 'distance_accuracy_value', 'NONE');
#55349=PLANE ( 'NONE',  #53383 ) ;
#55370=AXIS2_PLACEMENT_3D ( 'NONE', #3640, #72114, #64596 ) ;
#55378=ORIENTED_EDGE ( 'NONE', *, *, #23068, .F. ) ;
#55383=ORIENTED_EDGE ( 'NONE', *, *, #98365, .F. ) ;
#55406=FACE_OUTER_BOUND ( 'NONE', #33890, .T. ) ;
#55412=CIRCLE ( 'NONE', #34619, 0.2500000000000002220 ) ;
#55414=DIRECTION ( 'NONE',  ( 0.6246950475544237324, 0.7808688094430306093, 0.000000000000000000 ) ) ;
#55425=CARTESIAN_POINT ( 'NONE',  ( 18.00000000000000000, 84.07179676972448590, -3.750000000000000000 ) ) ;
#55430=VERTEX_POINT ( 'NONE', #82141 ) ;
#55440=CARTESIAN_POINT ( 'NONE',  ( -3.750000000000000000, 9.750000000000000000, -3.750000000000000000 ) ) ;
#55441=ADVANCED_FACE ( 'NONE', ( #65163 ), #50671, .F. ) ;
#55446=DIRECTION ( 'NONE',  ( 1.000000000000000000, 0.000000000000000000, 0.000000000000000000 ) ) ;
#55451=DIRECTION ( 'NONE',  ( 0.000000000000000000, 1.000000000000000000, 0.000000000000000000 ) ) ;
#55454=CARTESIAN_POINT ( 'NONE',  ( 4.219999999999999751, 10.00000000000000000, 2.500000000000000000 ) ) ;
#55455=DIRECTION ( 'NONE',  ( -2.107602052970794797E-16, 1.000000000000000000, 0.000000000000000000 ) ) ;
#55457=DIRECTION ( 'NONE',  ( 0.000000000000000000, 1.000000000000000000, -0.000000000000000000 ) ) ;
#55463=CARTESIAN_POINT ( 'NONE',  ( 4.629999999999990123, 76.07179676972444327, -4.250000000000000000 ) ) ;
#55464=VERTEX_POINT ( 'NONE', #58150 ) ;
#55501=CARTESIAN_POINT ( 'NONE',  ( -6.000000000000014211, 80.07179676972448590, -6.250000000000000000 ) ) ;
#55506=FILL_AREA_STYLE_COLOUR ( '', #20535 ) ;
#55510=VECTOR ( 'NONE', #21187, 1000.000000000000000 ) ;
#55519=AXIS2_PLACEMENT_3D ( 'NONE', #2921, #47891, #93892 ) ;
#55522=ORIENTED_EDGE ( 'NONE', *, *, #30160, .T. ) ;
#55529=EDGE_CURVE ( 'NONE', #1670, #1168, #2673, .T. ) ;
#55532=SURFACE_STYLE_USAGE ( .BOTH. , #56026 ) ;
#55533=ADVANCED_FACE ( 'NONE', ( #24166 ), #71985, .F. ) ;
#55539=DIRECTION ( 'NONE',  ( -1.000000000000000000, 0.000000000000000000, 0.000000000000000000 ) ) ;
#55550=DIRECTION ( 'NONE',  ( 1.000000000000000000, 0.000000000000000000, 0.000000000000000000 ) ) ;
#55557=CARTESIAN_POINT ( 'NONE',  ( -19.64999999999999858, 98.99999999999998579, 8.000000000000000000 ) ) ;
#55560=EDGE_CURVE ( 'NONE', #538, #37093, #79290, .T. ) ;
#55570=CARTESIAN_POINT ( 'NONE',  ( -7.750355510519348456, 84.07179676972448590, 4.000000000000000000 ) ) ;
#55572=CARTESIAN_POINT ( 'NONE',  ( 17.99999999999999645, 99.99999999999998579, -8.000000000000000000 ) ) ;
#55581=AXIS2_PLACEMENT_3D ( 'NONE', #93173, #12512, #35506 ) ;
#55582=DIRECTION ( 'NONE',  ( 0.000000000000000000, 1.000000000000000000, 0.000000000000000000 ) ) ;
#55593=DIRECTION ( 'NONE',  ( -1.000000000000000000, 0.000000000000000000, 0.000000000000000000 ) ) ;
#55599=DIRECTION ( 'NONE',  ( 1.000000000000000000, -3.469446951953623261E-15, -0.000000000000000000 ) ) ;
#55625=LINE ( 'NONE', #2651, #12594 ) ;
#55633=CARTESIAN_POINT ( 'NONE',  ( -10.53011945866294852, -98.59345040283277228, 4.000000000000000000 ) ) ;
#55638=VERTEX_POINT ( 'NONE', #11484 ) ;
#55649=AXIS2_PLACEMENT_3D ( 'NONE', #8262, #782, #14292 ) ;
#55652=ORIENTED_EDGE ( 'NONE', *, *, #12326, .T. ) ;
#55654=CARTESIAN_POINT ( 'NONE',  ( -4.535014064427665303, -17.52590857053631623, 2.500000000000806910 ) ) ;
#55656=( LENGTH_UNIT ( ) NAMED_UNIT ( * ) SI_UNIT ( .MILLI., .METRE. ) );
#55675=ORIENTED_EDGE ( 'NONE', *, *, #95309, .T. ) ;
#55684=DIRECTION ( 'NONE',  ( 0.000000000000000000, 0.000000000000000000, -1.000000000000000000 ) ) ;
#55713=FACE_OUTER_BOUND ( 'NONE', #10849, .T. ) ;
#55716=MECHANICAL_DESIGN_GEOMETRIC_PRESENTATION_REPRESENTATION('',(#22173),#4619);
#55721=DIRECTION ( 'NONE',  ( -1.000000000000000000, 0.000000000000000000, 0.000000000000000000 ) ) ;
#55725=EDGE_LOOP ( 'NONE', ( #66783, #15542, #76656, #30082 ) ) ;
#55726=CIRCLE ( 'NONE', #10965, 0.5000000000000000000 ) ;
#55730=CARTESIAN_POINT ( 'NONE',  ( -4.000000000000000000, 10.00000000000000000, -2.750000000000000000 ) ) ;
#55732=PRESENTATION_STYLE_ASSIGNMENT (( #2256 ) ) ;
#55736=CARTESIAN_POINT ( 'NONE',  ( -6.000000000000011546, 40.74999999999999289, -4.250000000000000000 ) ) ;
#55742=LINE ( 'NONE', #62235, #43403 ) ;
#55743=FACE_OUTER_BOUND ( 'NONE', #29242, .T. ) ;
#55746=CARTESIAN_POINT ( 'NONE',  ( -4.262581422817185661, -13.85606188144532958, 3.999999999998386624 ) ) ;
#55755=DIRECTION ( 'NONE',  ( 1.000000000000000000, 0.000000000000000000, 0.000000000000000000 ) ) ;
#55756=VERTEX_POINT ( 'NONE', #69560 ) ;
#55759=VERTEX_POINT ( 'NONE', #30555 ) ;
#55765=( GEOMETRIC_REPRESENTATION_CONTEXT ( 3 ) GLOBAL_UNCERTAINTY_ASSIGNED_CONTEXT ( ( #41210 ) ) GLOBAL_UNIT_ASSIGNED_CONTEXT ( ( #45625, #82634, #44127 ) ) REPRESENTATION_CONTEXT ( 'NONE', 'WORKASPACE' ) );
#55768=DIRECTION ( 'NONE',  ( 0.000000000000000000, 0.000000000000000000, 1.000000000000000000 ) ) ;
#55774=DIRECTION ( 'NONE',  ( -0.000000000000000000, 0.000000000000000000, 1.000000000000000000 ) ) ;
#55785=CARTESIAN_POINT ( 'NONE',  ( 0.000000000000000000, 80.32179676972448590, -4.250000000000000000 ) ) ;
#55790=AXIS2_PLACEMENT_3D ( 'NONE', #25517, #39034, #62997 ) ;
#55801=CARTESIAN_POINT ( 'NONE',  ( 4.573260519722770034, -6.401749983361684215, 2.750000000000000444 ) ) ;
#55817=ORIENTED_EDGE ( 'NONE', *, *, #56101, .F. ) ;
#55821=CARTESIAN_POINT ( 'NONE',  ( -8.331109669465192269, 86.16998870897720053, -4.268594137767635743 ) ) ;
#55836=CARTESIAN_POINT ( 'NONE',  ( 10.88670032895693218, -94.01435490391448013, -3.999999999999999112 ) ) ;
#55839=LINE ( 'NONE', #48320, #12347 ) ;
#55840=FILL_AREA_STYLE ('',( #9346 ) ) ;
#55843=EDGE_CURVE ( 'NONE', #92042, #5883, #61773, .T. ) ;
#55850=FACE_OUTER_BOUND ( 'NONE', #64109, .T. ) ;
#55858=EDGE_CURVE ( 'NONE', #56730, #74593, #62036, .T. ) ;
#55866=ORIENTED_EDGE ( 'NONE', *, *, #22376, .F. ) ;
#55867=DIRECTION ( 'NONE',  ( -0.000000000000000000, 1.000000000000000000, -0.000000000000000000 ) ) ;
#55877=CIRCLE ( 'NONE', #33442, 0.2500000000000002220 ) ;
#55879=ORIENTED_EDGE ( 'NONE', *, *, #63120, .F. ) ;
#55886=CIRCLE ( 'NONE', #30, 1.750000000000000666 ) ;
#55896=VERTEX_POINT ( 'NONE', #23087 ) ;
#55901=CARTESIAN_POINT ( 'NONE',  ( -11.30270631010403726, -57.08945084610907372, 3.750000000000001776 ) ) ;
#55905=CARTESIAN_POINT ( 'NONE',  ( 4.879999999999994564, 43.00000000000000711, 6.500000000000000888 ) ) ;
#55910=DIRECTION ( 'NONE',  ( 1.000000000000000000, 2.569960705150826877E-16, -0.000000000000000000 ) ) ;
#55918=CARTESIAN_POINT ( 'NONE',  ( 12.99999999999999822, 75.00000000000000000, -6.500000000000000888 ) ) ;
#55926=CARTESIAN_POINT ( 'NONE',  ( 6.655516370397832837, -69.44235516224610194, 2.500000000000000000 ) ) ;
#55931=CARTESIAN_POINT ( 'NONE',  ( 8.629999999999995453, 40.99999999999999289, 4.250000000000000000 ) ) ;
#55937=AXIS2_PLACEMENT_3D ( 'NONE', #32208, #1753, #55721 ) ;
#55941=( NAMED_UNIT ( * ) PLANE_ANGLE_UNIT ( ) SI_UNIT ( $, .RADIAN. ) );
#55945=( LENGTH_UNIT ( ) NAMED_UNIT ( * ) SI_UNIT ( .MILLI., .METRE. ) );
#55964=LINE ( 'NONE', #70972, #67279 ) ;
#55972=ORIENTED_EDGE ( 'NONE', *, *, #64637, .F. ) ;
#55973=LINE ( 'NONE', #54962, #50077 ) ;
#55983=DIRECTION ( 'NONE',  ( 1.000000000000000000, 0.000000000000000000, 0.000000000000000000 ) ) ;
#56016=EDGE_CURVE ( 'NONE', #8937, #39745, #12320, .T. ) ;
#56020=CIRCLE ( 'NONE', #20897, 0.2500000000000002220 ) ;
#56023=CIRCLE ( 'NONE', #51219, 0.2500000000000002220 ) ;
#56026=SURFACE_SIDE_STYLE ('',( #78518 ) ) ;
#56037=LINE ( 'NONE', #63519, #77764 ) ;
#56040=EDGE_CURVE ( 'NONE', #44664, #98330, #56037, .T. ) ;
#56043=CYLINDRICAL_SURFACE ( 'NONE', #18742, 0.2500000000000002220 ) ;
#56046=FACE_OUTER_BOUND ( 'NONE', #23570, .T. ) ;
#56053=LINE ( 'NONE', #48528, #31443 ) ;
#56057=VECTOR ( 'NONE', #16966, 1000.000000000000114 ) ;
#56074=CARTESIAN_POINT ( 'NONE',  ( -10.82625193755174742, -96.00405735513187722, -4.000000000000000000 ) ) ;
#56075=PLANE ( 'NONE',  #97708 ) ;
#56085=CARTESIAN_POINT ( 'NONE',  ( -7.072473351904092986, -84.40137333043811907, -3.750000000000000444 ) ) ;
#56086=SURFACE_STYLE_FILL_AREA ( #25594 ) ;
#56089=ORIENTED_EDGE ( 'NONE', *, *, #49798, .F. ) ;
#56101=EDGE_CURVE ( 'NONE', #53272, #31285, #87332, .T. ) ;
#56109=DIRECTION ( 'NONE',  ( 2.107602052970794797E-16, -1.000000000000000000, 0.000000000000000000 ) ) ;
#56120=FACE_OUTER_BOUND ( 'NONE', #94090, .T. ) ;
#56121=ADVANCED_FACE ( 'NONE', ( #94508 ), #18520, .T. ) ;
#56122=EDGE_LOOP ( 'NONE', ( #15787, #23555, #46232, #11487 ) ) ;
#56136=ORIENTED_EDGE ( 'NONE', *, *, #40124, .T. ) ;
#56145=AXIS2_PLACEMENT_3D ( 'NONE', #98049, #91512, #45510 ) ;
#56150=CARTESIAN_POINT ( 'NONE',  ( 11.20666413564172537, -56.81049121600104002, 4.000000000000000000 ) ) ;
#56159=CARTESIAN_POINT ( 'NONE',  ( -4.000000000000000000, 78.07179676972445748, 6.500000000000000888 ) ) ;
#56164=CIRCLE ( 'NONE', #60923, 0.2500000000000002220 ) ;
#56198=B_SPLINE_CURVE_WITH_KNOTS ( 'NONE', 3,
 ( #19765, #57756, #5277, #27256, #35754, #94777, #20266, #34253, #88259, #56779, #81254, #20761, #27752, #58236, #87274, #43251, #79778, #50250 ),
 .UNSPECIFIED., .F., .F.,
 ( 4, 2, 2, 2, 2, 2, 2, 2, 4 ),
 ( 2.775557561562891043E-17, 0.01113190067936639140, 0.02226380135873275504, 0.04452760271746546150, 0.06679140407619817144, 0.07792330475556452640, 0.08348925509524771083, 0.08627223026508930304, 0.08905520543493089525 ),
 .UNSPECIFIED. ) ;
#56207=CARTESIAN_POINT ( 'NONE',  ( 8.880000000000000782, 1.019547802438459216, -3.750000000000000000 ) ) ;
#56217=PRESENTATION_STYLE_ASSIGNMENT (( #19681 ) ) ;
#56233=DIRECTION ( 'NONE',  ( 0.000000000000000000, 0.000000000000000000, 1.000000000000000000 ) ) ;
#56237=STYLED_ITEM ( 'NONE', ( #28665 ), #90872 ) ;
#56239=CARTESIAN_POINT ( 'NONE',  ( 12.40504043596831885, 57.00871557427475977, -2.900000000000000799 ) ) ;
#56253=EDGE_CURVE ( 'NONE', #55896, #42155, #52222, .T. ) ;
#56260=PRODUCT_DEFINITION ( 'UNKNOWN', '', #88670, #37477 ) ;
#56269=DIRECTION ( 'NONE',  ( -0.000000000000000000, -1.000000000000000000, -0.000000000000000000 ) ) ;
#56288=CARTESIAN_POINT ( 'NONE',  ( -8.641261271118773735, 87.40425324006859853, 4.716577832614896160 ) ) ;
#56290=VECTOR ( 'NONE', #826, 999.9999999999998863 ) ;
#56291=ORIENTED_EDGE ( 'NONE', *, *, #40621, .F. ) ;
#56308=ORIENTED_EDGE ( 'NONE', *, *, #5536, .F. ) ;
#56312=CYLINDRICAL_SURFACE ( 'NONE', #78996, 0.2500000000000002220 ) ;
#56323=CIRCLE ( 'NONE', #61090, 1.000000000000000888 ) ;
#56335=ADVANCED_FACE ( 'NONE', ( #86533 ), #21911, .T. ) ;
#56337=AXIS2_PLACEMENT_3D ( 'NONE', #96859, #50843, #96362 ) ;
#56343=CARTESIAN_POINT ( 'NONE',  ( -10.09048698379360687, 46.92328126389585208, 2.899999999999999467 ) ) ;
#56368=AXIS2_PLACEMENT_3D ( 'NONE', #94033, #55550, #86050 ) ;
#56372=TOROIDAL_SURFACE ( 'NONE', #78769, 6.599999999999995204, 0.2500000000000000000 ) ;
#56394=CARTESIAN_POINT ( 'NONE',  ( -11.58473852101197998, -69.55955830444820265, 3.750000000000000444 ) ) ;
#56411=LINE ( 'NONE', #80384, #24888 ) ;
#56419=CARTESIAN_POINT ( 'NONE',  ( 6.829574850505125028, -88.00372650098204019, 2.750000000000000888 ) ) ;
#56424=CARTESIAN_POINT ( 'NONE',  ( -3.750000000000000000, 36.75000000000000000, 2.750000000000000000 ) ) ;
#56429=DIRECTION ( 'NONE',  ( 1.000000000000000000, 0.000000000000000000, 0.000000000000000000 ) ) ;
#56434=AXIS2_PLACEMENT_3D ( 'NONE', #39683, #22217, #93149 ) ;
#56454=UNCERTAINTY_MEASURE_WITH_UNIT (LENGTH_MEASURE( 1.000000000000000082E-05 ), #43913, 'distance_accuracy_value', 'NONE');
#56460=ORIENTED_EDGE ( 'NONE', *, *, #65647, .T. ) ;
#56472=EDGE_LOOP ( 'NONE', ( #12558, #65954, #75544, #97661 ) ) ;
#56479=CARTESIAN_POINT ( 'NONE',  ( 9.879999999999988347, 26.99999999999999645, 2.900000000000000355 ) ) ;
#56519=VERTEX_POINT ( 'NONE', #52960 ) ;
#56523=UNCERTAINTY_MEASURE_WITH_UNIT (LENGTH_MEASURE( 1.000000000000000082E-05 ), #17464, 'distance_accuracy_value', 'NONE');
#56544=EDGE_CURVE ( 'NONE', #18106, #63974, #14497, .T. ) ;
#56546=DIRECTION ( 'NONE',  ( 0.8070303256584298035, -0.5905099943842175847, 0.000000000000000000 ) ) ;
#56549=CARTESIAN_POINT ( 'NONE',  ( 9.879999999999991900, 20.99999999999999645, 0.000000000000000000 ) ) ;
#56562=CARTESIAN_POINT ( 'NONE',  ( 18.00000000000000000, 77.37581971779152923, -4.190584158844754548 ) ) ;
#56572=CARTESIAN_POINT ( 'NONE',  ( -6.867514897637334137, -58.37540146638243499, -3.750000000000000888 ) ) ;
#56578=AXIS2_PLACEMENT_3D ( 'NONE', #35516, #89016, #11537 ) ;
#56580=CARTESIAN_POINT ( 'NONE',  ( 3.969999999999999751, 37.25000000000000000, -4.000000000000000000 ) ) ;
#56588=DIRECTION ( 'NONE',  ( 1.000000000000000000, 0.000000000000000000, 0.000000000000000000 ) ) ;
#56590=ORIENTED_EDGE ( 'NONE', *, *, #72570, .F. ) ;
#56604=ORIENTED_EDGE ( 'NONE', *, *, #89557, .F. ) ;
#56613=AXIS2_PLACEMENT_3D ( 'NONE', #12304, #56819, #72792 ) ;
#56620=ORIENTED_EDGE ( 'NONE', *, *, #24297, .F. ) ;
#56623=( NAMED_UNIT ( * ) PLANE_ANGLE_UNIT ( ) SI_UNIT ( $, .RADIAN. ) );
#56625=ADVANCED_FACE ( 'NONE', ( #16945 ), #2459, .T. ) ;
#56629=ORIENTED_EDGE ( 'NONE', *, *, #71677, .F. ) ;
#56630=CARTESIAN_POINT ( 'NONE',  ( 9.729341964107060647, -19.62354698957123134, 3.750000000000000000 ) ) ;
#56642=ORIENTED_EDGE ( 'NONE', *, *, #45617, .T. ) ;
#56654=DIRECTION ( 'NONE',  ( 1.000000000000000000, 0.000000000000000000, 0.000000000000000000 ) ) ;
#56662=CARTESIAN_POINT ( 'NONE',  ( -8.107947183327409491, -3.126532598402040897, -3.750000000000000000 ) ) ;
#56666=CIRCLE ( 'NONE', #4013, 0.1000000000000001166 ) ;
#56683=ORIENTED_EDGE ( 'NONE', *, *, #36933, .F. ) ;
#56695=ORIENTED_EDGE ( 'NONE', *, *, #45407, .F. ) ;
#56696=CARTESIAN_POINT ( 'NONE',  ( 6.507517414235559627, -58.30789062360079100, 2.499999999999999556 ) ) ;
#56697=ORIENTED_EDGE ( 'NONE', *, *, #85182, .T. ) ;
#56712=CARTESIAN_POINT ( 'NONE',  ( 0.000000000000000000, 99.74999999999998579, 7.750000000000000000 ) ) ;
#56725=EDGE_CURVE ( 'NONE', #30576, #76841, #60288, .T. ) ;
#56728=TOROIDAL_SURFACE ( 'NONE', #87056, 3.750000000000001776, 0.2500000000000000000 ) ;
#56730=VERTEX_POINT ( 'NONE', #10399 ) ;
#56741=( NAMED_UNIT ( * ) SI_UNIT ( $, .STERADIAN. ) SOLID_ANGLE_UNIT ( ) );
#56748=EDGE_CURVE ( 'NONE', #76742, #49408, #41106, .T. ) ;
#56758=EDGE_CURVE ( 'NONE', #12076, #70662, #79419, .T. ) ;
#56764=CARTESIAN_POINT ( 'NONE',  ( -12.19495285927274431, 90.49761223356982498, 7.228801115472508698 ) ) ;
#56779=CARTESIAN_POINT ( 'NONE',  ( 5.114754712244249824, -17.52455492747532517, 3.750000000000000444 ) ) ;
#56780=DIRECTION ( 'NONE',  ( 0.000000000000000000, 0.000000000000000000, -1.000000000000000000 ) ) ;
#56783=CARTESIAN_POINT ( 'NONE',  ( -3.500000000000001776, 0.08936006763181135459, 2.750000000000000888 ) ) ;
#56788=CARTESIAN_POINT ( 'NONE',  ( -8.641261271118773735, 87.40425324006859853, -4.716577832614896160 ) ) ;
#56796=ORIENTED_EDGE ( 'NONE', *, *, #47002, .F. ) ;
#56797=FACE_OUTER_BOUND ( 'NONE', #28562, .T. ) ;
#56804=FACE_OUTER_BOUND ( 'NONE', #32164, .T. ) ;
#56806=DIRECTION ( 'NONE',  ( -1.000000000000000000, 6.938893903907221278E-15, -6.938893903907221278E-15 ) ) ;
#56808=SURFACE_STYLE_USAGE ( .BOTH. , #72778 ) ;
#56818=EDGE_CURVE ( 'NONE', #76742, #14585, #66637, .T. ) ;
#56819=DIRECTION ( 'NONE',  ( -0.000000000000000000, -1.000000000000000000, -0.000000000000000000 ) ) ;
#56829=EDGE_LOOP ( 'NONE', ( #49555, #41021 ) ) ;
#56869=CARTESIAN_POINT ( 'NONE',  ( -10.81543368776825886, -98.37186030702901007, 3.750000000000000444 ) ) ;
#56878=PRESENTATION_STYLE_ASSIGNMENT (( #93901 ) ) ;
#56884=COLOUR_RGB ( '', 0.09019608, 0.27058824, 0.51372549) ;
#56894=AXIS2_PLACEMENT_3D ( 'NONE', #43744, #67749, #74739 ) ;
#56902=EDGE_CURVE ( 'NONE', #34926, #69049, #76208, .T. ) ;
#56906=CARTESIAN_POINT ( 'NONE',  ( -3.887834249506515683, -8.254296980867451339, -2.499999999999195310 ) ) ;
#56913=CARTESIAN_POINT ( 'NONE',  ( 6.829574850505125028, -88.00372650098209704, -3.750000000000000000 ) ) ;
#56928=COLOUR_RGB ( '', 0.31764706, 0.68627451, 0.89019608) ;
#56935=ORIENTED_EDGE ( 'NONE', *, *, #96342, .F. ) ;
#56955=DIRECTION ( 'NONE',  ( -0.000000000000000000, -0.000000000000000000, 1.000000000000000000 ) ) ;
#56962=CARTESIAN_POINT ( 'NONE',  ( -11.62551083756942027, -75.79479195806536040, -3.750000000000000444 ) ) ;
#56974=AXIS2_PLACEMENT_3D ( 'NONE', #80116, #42140, #72605 ) ;
#56983=CARTESIAN_POINT ( 'NONE',  ( -5.559536763064313547, -36.09058695999160449, 2.499999999999999112 ) ) ;
#56994=EDGE_LOOP ( 'NONE', ( #3398, #35918, #93971, #40064 ) ) ;
#57008=PRESENTATION_STYLE_ASSIGNMENT (( #18044 ) ) ;
#57021=EDGE_CURVE ( 'NONE', #63243, #62370, #93756, .T. ) ;
#57023=( GEOMETRIC_REPRESENTATION_CONTEXT ( 3 ) GLOBAL_UNCERTAINTY_ASSIGNED_CONTEXT ( ( #69114 ) ) GLOBAL_UNIT_ASSIGNED_CONTEXT ( ( #57296, #4314, #3825 ) ) REPRESENTATION_CONTEXT ( 'NONE', 'WORKASPACE' ) );
#57030=CARTESIAN_POINT ( 'NONE',  ( -11.80960303780298126, 90.32667112043513669, 7.004222671090198027 ) ) ;
#57032=ADVANCED_FACE ( 'NONE', ( #3889 ), #52297, .F. ) ;
#57033=CARTESIAN_POINT ( 'NONE',  ( -6.356754967080490815, -50.93964766207073325, -2.500000000000000000 ) ) ;
#57036=( NAMED_UNIT ( * ) PLANE_ANGLE_UNIT ( ) SI_UNIT ( $, .RADIAN. ) );
#57043=CARTESIAN_POINT ( 'NONE',  ( 18.00000000000000000, 77.66934307245453795, -4.068269658013956125 ) ) ;
#57045=MECHANICAL_DESIGN_GEOMETRIC_PRESENTATION_REPRESENTATION('',(#44277),#93386);
#57069=CARTESIAN_POINT ( 'NONE',  ( -3.500000000000000444, 0.08393865084444233904, -3.750000000002423839 ) ) ;
#57070=CIRCLE ( 'NONE', #88980, 1.750000000000000666 ) ;
#57082=( NAMED_UNIT ( * ) SI_UNIT ( $, .STERADIAN. ) SOLID_ANGLE_UNIT ( ) );
#57083=ADVANCED_FACE ( 'NONE', ( #55406 ), #85909, .F. ) ;
#57086=CARTESIAN_POINT ( 'NONE',  ( 17.75000000000000000, 77.07179676972445748, 6.500000000000000888 ) ) ;
#57088=FILL_AREA_STYLE ('',( #88568 ) ) ;
#57110=CARTESIAN_POINT ( 'NONE',  ( 10.95672398092068711, -56.81605919578149155, 4.000000000000000000 ) ) ;
#57113=CARTESIAN_POINT ( 'NONE',  ( 4.879999999999991900, 76.07179676972444327, 6.500000000000000888 ) ) ;
#57115=CARTESIAN_POINT ( 'NONE',  ( -3.990799379706100325, -9.967613007074422882, 3.750000000000000444 ) ) ;
#57116=VECTOR ( 'NONE', #65682, 1000.000000000000000 ) ;
#57118=CARTESIAN_POINT ( 'NONE',  ( -3.771484213771641336, -6.414706846149704766, 3.750000000000001332 ) ) ;
#57125=ADVANCED_FACE ( 'NONE', ( #7209 ), #65042, .T. ) ;
#57126=DIRECTION ( 'NONE',  ( 0.000000000000000000, 0.000000000000000000, 1.000000000000000000 ) ) ;
#57129=COLOUR_RGB ( '', 0.08235294, 0.09019608, 0.10196078) ;
#57130=SURFACE_STYLE_USAGE ( .BOTH. , #49145 ) ;
#57133=AXIS2_PLACEMENT_3D ( 'NONE', #56712, #80697, #65679 ) ;
#57167=CARTESIAN_POINT ( 'NONE',  ( 4.474002695404426966, -3.767820133606233579, 2.750000000000000000 ) ) ;
#57180=ORIENTED_EDGE ( 'NONE', *, *, #14389, .F. ) ;
#57199=ORIENTED_EDGE ( 'NONE', *, *, #76248, .F. ) ;
#57206=DIRECTION ( 'NONE',  ( 0.000000000000000000, 0.000000000000000000, -1.000000000000000000 ) ) ;
#57259=AXIS2_PLACEMENT_3D ( 'NONE', #36349, #66844, #97364 ) ;
#57263=FILL_AREA_STYLE_COLOUR ( '', #50554 ) ;
#57266=AXIS2_PLACEMENT_3D ( 'NONE', #30142, #98192, #91150 ) ;
#57268=ADVANCED_FACE ( 'NONE', ( #50855 ), #35848, .T. ) ;
#57269=AXIS2_PLACEMENT_3D ( 'NONE', #68206, #14217, #44697 ) ;
#57273=CARTESIAN_POINT ( 'NONE',  ( -7.072473369627247486, -84.40137233605018707, 2.750000000000000000 ) ) ;
#57278=CARTESIAN_POINT ( 'NONE',  ( -9.247107438774047949, 88.00886336720424197, -5.024692236534948009 ) ) ;
#57296=( LENGTH_UNIT ( ) NAMED_UNIT ( * ) SI_UNIT ( .MILLI., .METRE. ) );
#57332=ORIENTED_EDGE ( 'NONE', *, *, #21963, .F. ) ;
#57335=COLOUR_RGB ( '', 0.31764706, 0.68627451, 0.89019608) ;
#57339=EDGE_CURVE ( 'NONE', #5309, #9323, #44293, .T. ) ;
#57346=AXIS2_PLACEMENT_3D ( 'NONE', #71152, #48137, #55142 ) ;
#57356=ORIENTED_EDGE ( 'NONE', *, *, #55843, .F. ) ;
#57361=DIRECTION ( 'NONE',  ( 1.000000000000000000, -0.000000000000000000, -0.000000000000000000 ) ) ;
#57377=CARTESIAN_POINT ( 'NONE',  ( -3.999999999999999112, 78.07179676972445748, 4.250000000000000000 ) ) ;
#57399=CARTESIAN_POINT ( 'NONE',  ( -5.079065453171176969, -28.67168118942974075, -2.500000000000000888 ) ) ;
#57407=CARTESIAN_POINT ( 'NONE',  ( 5.680373671027947324, -28.65980262291034819, -3.749999999996780353 ) ) ;
#57422=UNCERTAINTY_MEASURE_WITH_UNIT (LENGTH_MEASURE( 1.000000000000000082E-05 ), #29839, 'distance_accuracy_value', 'NONE');
#57443=EDGE_CURVE ( 'NONE', #16387, #29547, #23706, .T. ) ;
#57452=SURFACE_SIDE_STYLE ('',( #95460 ) ) ;
#57475=EDGE_CURVE ( 'NONE', #26330, #55756, #88975, .T. ) ;
#57486=DIRECTION ( 'NONE',  ( 0.000000000000000000, 0.000000000000000000, 1.000000000000000000 ) ) ;
#57490=LINE ( 'NONE', #11995, #21454 ) ;
#57492=ORIENTED_EDGE ( 'NONE', *, *, #5168, .T. ) ;
#57517=ORIENTED_EDGE ( 'NONE', *, *, #31500, .F. ) ;
#57518=CARTESIAN_POINT ( 'NONE',  ( -9.000000000000001776, 80.99999999999994316, -1.249999999999987121 ) ) ;
#57525=CARTESIAN_POINT ( 'NONE',  ( -3.377746357650261988, -3.629174488344641070, -2.499999999999998668 ) ) ;
#57535=CARTESIAN_POINT ( 'NONE',  ( 17.99999999999999645, 78.68095262111053501, -3.967704011867417613 ) ) ;
#57540=CARTESIAN_POINT ( 'NONE',  ( 8.979999999999991545, 21.00000000000000000, 3.000000000000000000 ) ) ;
#57563=CARTESIAN_POINT ( 'NONE',  ( -13.11254139118232231, 91.00000000000000000, 8.000000000000000000 ) ) ;
#57569=VECTOR ( 'NONE', #21400, 1000.000000000000000 ) ;
#57570=VECTOR ( 'NONE', #14532, 1000.000000000000000 ) ;
#57575=B_SPLINE_CURVE_WITH_KNOTS ( 'NONE', 3,
 ( #34516, #95537, #88519, #65009, #20523, #28512, #42057, #27025, #57033, #43021, #19534, #19047, #81018, #96535, #80533, #12031, #59006, #57525, #12519, #51008, #5528, #3567 ),
 .UNSPECIFIED., .F., .F.,
 ( 4, 2, 2, 2, 2, 2, 2, 2, 2, 2, 4 ),
 ( 0.000000000000000000, 0.005576344000565805654, 0.01115268800113161131, 0.02230537600226322262, 0.04461075200452644524, 0.05576344000565804093, 0.06691612800678964357, 0.07806881600792124620, 0.08364516000848705446, 0.08643333200876995859, 0.08922150400905284884 ),
 .UNSPECIFIED. ) ;
#57582=CARTESIAN_POINT ( 'NONE',  ( -6.000000000000009770, 41.24999999999999289, 6.500000000000000888 ) ) ;
#57586=VERTEX_POINT ( 'NONE', #63628 ) ;
#57591=VERTEX_POINT ( 'NONE', #16681 ) ;
#57602=CARTESIAN_POINT ( 'NONE',  ( 11.04397247079906030, -89.88416767672931940, 4.000000000000000000 ) ) ;
#57605=CARTESIAN_POINT ( 'NONE',  ( -6.445967608602039434, -48.01283281809150338, 3.750000000000000444 ) ) ;
#57606=ORIENTED_EDGE ( 'NONE', *, *, #66209, .T. ) ;
#57609=CARTESIAN_POINT ( 'NONE',  ( -3.628035180575734486, -3.629434796165400989, 3.750000000000000888 ) ) ;
#57610=SURFACE_STYLE_USAGE ( .BOTH. , #27111 ) ;
#57613=LINE ( 'NONE', #17674, #97785 ) ;
#57617=FILL_AREA_STYLE ('',( #49141 ) ) ;
#57620=EDGE_CURVE ( 'NONE', #57586, #67582, #47151, .T. ) ;
#57621=PRESENTATION_STYLE_ASSIGNMENT (( #57130 ) ) ;
#57625=CIRCLE ( 'NONE', #65612, 0.2500000000000002220 ) ;
#57626=EDGE_LOOP ( 'NONE', ( #39202, #48613, #77510, #3735 ) ) ;
#57631=TOROIDAL_SURFACE ( 'NONE', #48069, 0.5000000000000000000, 0.2500000000000000000 ) ;
#57633=DIRECTION ( 'NONE',  ( 1.000000000000000000, -0.000000000000000000, -0.000000000000000000 ) ) ;
#57634=DIRECTION ( 'NONE',  ( 0.000000000000000000, 1.000000000000000000, -0.000000000000000000 ) ) ;
#57635=DIRECTION ( 'NONE',  ( 0.8070303256584298035, -0.5905099943842175847, 0.000000000000000000 ) ) ;
#57636=CIRCLE ( 'NONE', #92761, 0.2500000000000002220 ) ;
#57637=CYLINDRICAL_SURFACE ( 'NONE', #21698, 0.2500000000000002220 ) ;
#57642=CARTESIAN_POINT ( 'NONE',  ( -10.91892017000252046, -97.58704351930606435, -3.999999999999996891 ) ) ;
#57644=DIRECTION ( 'NONE',  ( 1.000000000000000000, 0.000000000000000000, 0.000000000000000000 ) ) ;
#57646=FILL_AREA_STYLE_COLOUR ( '', #44923 ) ;
#57662=CARTESIAN_POINT ( 'NONE',  ( 17.75000000000000355, 73.00000000000001421, 6.250000000000000000 ) ) ;
#57666=DIRECTION ( 'NONE',  ( 0.000000000000000000, 0.000000000000000000, -1.000000000000000000 ) ) ;
#57672=CARTESIAN_POINT ( 'NONE',  ( 6.683977931330074895, -73.15273079441168136, 2.500000000000000000 ) ) ;
#57674=ORIENTED_EDGE ( 'NONE', *, *, #78891, .T. ) ;
#57675=EDGE_LOOP ( 'NONE', ( #21011, #78755, #86959, #66320 ) ) ;
#57676=AXIS2_PLACEMENT_3D ( 'NONE', #80530, #18550, #56546 ) ;
#57695=ORIENTED_EDGE ( 'NONE', *, *, #34928, .F. ) ;
#57706=ADVANCED_FACE ( 'NONE', ( #9666 ), #4249, .F. ) ;
#57713=CARTESIAN_POINT ( 'NONE',  ( -4.000000000000000000, 10.00000000000000000, -2.500000000000000000 ) ) ;
#57728=DIRECTION ( 'NONE',  ( 0.000000000000000000, 0.000000000000000000, 1.000000000000000000 ) ) ;
#57732=DIRECTION ( 'NONE',  ( -0.5901017155109078427, -0.8073289077885689169, 0.000000000000000000 ) ) ;
#57735=EDGE_CURVE ( 'NONE', #81929, #86010, #72118, .T. ) ;
#57747=CARTESIAN_POINT ( 'NONE',  ( 15.00000000000000000, 77.07179676972447169, 6.250000000000000000 ) ) ;
#57756=CARTESIAN_POINT ( 'NONE',  ( 6.910419567532135154, -84.29192550413311835, 3.750000000000001776 ) ) ;
#57762=CARTESIAN_POINT ( 'NONE',  ( -8.399999999999998579, 98.49999999999998579, -8.525133428036873795 ) ) ;
#57766=CARTESIAN_POINT ( 'NONE',  ( -3.750000000000000000, 10.00000000000000000, 2.750000000000000000 ) ) ;
#57769=AXIS2_PLACEMENT_3D ( 'NONE', #54374, #7429, #61384 ) ;
#57774=CARTESIAN_POINT ( 'NONE',  ( 9.879999999999988347, 26.99999999999999645, 2.900000000000000355 ) ) ;
#57783=DIRECTION ( 'NONE',  ( 0.000000000000000000, 0.000000000000000000, 1.000000000000000000 ) ) ;
#57792=DIRECTION ( 'NONE',  ( 0.000000000000000000, 1.000000000000000000, 0.000000000000000000 ) ) ;
#57798=ADVANCED_FACE ( 'NONE', ( #35095 ), #34602, .F. ) ;
#57808=ORIENTED_EDGE ( 'NONE', *, *, #51184, .F. ) ;
#57810=ORIENTED_EDGE ( 'NONE', *, *, #86392, .T. ) ;
#57813=ORIENTED_EDGE ( 'NONE', *, *, #92675, .F. ) ;
#57827=VERTEX_POINT ( 'NONE', #84705 ) ;
#57831=LINE ( 'NONE', #34334, #11191 ) ;
#57841=ORIENTED_EDGE ( 'NONE', *, *, #42717, .F. ) ;
#57842=CIRCLE ( 'NONE', #76993, 2.000000000000000000 ) ;
#57848=DIRECTION ( 'NONE',  ( 1.000000000000000000, 0.000000000000000000, 0.000000000000000000 ) ) ;
#57855=ORIENTED_EDGE ( 'NONE', *, *, #75342, .T. ) ;
#57867=AXIS2_PLACEMENT_3D ( 'NONE', #6456, #95496, #57486 ) ;
#57872=CARTESIAN_POINT ( 'NONE',  ( 6.935134328181136176, -80.57830137131841752, 2.500000000002415401 ) ) ;
#57875=DIRECTION ( 'NONE',  ( -1.257402221000611116E-16, 1.000000000000000000, 0.000000000000000000 ) ) ;
#57883=CARTESIAN_POINT ( 'NONE',  ( -3.271890209819572792, -0.8418601081564157651, -2.499999999999999112 ) ) ;
#57891=CARTESIAN_POINT ( 'NONE',  ( 5.170525679121678486, -13.81869365337359845, -4.000000000000000000 ) ) ;
#57903=EDGE_CURVE ( 'NONE', #63872, #77456, #22049, .T. ) ;
#57904=SURFACE_SIDE_STYLE ('',( #96430 ) ) ;
#57906=AXIS2_PLACEMENT_3D ( 'NONE', #33143, #18652, #57126 ) ;
#57913=STYLED_ITEM ( 'NONE', ( #92657 ), #24988 ) ;
#57916=DIRECTION ( 'NONE',  ( 0.000000000000000000, 1.000000000000000000, -0.000000000000000000 ) ) ;
#57933=CARTESIAN_POINT ( 'NONE',  ( 4.471658927061713307, -3.629165645961075715, 3.750000000000000000 ) ) ;
#57957=LINE ( 'NONE', #44924, #69047 ) ;
#57958=ORIENTED_EDGE ( 'NONE', *, *, #83876, .F. ) ;
#57969=CARTESIAN_POINT ( 'NONE',  ( -3.377759596007864129, -3.629459927034941025, 2.500000000000000888 ) ) ;
#57975=CARTESIAN_POINT ( 'NONE',  ( 5.930053198192435815, -28.64714083316723503, 4.000000000000000000 ) ) ;
#57977=ORIENTED_EDGE ( 'NONE', *, *, #53534, .F. ) ;
#57985=DIRECTION ( 'NONE',  ( 1.000000000000000000, 0.000000000000000000, 0.000000000000000000 ) ) ;
#57988=CARTESIAN_POINT ( 'NONE',  ( 6.878063601867475008, -66.29791949882819324, -2.750000000000000000 ) ) ;
#57990=VECTOR ( 'NONE', #61790, 1000.000000000000114 ) ;
#58002=ORIENTED_EDGE ( 'NONE', *, *, #98245, .F. ) ;
#58017=CARTESIAN_POINT ( 'NONE',  ( 14.99999999999998046, 79.82179676972448590, 6.500000000000000888 ) ) ;
#58021=CARTESIAN_POINT ( 'NONE',  ( 17.90558034491733963, 78.11737700066652224, -4.059948642090408732 ) ) ;
#58025=EDGE_CURVE ( 'NONE', #19716, #70499, #67738, .T. ) ;
#58028=CARTESIAN_POINT ( 'NONE',  ( 3.969999999999999751, 10.00000000000000000, 2.750000000000000000 ) ) ;
#58029=PRESENTATION_STYLE_ASSIGNMENT (( #4565 ) ) ;
#58044=CARTESIAN_POINT ( 'NONE',  ( -3.772435416985459256, -6.430908609848360769, -4.000000000000000000 ) ) ;
#58051=CIRCLE ( 'NONE', #97989, 0.2500000000000002220 ) ;
#58055=CARTESIAN_POINT ( 'NONE',  ( 6.879999999999995453, 43.00000000000000000, -4.250000000000000000 ) ) ;
#58064=SURFACE_STYLE_FILL_AREA ( #57088 ) ;
#58076=ORIENTED_EDGE ( 'NONE', *, *, #21238, .F. ) ;
#58085=FILL_AREA_STYLE_COLOUR ( '', #84049 ) ;
#58090=CARTESIAN_POINT ( 'NONE',  ( 6.599999999999995204, -97.00000000000000000, 3.750000000000000000 ) ) ;
#58091=CARTESIAN_POINT ( 'NONE',  ( -3.990799379706100325, -9.967613007074422882, 2.750000000000000000 ) ) ;
#58093=CARTESIAN_POINT ( 'NONE',  ( -3.750000000000000888, 1.019547802438465212, 3.750000000000000000 ) ) ;
#58099=SURFACE_STYLE_FILL_AREA ( #57617 ) ;
#58107=ORIENTED_EDGE ( 'NONE', *, *, #48492, .T. ) ;
#58122=CARTESIAN_POINT ( 'NONE',  ( -11.26382985233585643, -93.42670896123698299, -3.750000000000000000 ) ) ;
#58130=EDGE_CURVE ( 'NONE', #2137, #14813, #62673, .T. ) ;
#58141=CARTESIAN_POINT ( 'NONE',  ( 17.74999999999999645, 91.00000000000000000, -8.000000000000000000 ) ) ;
#58142=CARTESIAN_POINT ( 'NONE',  ( 4.380000000000000782, -0.01592157648205478476, 2.750000000000000000 ) ) ;
#58147=FACE_OUTER_BOUND ( 'NONE', #72758, .T. ) ;
#58150=CARTESIAN_POINT ( 'NONE',  ( 4.879999999999994564, 43.00000000000000711, 4.250000000000000000 ) ) ;
#58163=CARTESIAN_POINT ( 'NONE',  ( -10.82635109531846673, -96.00292546281325201, 4.000000000000000000 ) ) ;
#58172=ORIENTED_EDGE ( 'NONE', *, *, #40812, .T. ) ;
#58174=ORIENTED_EDGE ( 'NONE', *, *, #44993, .F. ) ;
#58186=COLOUR_RGB ( '', 0.31764706, 0.68627451, 0.89019608) ;
#58197=COLOUR_RGB ( '', 0.40784314, 0.44705882, 0.49803922) ;
#58208=CARTESIAN_POINT ( 'NONE',  ( -6.000000000000000000, 78.07179676972447169, 6.500000000000000888 ) ) ;
#58209=DIRECTION ( 'NONE',  ( -0.000000000000000000, 0.000000000000000000, 1.000000000000000000 ) ) ;
#58216=EDGE_CURVE ( 'NONE', #66682, #12912, #48164, .T. ) ;
#58225=DIRECTION ( 'NONE',  ( 6.938893903907222067E-15, 0.000000000000000000, -1.000000000000000000 ) ) ;
#58236=CARTESIAN_POINT ( 'NONE',  ( 4.471369574522381818, -3.620508344108031018, 3.750000000000000444 ) ) ;
#58237=SURFACE_STYLE_FILL_AREA ( #4286 ) ;
#58241=FACE_OUTER_BOUND ( 'NONE', #66154, .T. ) ;
#58243=EDGE_CURVE ( 'NONE', #86107, #13092, #71181, .T. ) ;
#58247=CARTESIAN_POINT ( 'NONE',  ( -11.88867004768947488, 90.28252147127371074, -6.948627224671861669 ) ) ;
#58249=DIRECTION ( 'NONE',  ( -2.569960705150826877E-16, 1.000000000000000000, 0.000000000000000000 ) ) ;
#58250=CIRCLE ( 'NONE', #27936, 0.5000000000000004441 ) ;
#58266=DIRECTION ( 'NONE',  ( 1.000000000000000000, 0.000000000000000000, 0.000000000000000000 ) ) ;
#58287=SURFACE_SIDE_STYLE ('',( #28789 ) ) ;
#58293=AXIS2_PLACEMENT_3D ( 'NONE', #53325, #44831, #23840 ) ;
#58299=LINE ( 'NONE', #81315, #73254 ) ;
#58305=VERTEX_POINT ( 'NONE', #19526 ) ;
#58308=ORIENTED_EDGE ( 'NONE', *, *, #42353, .F. ) ;
#58348=CARTESIAN_POINT ( 'NONE',  ( 4.879999999999991900, 76.07179676972444327, -6.250000000000000000 ) ) ;
#58353=CARTESIAN_POINT ( 'NONE',  ( -8.000000000000000000, 80.99999999999994316, 2.900000000000001243 ) ) ;
#58355=ADVANCED_FACE ( 'NONE', ( #27508 ), #88510, .F. ) ;
#58365=ORIENTED_EDGE ( 'NONE', *, *, #9438, .F. ) ;
#58377=EDGE_CURVE ( 'NONE', #23275, #24577, #45472, .T. ) ;
#58378=CARTESIAN_POINT ( 'NONE',  ( 6.829574850505124139, -88.00372650098208283, -4.000000000000000000 ) ) ;
#58379=CARTESIAN_POINT ( 'NONE',  ( -8.900000000000002132, 80.99999999999994316, -2.900000000000000355 ) ) ;
#58394=STYLED_ITEM ( 'NONE', ( #13046 ), #35948 ) ;
#58398=CIRCLE ( 'NONE', #88740, 0.1000000000000001166 ) ;
#58403=CARTESIAN_POINT ( 'NONE',  ( -7.750000000000000000, 40.99999999999999289, -4.250000000000000000 ) ) ;
#58406=CARTESIAN_POINT ( 'NONE',  ( 7.361080431567760485, -0.6440110890646428832, 2.900000000000000355 ) ) ;
#58411=VERTEX_POINT ( 'NONE', #44487 ) ;
#58421=CIRCLE ( 'NONE', #83995, 2.750000000000000888 ) ;
#58443=VECTOR ( 'NONE', #76601, 1000.000000000000000 ) ;
#58446=ORIENTED_EDGE ( 'NONE', *, *, #84746, .F. ) ;
#58451=ORIENTED_EDGE ( 'NONE', *, *, #19126, .F. ) ;
#58460=DIRECTION ( 'NONE',  ( 0.9942165912674658657, -0.1073935270325955399, 0.000000000000000000 ) ) ;
#58462=MECHANICAL_DESIGN_GEOMETRIC_PRESENTATION_REPRESENTATION('',(#20144),#80821);
#58467=CARTESIAN_POINT ( 'NONE',  ( 7.160365893312770069, -84.29711206764774545, 3.999999999999999112 ) ) ;
#58471=EDGE_CURVE ( 'NONE', #69763, #94718, #30104, .T. ) ;
#58482=EDGE_LOOP ( 'NONE', ( #44945, #1640, #42495, #44363, #70047, #18253, #81742, #97400, #67574, #88190, #69746, #2237, #46068, #74282, #86865, #63156, #38743, #51076, #35463, #41203 ) ) ;
#58494=MECHANICAL_DESIGN_GEOMETRIC_PRESENTATION_REPRESENTATION('',(#9044),#64904);
#58512=CARTESIAN_POINT ( 'NONE',  ( 7.285838599102620089E-14, 21.00000000000003197, 3.000000000000000000 ) ) ;
#58524=LINE ( 'NONE', #51526, #57570 ) ;
#58526=ORIENTED_EDGE ( 'NONE', *, *, #93150, .F. ) ;
#58540=VECTOR ( 'NONE', #20757, 1000.000000000000000 ) ;
#58542=CARTESIAN_POINT ( 'NONE',  ( -3.500000000000000888, 1.019547802438454109, -4.000000000000000000 ) ) ;
#58551=CIRCLE ( 'NONE', #50567, 0.09999999999999982514 ) ;
#58558=ORIENTED_EDGE ( 'NONE', *, *, #43941, .T. ) ;
#58559=FILL_AREA_STYLE_COLOUR ( '', #66915 ) ;
#58560=ORIENTED_EDGE ( 'NONE', *, *, #72663, .T. ) ;
#58583=PRESENTATION_STYLE_ASSIGNMENT (( #88092 ) ) ;
#58588=EDGE_CURVE ( 'NONE', #45519, #12193, #48063, .T. ) ;
#58598=DIRECTION ( 'NONE',  ( 4.510281037539694028E-14, 1.000000000000000000, -0.000000000000000000 ) ) ;
#58612=DIRECTION ( 'NONE',  ( 1.000000000000000000, 2.641710877122040890E-15, 0.000000000000000000 ) ) ;
#58621=PRESENTATION_STYLE_ASSIGNMENT (( #75104 ) ) ;
#58625=SURFACE_SIDE_STYLE ('',( #95648 ) ) ;
#58632=CARTESIAN_POINT ( 'NONE',  ( -11.48880622960838593, -88.23206844530358239, -3.999999999998199218 ) ) ;
#58669=CARTESIAN_POINT ( 'NONE',  ( -10.91898769931337299, -97.58648078756493760, 4.000000000000000000 ) ) ;
#58678=CARTESIAN_POINT ( 'NONE',  ( 4.629999999999991900, 76.07179676972444327, -4.000000000000000000 ) ) ;
#58681=ORIENTED_EDGE ( 'NONE', *, *, #33608, .T. ) ;
#58683=ORIENTED_EDGE ( 'NONE', *, *, #98365, .T. ) ;
#58687=EDGE_CURVE ( 'NONE', #13062, #88822, #38036, .T. ) ;
#58689=AXIS2_PLACEMENT_3D ( 'NONE', #41116, #36050, #68041 ) ;
#58701=DIRECTION ( 'NONE',  ( 0.7808688094430307203, -0.6246950475544238435, 0.000000000000000000 ) ) ;
#58705=TOROIDAL_SURFACE ( 'NONE', #28379, 0.5000000000000000000, 0.2500000000000000000 ) ;
#58707=EDGE_CURVE ( 'NONE', #87189, #39787, #95542, .T. ) ;
#58710=FACE_OUTER_BOUND ( 'NONE', #51168, .T. ) ;
#58722=CARTESIAN_POINT ( 'NONE',  ( 3.969999999999999751, 36.75000000000000000, 3.750000000000000000 ) ) ;
#58730=CARTESIAN_POINT ( 'NONE',  ( 8.880000000000022098, 80.32179676972448590, 4.000000000000000000 ) ) ;
#58743=CYLINDRICAL_SURFACE ( 'NONE', #66465, 1.500000000000001332 ) ;
#58747=( NAMED_UNIT ( * ) SI_UNIT ( $, .STERADIAN. ) SOLID_ANGLE_UNIT ( ) );
#58751=CIRCLE ( 'NONE', #44331, 7.250000000000002665 ) ;
#58757=CARTESIAN_POINT ( 'NONE',  ( -13.86076281203281901, 90.90669854496248092, -7.842019570309373577 ) ) ;
#58769=VECTOR ( 'NONE', #86160, 1000.000000000000000 ) ;
#58774=CARTESIAN_POINT ( 'NONE',  ( -0.6999999999999975131, 99.99999999999998579, 8.000000000000000000 ) ) ;
#58779=COLOUR_RGB ( '', 0.09019608, 0.27058824, 0.51372549) ;
#58821=ADVANCED_FACE ( 'NONE', ( #33063 ), #4551, .T. ) ;
#58844=VECTOR ( 'NONE', #44419, 1000.000000000000000 ) ;
#58848=CARTESIAN_POINT ( 'NONE',  ( -8.000343251535921851, 84.06932101904432386, -3.750000000000000000 ) ) ;
#58853=CARTESIAN_POINT ( 'NONE',  ( -11.12340613366069419, 89.95527085539235657, -6.571742733942876669 ) ) ;
#58868=CARTESIAN_POINT ( 'NONE',  ( 0.000000000000000000, -97.00000000000000000, -3.750000000000000000 ) ) ;
#58869=CARTESIAN_POINT ( 'NONE',  ( -8.000000000000000000, 80.07179676972448590, -4.250000000000000000 ) ) ;
#58877=CARTESIAN_POINT ( 'NONE',  ( -7.124975165242272368, -78.82169502743931844, -2.750000000000000000 ) ) ;
#58884=EDGE_LOOP ( 'NONE', ( #65869, #50821, #49605 ) ) ;
#58887=CARTESIAN_POINT ( 'NONE',  ( -8.922167142635604620, 75.09950301435408448, -3.000000000000000000 ) ) ;
#58917=ORIENTED_EDGE ( 'NONE', *, *, #32045, .T. ) ;
#58928=PRESENTATION_STYLE_ASSIGNMENT (( #81919 ) ) ;
#58949=CIRCLE ( 'NONE', #26970, 0.2500000000000002220 ) ;
#58952=ORIENTED_EDGE ( 'NONE', *, *, #62755, .T. ) ;
#58960=CARTESIAN_POINT ( 'NONE',  ( -3.999999999999999112, 78.07179676972445748, 6.250000000000000000 ) ) ;
#58962=AXIS2_PLACEMENT_3D ( 'NONE', #37152, #38143, #60121 ) ;
#58969=CARTESIAN_POINT ( 'NONE',  ( -39.29878048780484789, 31.43902439024384776, -8.000000000000000000 ) ) ;
#58982=CYLINDRICAL_SURFACE ( 'NONE', #35583, 3.940000000000000835 ) ;
#58990=CARTESIAN_POINT ( 'NONE',  ( 18.00000000000000000, 77.34875458013688387, 4.131905931794615405 ) ) ;
#59004=DIRECTION ( 'NONE',  ( 0.000000000000000000, -1.000000000000000000, 0.000000000000000000 ) ) ;
#59006=CARTESIAN_POINT ( 'NONE',  ( -3.521020805652876007, -6.414291667507516337, -2.500000000000000000 ) ) ;
#59013=( GEOMETRIC_REPRESENTATION_CONTEXT ( 3 ) GLOBAL_UNCERTAINTY_ASSIGNED_CONTEXT ( ( #82127 ) ) GLOBAL_UNIT_ASSIGNED_CONTEXT ( ( #2504, #63933, #94447 ) ) REPRESENTATION_CONTEXT ( 'NONE', 'WORKASPACE' ) );
#59020=CARTESIAN_POINT ( 'NONE',  ( 4.219999999999999751, 9.750000000000000000, -4.000000000000000000 ) ) ;
#59038=CARTESIAN_POINT ( 'NONE',  ( 11.40652922194187369, -69.23660773168047911, -3.749999999999999556 ) ) ;
#59039=VERTEX_POINT ( 'NONE', #84437 ) ;
#59045=FILL_AREA_STYLE_COLOUR ( '', #47558 ) ;
#59052=DIRECTION ( 'NONE',  ( 0.9975640502598257520, -0.06975647374410356982, 0.000000000000000000 ) ) ;
#59059=VERTEX_POINT ( 'NONE', #36287 ) ;
#59069=ADVANCED_FACE ( 'NONE', ( #66276 ), #89773, .T. ) ;
#59071=EDGE_LOOP ( 'NONE', ( #96612, #29364, #38099, #76891 ) ) ;
#59086=FACE_OUTER_BOUND ( 'NONE', #21701, .T. ) ;
#59087=CARTESIAN_POINT ( 'NONE',  ( -5.069388085562224866, -24.96207786480668744, 3.750000000000001332 ) ) ;
#59094=CARTESIAN_POINT ( 'NONE',  ( 8.880000000000000782, -7.313785530894214126, 3.750000000000000000 ) ) ;
#59100=CARTESIAN_POINT ( 'NONE',  ( -8.399999999999998579, 98.49999999999998579, 8.000000000000000000 ) ) ;
#59109=CARTESIAN_POINT ( 'NONE',  ( -10.98829462902744858, 46.98606209026556968, -2.899999999999999467 ) ) ;
#59115=CARTESIAN_POINT ( 'NONE',  ( -10.91892017065343445, -97.58704351937099375, -3.750000000000000000 ) ) ;
#59118=EDGE_CURVE ( 'NONE', #87452, #24464, #12299, .T. ) ;
#59121=MECHANICAL_DESIGN_GEOMETRIC_PRESENTATION_REPRESENTATION('',(#76691),#83117);
#59126=UNCERTAINTY_MEASURE_WITH_UNIT (LENGTH_MEASURE( 1.000000000000000082E-05 ), #65581, 'distance_accuracy_value', 'NONE');
#59130=ORIENTED_EDGE ( 'NONE', *, *, #6639, .T. ) ;
#59143=CIRCLE ( 'NONE', #16055, 0.7500000000000006661 ) ;
#59145=CARTESIAN_POINT ( 'NONE',  ( -13.77612262535527954, 90.93158326518027934, 7.883772450803742338 ) ) ;
#59157=CARTESIAN_POINT ( 'NONE',  ( -11.26393249254987516, -93.42496533367179268, 3.999999999999998224 ) ) ;
#59169=CARTESIAN_POINT ( 'NONE',  ( -3.750000000000000000, 36.75000000000000000, -4.000000000000000000 ) ) ;
#59178=AXIS2_PLACEMENT_3D ( 'NONE', #58208, #88725, #43223 ) ;
#59183=EDGE_CURVE ( 'NONE', #23479, #88687, #80306, .T. ) ;
#59185=EDGE_LOOP ( 'NONE', ( #15728, #5595, #31623, #94507 ) ) ;
#59190=CARTESIAN_POINT ( 'NONE',  ( 12.14357320772536575, 54.02013147999952736, -3.000000000000000000 ) ) ;
#59192=EDGE_CURVE ( 'NONE', #29547, #89183, #13287, .T. ) ;
#59196=CARTESIAN_POINT ( 'NONE',  ( 4.879999999999991900, 76.07179676972444327, 6.250000000000000000 ) ) ;
#59201=STYLED_ITEM ( 'NONE', ( #2120 ), #46296 ) ;
#59202=CARTESIAN_POINT ( 'NONE',  ( 9.779999999999988702, 27.00436609429084811, -3.000000000000000000 ) ) ;
#59209=DIRECTION ( 'NONE',  ( 0.000000000000000000, 0.000000000000000000, 1.000000000000000000 ) ) ;
#59231=SURFACE_SIDE_STYLE ('',( #64751 ) ) ;
#59237=TOROIDAL_SURFACE ( 'NONE', #24156, 0.7500000000000008882, 0.2500000000000000000 ) ;
#59248=PRESENTATION_STYLE_ASSIGNMENT (( #28756 ) ) ;
#59249=DIRECTION ( 'NONE',  ( -0.000000000000000000, 1.000000000000000000, 0.000000000000000000 ) ) ;
#59252=ORIENTED_EDGE ( 'NONE', *, *, #73729, .T. ) ;
#59262=FACE_OUTER_BOUND ( 'NONE', #53317, .T. ) ;
#59269=UNCERTAINTY_MEASURE_WITH_UNIT (LENGTH_MEASURE( 1.000000000000000082E-05 ), #28776, 'distance_accuracy_value', 'NONE');
#59271=EDGE_CURVE ( 'NONE', #55464, #88425, #38104, .T. ) ;
#59281=EDGE_CURVE ( 'NONE', #63243, #15746, #90260, .T. ) ;
#59285=SURFACE_SIDE_STYLE ('',( #21300 ) ) ;
#59289=DIRECTION ( 'NONE',  ( 1.000000000000000000, 0.000000000000000000, 0.000000000000000000 ) ) ;
#59292=VECTOR ( 'NONE', #50674, 1000.000000000000000 ) ;
#59298=VERTEX_POINT ( 'NONE', #29271 ) ;
#59301=ORIENTED_EDGE ( 'NONE', *, *, #42395, .F. ) ;
#59311=( LENGTH_UNIT ( ) NAMED_UNIT ( * ) SI_UNIT ( .MILLI., .METRE. ) );
#59328=FILL_AREA_STYLE_COLOUR ( '', #846 ) ;
#59335=DIRECTION ( 'NONE',  ( 0.000000000000000000, 0.000000000000000000, 1.000000000000000000 ) ) ;
#59344=CARTESIAN_POINT ( 'NONE',  ( -12.94148294176549108, 90.75484370785780186, -7.596443435273322997 ) ) ;
#59353=VERTEX_POINT ( 'NONE', #21793 ) ;
#59355=ADVANCED_FACE ( 'NONE', ( #38761 ), #85991, .T. ) ;
#59363=B_SPLINE_SURFACE_WITH_KNOTS ( 'NONE', 3, 1, ( 
 ( #47222, #86224 ),
 ( #62717, #54721 ),
 ( #41232, #93217 ),
 ( #54237, #92733 ),
 ( #69749, #8739 ) ),
 .UNSPECIFIED., .F., .F., .F.,
 ( 4, 1, 4 ),
 ( 2, 2 ),
 ( 0.000000000000000000, 0.4679165934955020201, 1.000000000000000000 ),
 ( 0.000000000000000000, 1.000000000000000000 ),
 .UNSPECIFIED. ) ;
#59411=( NAMED_UNIT ( * ) SI_UNIT ( $, .STERADIAN. ) SOLID_ANGLE_UNIT ( ) );
#59435=CIRCLE ( 'NONE', #37115, 1.000000000000000888 ) ;
#59436=CYLINDRICAL_SURFACE ( 'NONE', #67466, 0.2500000000000002220 ) ;
#59453=CARTESIAN_POINT ( 'NONE',  ( 10.34946471146702152, -32.01331896740364158, 3.750000000000000000 ) ) ;
#59455=ORIENTED_EDGE ( 'NONE', *, *, #48537, .T. ) ;
#59458=CARTESIAN_POINT ( 'NONE',  ( 7.184033521041855330, -73.16344059793534882, 4.000000000000000888 ) ) ;
#59462=UNCERTAINTY_MEASURE_WITH_UNIT (LENGTH_MEASURE( 1.000000000000000082E-05 ), #69104, 'distance_accuracy_value', 'NONE');
#59470=DIRECTION ( 'NONE',  ( -0.000000000000000000, -0.000000000000000000, -1.000000000000000000 ) ) ;
#59471=EDGE_LOOP ( 'NONE', ( #61883, #24177, #63996, #18250 ) ) ;
#59486=ORIENTED_EDGE ( 'NONE', *, *, #57620, .F. ) ;
#59495=CARTESIAN_POINT ( 'NONE',  ( 4.380000000000002558, 1.019547802438462547, 2.750000000000000000 ) ) ;
#59502=CIRCLE ( 'NONE', #29163, 0.2500000000000034972 ) ;
#59510=CIRCLE ( 'NONE', #11397, 0.2499999999999998890 ) ;
#59512=ADVANCED_FACE ( 'NONE', ( #75269 ), #13784, .F. ) ;
#59517=CARTESIAN_POINT ( 'NONE',  ( -8.900000000000002132, 80.99999999999994316, 2.900000000000001243 ) ) ;
#59532=CARTESIAN_POINT ( 'NONE',  ( 11.04741838685800204, -95.58930130597927644, -3.750000000000000000 ) ) ;
#59542=DIRECTION ( 'NONE',  ( 0.6246950475544238435, 0.7808688094430307203, 0.000000000000000000 ) ) ;
#59554=ORIENTED_EDGE ( 'NONE', *, *, #18074, .T. ) ;
#59560=EDGE_CURVE ( 'NONE', #63305, #19716, #33227, .T. ) ;
#59591=TOROIDAL_SURFACE ( 'NONE', #64364, 11.15000000000026326, 0.2500000000000000000 ) ;
#59598=ADVANCED_FACE ( 'NONE', ( #61250 ), #59363, .T. ) ;
#59606=CARTESIAN_POINT ( 'NONE',  ( -3.530007528296587704, -1.230351260576522110, -2.750000000000000444 ) ) ;
#59608=DIRECTION ( 'NONE',  ( -1.483861936729427615E-16, 1.000000000000000000, -0.000000000000000000 ) ) ;
#59609=CARTESIAN_POINT ( 'NONE',  ( -16.94999999999999574, 99.99999999999998579, -8.525133428036873795 ) ) ;
#59622=EDGE_CURVE ( 'NONE', #74673, #84748, #63351, .T. ) ;
#59624=COLOUR_RGB ( '', 0.72549020, 0.75294118, 0.79215686) ;
#59643=ORIENTED_EDGE ( 'NONE', *, *, #52708, .T. ) ;
#59673=CARTESIAN_POINT ( 'NONE',  ( -3.750000000000000000, 78.07179676972445748, 4.250000000000000000 ) ) ;
#59675=ADVANCED_FACE ( 'NONE', ( #50822 ), #27814, .F. ) ;
#59681=ORIENTED_EDGE ( 'NONE', *, *, #71236, .F. ) ;
#59689=DIRECTION ( 'NONE',  ( 2.569960705150826877E-16, -1.000000000000000000, -0.000000000000000000 ) ) ;
#59691=ORIENTED_EDGE ( 'NONE', *, *, #59183, .F. ) ;
#59694=CARTESIAN_POINT ( 'NONE',  ( 8.879999999999991900, 27.04366094290857347, -2.900000000000000799 ) ) ;
#59698=DIRECTION ( 'NONE',  ( 0.000000000000000000, 0.000000000000000000, 1.000000000000000000 ) ) ;
#59710=CARTESIAN_POINT ( 'NONE',  ( 8.629999999999995453, 40.74999999999999289, 3.750000000000000000 ) ) ;
#59715=EDGE_CURVE ( 'NONE', #2137, #98319, #9394, .T. ) ;
#59717=EDGE_CURVE ( 'NONE', #39257, #52793, #63690, .T. ) ;
#59719=CARTESIAN_POINT ( 'NONE',  ( 8.880000000000020322, 79.82179676972448590, -6.500000000000000888 ) ) ;
#59723=( NAMED_UNIT ( * ) SI_UNIT ( $, .STERADIAN. ) SOLID_ANGLE_UNIT ( ) );
#59727=CARTESIAN_POINT ( 'NONE',  ( 8.880000000000020322, 79.82179676972448590, 6.500000000000000888 ) ) ;
#59734=EDGE_CURVE ( 'NONE', #91147, #63974, #17406, .T. ) ;
#59735=SURFACE_STYLE_USAGE ( .BOTH. , #23738 ) ;
#59744=FACE_OUTER_BOUND ( 'NONE', #52480, .T. ) ;
#59751=CARTESIAN_POINT ( 'NONE',  ( 11.33987066880781036, -87.82218667481943442, -3.999999999998208100 ) ) ;
#59765=DIRECTION ( 'NONE',  ( 1.000000000000000000, 0.000000000000000000, 0.000000000000000000 ) ) ;
#59766=VECTOR ( 'NONE', #89958, 1000.000000000000000 ) ;
#59772=DIRECTION ( 'NONE',  ( 1.000000000000000000, 1.387778780781444413E-14, 0.000000000000000000 ) ) ;
#59776=DIRECTION ( 'NONE',  ( -1.000000000000000000, 0.000000000000000000, 0.000000000000000000 ) ) ;
#59780=CARTESIAN_POINT ( 'NONE',  ( -3.586264863029322569, -2.711807932117639819, 3.999999999999596323 ) ) ;
#59781=EDGE_LOOP ( 'NONE', ( #8829, #88385, #71706, #88169 ) ) ;
#59784=ORIENTED_EDGE ( 'NONE', *, *, #63780, .T. ) ;
#59803=ADVANCED_FACE ( 'NONE', ( #54131 ), #53156, .T. ) ;
#59804=VERTEX_POINT ( 'NONE', #65806 ) ;
#59823=VERTEX_POINT ( 'NONE', #45659 ) ;
#59826=EDGE_CURVE ( 'NONE', #91690, #19964, #58299, .T. ) ;
#59836=VECTOR ( 'NONE', #28392, 1000.000000000000000 ) ;
#59842=DIRECTION ( 'NONE',  ( -0.000000000000000000, -0.000000000000000000, 1.000000000000000000 ) ) ;
#59847=ORIENTED_EDGE ( 'NONE', *, *, #6932, .T. ) ;
#59851=DIRECTION ( 'NONE',  ( 0.000000000000000000, 0.000000000000000000, -1.000000000000000000 ) ) ;
#59873=DIRECTION ( 'NONE',  ( 0.000000000000000000, 0.000000000000000000, -1.000000000000000000 ) ) ;
#59874=( NAMED_UNIT ( * ) PLANE_ANGLE_UNIT ( ) SI_UNIT ( $, .RADIAN. ) );
#59876=DIRECTION ( 'NONE',  ( 1.000000000000000000, 0.000000000000000000, -0.000000000000000000 ) ) ;
#59878=FACE_OUTER_BOUND ( 'NONE', #78904, .T. ) ;
#59900=FILL_AREA_STYLE ('',( #37921 ) ) ;
#59906=FILL_AREA_STYLE_COLOUR ( '', #89686 ) ;
#59911=MECHANICAL_DESIGN_GEOMETRIC_PRESENTATION_REPRESENTATION('',(#10389),#5612);
#59914=CARTESIAN_POINT ( 'NONE',  ( -8.000000000000000000, 80.32179676972448590, -3.750000000000000000 ) ) ;
#59916=VERTEX_POINT ( 'NONE', #64081 ) ;
#59928=COLOUR_RGB ( '', 0.40784314, 0.44705882, 0.49803922) ;
#59940=CARTESIAN_POINT ( 'NONE',  ( -6.606690058690507961, -50.93246948815529151, 2.750000000000000000 ) ) ;
#59943=DIRECTION ( 'NONE',  ( 0.000000000000000000, -0.000000000000000000, -1.000000000000000000 ) ) ;
#59944=CARTESIAN_POINT ( 'NONE',  ( 5.365133693937636394, -17.52547282955412911, -4.000000000000000888 ) ) ;
#59948=CARTESIAN_POINT ( 'NONE',  ( 7.007880867418011306, -58.32092081208355694, 4.000000000000000000 ) ) ;
#59977=ORIENTED_EDGE ( 'NONE', *, *, #1966, .T. ) ;
#59978=TOROIDAL_SURFACE ( 'NONE', #64740, 2.899999999999999467, 0.1000000000000000056 ) ;
#59979=FACE_OUTER_BOUND ( 'NONE', #22496, .T. ) ;
#60004=CARTESIAN_POINT ( 'NONE',  ( 18.00000000000000000, 91.21636964435548123, 8.000000000000000000 ) ) ;
#60013=CARTESIAN_POINT ( 'NONE',  ( 18.00000000000000355, 77.07179676972445748, -6.250000000000000000 ) ) ;
#60016=CARTESIAN_POINT ( 'NONE',  ( -5.999999999999994671, 43.00000000000000000, -6.250000000000000000 ) ) ;
#60021=CARTESIAN_POINT ( 'NONE',  ( -6.281594481400936125, -39.81112291747236043, -4.000000000000000000 ) ) ;
#60027=( NAMED_UNIT ( * ) PLANE_ANGLE_UNIT ( ) SI_UNIT ( $, .RADIAN. ) );
#60038=ORIENTED_EDGE ( 'NONE', *, *, #12999, .F. ) ;
#60039=EDGE_LOOP ( 'NONE', ( #76049, #41887, #82681, #87674 ) ) ;
#60041=ORIENTED_EDGE ( 'NONE', *, *, #49221, .F. ) ;
#60055=EDGE_LOOP ( 'NONE', ( #87127, #86955, #45307, #62510 ) ) ;
#60064=EDGE_CURVE ( 'NONE', #21427, #93614, #55625, .T. ) ;
#60091=CARTESIAN_POINT ( 'NONE',  ( -3.990799379706100325, -9.967613007074422882, -2.750000000000000444 ) ) ;
#60094=CARTESIAN_POINT ( 'NONE',  ( -19.64999999999999858, 92.00000000000000000, -8.000000000000000000 ) ) ;
#60101=FILL_AREA_STYLE_COLOUR ( '', #32442 ) ;
#60107=CONICAL_SURFACE ( 'NONE', #93658, 1.249999999999987121, 1.029744258676654312 ) ;
#60114=UNCERTAINTY_MEASURE_WITH_UNIT (LENGTH_MEASURE( 1.000000000000000082E-05 ), #66745, 'distance_accuracy_value', 'NONE');
#60118=VERTEX_POINT ( 'NONE', #47118 ) ;
#60120=EDGE_CURVE ( 'NONE', #97225, #22589, #8642, .T. ) ;
#60121=DIRECTION ( 'NONE',  ( 0.000000000000000000, 0.000000000000000000, -1.000000000000000000 ) ) ;
#60130=ORIENTED_EDGE ( 'NONE', *, *, #41929, .T. ) ;
#60131=CARTESIAN_POINT ( 'NONE',  ( -8.000000000000000000, 40.99999999999999289, 4.250000000000000000 ) ) ;
#60133=VECTOR ( 'NONE', #60441, 1000.000000000000000 ) ;
#60138=AXIS2_PLACEMENT_3D ( 'NONE', #28109, #74094, #52590 ) ;
#60143=CARTESIAN_POINT ( 'NONE',  ( -7.750000002553937506, -0.02145965645720818507, 4.000000000000000000 ) ) ;
#60149=DIRECTION ( 'NONE',  ( 0.000000000000000000, 0.000000000000000000, 1.000000000000000000 ) ) ;
#60156=CLOSED_SHELL ( 'NONE', ( #93070, #58821, #7689, #22643, #70810, #57032, #35211, #11973, #33558, #40082, #77779, #28482, #65095, #72720, #61971, #776, #49810, #33244, #72135, #87902, #59598, #3874, #30011, #43472, #28126, #87824, #30522, #73599, #79894, #86801, #29714, #57798, #40765, #37733, #60549, #57706, #80015, #15156, #51465, #36231, #22948, #61046, #65071, #54233, #83398, #33748, #20509, #48888, #48800, #1505, #41853, #6272, #23418, #43920, #78692, #92914, #36921, #95174, #9524, #79198, #50330, #98237, #39916, #34853, #31128, #61105, #97036, #55441, #50969, #89541, #62308, #13232, #88738, #88496, #68199, #25986, #44365, #53639, #23305, #49894, #74599, #77911, #60722, #74386, #57268, #8377, #9079, #92255, #33806, #4647, #19478, #63592, #30687, #84622, #18963, #28439, #11513, #33424, #46610, #35038, #27325, #19818, #53709, #74298, #8170, #96546, #14476, #78733, #88983, #78266, #98941, #81713, #35426, #95629, #41105, #55315, #83503, #80515, #40656, #27309, #28115, #38400, #7903, #72298, #83555, #17354, #52147, #69668, #3610, #89316, #12647, #90872, #45170, #66372, #55533, #85238, #70523, #69587, #1445, #14513, #24988, #66500, #47084, #52424, #72165, #34314, #62711, #94574, #40368, #84096, #62469, #49935, #93928, #62435, #41174, #60195, #77518, #17764, #12556, #818, #59512, #13790, #65927, #33401, #69324, #4684, #38078, #42517, #37606, #27673, #57083, #4481, #38853, #13728, #17991, #53296, #45605, #30369, #71604, #48292, #93184, #42728, #75652, #94194, #5038, #66347, #80489, #89831, #48631, #70016, #7167, #35208, #39060, #77457, #77673, #2776, #90669, #5997, #37372, #22494, #39648, #67807, #46435, #92469, #36713, #15837, #89872, #63320, #3431, #79694, #14192, #98724, #96915, #67519, #14479, #14065, #86133, #84999, #96348, #59675, #83936, #60167, #46296, #96833, #58355, #16638, #26841, #66015, #92799, #26526, #60234, #52391, #35948, #39083, #95230, #14380, #96216, #76215, #66016, #74243, #46100, #46646, #75723, #24342, #30569, #37262, #97716, #95646, #57125, #52187, #38967, #38010, #72715, #7221, #23577, #30076, #68884, #78361, #59069, #54859, #96435, #68084, #69470, #22896, #10558, #15970, #64226, #34765, #43141, #40771, #41331, #56335, #56625, #56121, #69204, #52302, #98614 ) ) ;
#60157=DIRECTION ( 'NONE',  ( 1.000000000000000000, 0.000000000000000000, 0.000000000000000000 ) ) ;
#60167=ADVANCED_FACE ( 'NONE', ( #56120 ), #65063, .F. ) ;
#60190=CYLINDRICAL_SURFACE ( 'NONE', #51620, 0.2500000000000002220 ) ;
#60191=AXIS2_PLACEMENT_3D ( 'NONE', #66212, #28219, #28714 ) ;
#60195=ADVANCED_FACE ( 'NONE', ( #42108 ), #17476, .T. ) ;
#60199=CARTESIAN_POINT ( 'NONE',  ( -7.750000000000000000, 80.32179676972448590, -4.000000000000000000 ) ) ;
#60212=COLOUR_RGB ( '', 0.31764706, 0.68627451, 0.89019608) ;
#60214=FACE_OUTER_BOUND ( 'NONE', #12177, .T. ) ;
#60221=( LENGTH_UNIT ( ) NAMED_UNIT ( * ) SI_UNIT ( .MILLI., .METRE. ) );
#60223=FACE_OUTER_BOUND ( 'NONE', #59471, .T. ) ;
#60225=DIRECTION ( 'NONE',  ( 0.000000000000000000, 0.000000000000000000, -1.000000000000000000 ) ) ;
#60234=ADVANCED_FACE ( 'NONE', ( #5082 ), #39805, .T. ) ;
#60250=CARTESIAN_POINT ( 'NONE',  ( 10.93739314578613353, -97.13232482343475738, -3.999999999999775291 ) ) ;
#60259=SURFACE_STYLE_FILL_AREA ( #22281 ) ;
#60274=CARTESIAN_POINT ( 'NONE',  ( 6.685141491970515659, -80.57575624204726239, -2.500000000000000000 ) ) ;
#60277=AXIS2_PLACEMENT_3D ( 'NONE', #91563, #44574, #37089 ) ;
#60278=CARTESIAN_POINT ( 'NONE',  ( -3.500000000000000888, 1.019547802438454109, 4.000000000000000000 ) ) ;
#60279=EDGE_LOOP ( 'NONE', ( #33815, #33509, #81844, #55972 ) ) ;
#60284=ORIENTED_EDGE ( 'NONE', *, *, #75787, .F. ) ;
#60288=CIRCLE ( 'NONE', #49081, 0.2500000000000002220 ) ;
#60289=SURFACE_SIDE_STYLE ('',( #92272 ) ) ;
#60333=CARTESIAN_POINT ( 'NONE',  ( 6.935134328184320296, -80.57830137102044432, -2.500000000001611156 ) ) ;
#60346=SURFACE_SIDE_STYLE ('',( #39338 ) ) ;
#60348=FACE_OUTER_BOUND ( 'NONE', #75346, .T. ) ;
#60351=CARTESIAN_POINT ( 'NONE',  ( 3.969999999999999751, 37.25000000000000000, 4.000000000000000000 ) ) ;
#60354=CARTESIAN_POINT ( 'NONE',  ( -6.867320125584340573, -58.36821204062217561, -2.500000000000000000 ) ) ;
#60375=UNCERTAINTY_MEASURE_WITH_UNIT (LENGTH_MEASURE( 1.000000000000000082E-05 ), #15029, 'distance_accuracy_value', 'NONE');
#60385=CARTESIAN_POINT ( 'NONE',  ( 14.99999999999998046, 79.82179676972448590, -6.500000000000000888 ) ) ;
#60398=VERTEX_POINT ( 'NONE', #60540 ) ;
#60401=EDGE_CURVE ( 'NONE', #15178, #79717, #44551, .T. ) ;
#60402=CARTESIAN_POINT ( 'NONE',  ( 5.680373670949098397, -28.65980262290164049, 3.999999999990341504 ) ) ;
#60403=SURFACE_SIDE_STYLE ('',( #28909 ) ) ;
#60408=ADVANCED_FACE ( 'NONE', ( #83050 ), #82553, .T. ) ;
#60436=DIRECTION ( 'NONE',  ( 1.000000000000000000, 0.000000000000000000, 0.000000000000000000 ) ) ;
#60441=DIRECTION ( 'NONE',  ( 1.483861936729427615E-16, -1.000000000000000000, -0.000000000000000000 ) ) ;
#60452=CARTESIAN_POINT ( 'NONE',  ( -9.524127588829090385, 88.37770237763953673, 5.051303975186559825 ) ) ;
#60457=CARTESIAN_POINT ( 'NONE',  ( -13.57366680649685087, 90.98132597431157365, -7.967802692208045379 ) ) ;
#60494=AXIS2_PLACEMENT_3D ( 'NONE', #12324, #43310, #8160 ) ;
#60498=CIRCLE ( 'NONE', #84424, 0.2500000000000002220 ) ;
#60503=LINE ( 'NONE', #46974, #8130 ) ;
#60514=DIRECTION ( 'NONE',  ( 0.000000000000000000, 0.000000000000000000, -1.000000000000000000 ) ) ;
#60519=CARTESIAN_POINT ( 'NONE',  ( -4.537879770911400712, -17.56524742834905695, -3.999999999996772360 ) ) ;
#60526=DIRECTION ( 'NONE',  ( -0.000000000000000000, -0.000000000000000000, 1.000000000000000000 ) ) ;
#60527=CARTESIAN_POINT ( 'NONE',  ( -8.350463100006260575, 86.22728700194303997, -4.047063141920883567 ) ) ;
#60540=CARTESIAN_POINT ( 'NONE',  ( 17.75000000000000000, 84.07179676972448590, -4.000000000000000000 ) ) ;
#60549=ADVANCED_FACE ( 'NONE', ( #24536 ), #85020, .F. ) ;
#60555=ORIENTED_EDGE ( 'NONE', *, *, #56758, .T. ) ;
#60567=CARTESIAN_POINT ( 'NONE',  ( 8.705946125382041600, -3.115782928399954521, 4.000000000000000000 ) ) ;
#60585=CARTESIAN_POINT ( 'NONE',  ( 8.629999999999991900, 70.25000000000000000, 6.500000000000000888 ) ) ;
#60595=CARTESIAN_POINT ( 'NONE',  ( -6.757332319902496387, -55.97232334539076959, -2.750000000000000444 ) ) ;
#60606=EDGE_CURVE ( 'NONE', #23275, #97363, #19031, .T. ) ;
#60629=VERTEX_POINT ( 'NONE', #71012 ) ;
#60630=EDGE_LOOP ( 'NONE', ( #44313, #11615, #1697, #13716 ) ) ;
#60637=CARTESIAN_POINT ( 'NONE',  ( -11.37817008395673035, -77.84129771019460975, 4.000000000000000000 ) ) ;
#60648=ORIENTED_EDGE ( 'NONE', *, *, #13576, .T. ) ;
#60653=ORIENTED_EDGE ( 'NONE', *, *, #64756, .T. ) ;
#60667=EDGE_CURVE ( 'NONE', #73802, #16898, #26484, .T. ) ;
#60680=SURFACE_STYLE_FILL_AREA ( #76185 ) ;
#60681=ORIENTED_EDGE ( 'NONE', *, *, #95280, .F. ) ;
#60682=PRESENTATION_STYLE_ASSIGNMENT (( #36719 ) ) ;
#60687=DIRECTION ( 'NONE',  ( -0.06975647374412512203, -0.9975640502598241977, 0.000000000000000000 ) ) ;
#60699=PRODUCT_CONTEXT ( 'NONE', #4669, 'mechanical' ) ;
#60704=DIRECTION ( 'NONE',  ( 0.8070303256584298035, -0.5905099943842175847, 0.000000000000000000 ) ) ;
#60722=ADVANCED_FACE ( 'NONE', ( #72966 ), #34962, .F. ) ;
#60736=CARTESIAN_POINT ( 'NONE',  ( 11.20666035742026878, -56.81027457018397087, -4.000000000000000000 ) ) ;
#60741=PRESENTATION_STYLE_ASSIGNMENT (( #30237 ) ) ;
#60758=LINE ( 'NONE', #45774, #96521 ) ;
#60767=( LENGTH_UNIT ( ) NAMED_UNIT ( * ) SI_UNIT ( .MILLI., .METRE. ) );
#60770=EDGE_LOOP ( 'NONE', ( #64809, #55383, #22576, #23301 ) ) ;
#60772=ORIENTED_EDGE ( 'NONE', *, *, #47745, .F. ) ;
#60776=ORIENTED_EDGE ( 'NONE', *, *, #40653, .T. ) ;
#60777=AXIS2_PLACEMENT_3D ( 'NONE', #35523, #5539, #73021 ) ;
#60782=CIRCLE ( 'NONE', #22469, 0.2500000000000002220 ) ;
#60788=( LENGTH_UNIT ( ) NAMED_UNIT ( * ) SI_UNIT ( .MILLI., .METRE. ) );
#60792=EDGE_CURVE ( 'NONE', #37672, #16289, #83438, .T. ) ;
#60806=LINE ( 'NONE', #46311, #57990 ) ;
#60810=CARTESIAN_POINT ( 'NONE',  ( -7.750000000000000000, 0.000000000000000000, 3.750000000000000000 ) ) ;
#60818=AXIS2_PLACEMENT_3D ( 'NONE', #41936, #71446, #2960 ) ;
#60819=CARTESIAN_POINT ( 'NONE',  ( 6.683985746565565655, -73.15435785421902892, -2.500000000000000888 ) ) ;
#60839=CARTESIAN_POINT ( 'NONE',  ( -9.793405416303651023, -28.00185549904734472, -4.000000000000000888 ) ) ;
#60847=DIRECTION ( 'NONE',  ( -1.000000000000000000, 0.000000000000000000, 0.000000000000000000 ) ) ;
#60855=ORIENTED_EDGE ( 'NONE', *, *, #73045, .F. ) ;
#60862=CARTESIAN_POINT ( 'NONE',  ( -6.000000000000009770, 40.74999999999999289, 4.000000000000000000 ) ) ;
#60871=EDGE_CURVE ( 'NONE', #16289, #25004, #74176, .T. ) ;
#60878=CARTESIAN_POINT ( 'NONE',  ( -3.750000000000000000, 0.000000000000000000, 2.750000000000000000 ) ) ;
#60887=AXIS2_PLACEMENT_3D ( 'NONE', #62802, #3297, #9816 ) ;
#60890=SURFACE_STYLE_FILL_AREA ( #59900 ) ;
#60895=CIRCLE ( 'NONE', #96096, 0.2500000000000002220 ) ;
#60896=CYLINDRICAL_SURFACE ( 'NONE', #41298, 0.2500000000000002220 ) ;
#60923=AXIS2_PLACEMENT_3D ( 'NONE', #72606, #11625, #80622 ) ;
#60938=CARTESIAN_POINT ( 'NONE',  ( -8.854007681963667054, 87.37522428062567315, 4.483348028977646393 ) ) ;
#60964=DIRECTION ( 'NONE',  ( -1.000000000000000000, -1.244644646440729013E-15, 0.000000000000000000 ) ) ;
#60989=CARTESIAN_POINT ( 'NONE',  ( -5.149999999999995026, 98.50000000000000000, -8.000000000000000000 ) ) ;
#60990=CIRCLE ( 'NONE', #78558, 0.2500000000000002220 ) ;
#61006=STYLED_ITEM ( 'NONE', ( #61456 ), #75652 ) ;
#61017=CARTESIAN_POINT ( 'NONE',  ( -13.38735934610854628, 90.81479509783851256, -7.611013694208273783 ) ) ;
#61026=ORIENTED_EDGE ( 'NONE', *, *, #12413, .F. ) ;
#61040=VERTEX_POINT ( 'NONE', #59719 ) ;
#61046=ADVANCED_FACE ( 'NONE', ( #96763 ), #28238, .T. ) ;
#61068=CARTESIAN_POINT ( 'NONE',  ( 6.579634127946654587, -87.99828267815715321, -2.750000000000000444 ) ) ;
#61069=VECTOR ( 'NONE', #90848, 1000.000000000000000 ) ;
#61076=DIRECTION ( 'NONE',  ( -0.5150380749100542666, 0.000000000000000000, 0.8571673007021122226 ) ) ;
#61087=DIRECTION ( 'NONE',  ( 0.000000000000000000, 1.000000000000000000, 0.000000000000000000 ) ) ;
#61090=AXIS2_PLACEMENT_3D ( 'NONE', #80493, #42492, #6960 ) ;
#61095=DIRECTION ( 'NONE',  ( 0.000000000000000000, -0.000000000000000000, 1.000000000000000000 ) ) ;
#61098=DIRECTION ( 'NONE',  ( 1.000000000000000000, 0.000000000000000000, 0.000000000000000000 ) ) ;
#61105=ADVANCED_FACE ( 'NONE', ( #4767 ), #35238, .F. ) ;
#61110=ORIENTED_EDGE ( 'NONE', *, *, #25755, .F. ) ;
#61121=CIRCLE ( 'NONE', #33914, 2.750000000000000888 ) ;
#61130=CARTESIAN_POINT ( 'NONE',  ( -11.23896940073626105, -88.22260584719931842, 4.000000000000000000 ) ) ;
#61135=( GEOMETRIC_REPRESENTATION_CONTEXT ( 3 ) GLOBAL_UNCERTAINTY_ASSIGNED_CONTEXT ( ( #25228 ) ) GLOBAL_UNIT_ASSIGNED_CONTEXT ( ( #77653, #23705, #8196 ) ) REPRESENTATION_CONTEXT ( 'NONE', 'WORKASPACE' ) );
#61152=DIRECTION ( 'NONE',  ( 0.000000000000000000, 1.000000000000000000, 0.000000000000000000 ) ) ;
#61161=STYLED_ITEM ( 'NONE', ( #87944 ), #9364 ) ;
#61171=EDGE_CURVE ( 'NONE', #74685, #66694, #52148, .T. ) ;
#61177=LINE ( 'NONE', #23700, #2112 ) ;
#61178=ORIENTED_EDGE ( 'NONE', *, *, #8490, .F. ) ;
#61200=ORIENTED_EDGE ( 'NONE', *, *, #73948, .T. ) ;
#61214=DIRECTION ( 'NONE',  ( 0.000000000000000000, 0.000000000000000000, 1.000000000000000000 ) ) ;
#61219=FACE_BOUND ( 'NONE', #25652, .T. ) ;
#61228=( NAMED_UNIT ( * ) PLANE_ANGLE_UNIT ( ) SI_UNIT ( $, .RADIAN. ) );
#61235=CARTESIAN_POINT ( 'NONE',  ( 10.95672020365094923, -56.81584260457628233, -4.000000000000000000 ) ) ;
#61244=CIRCLE ( 'NONE', #86800, 0.2500000000000004441 ) ;
#61247=EDGE_LOOP ( 'NONE', ( #28199, #61992, #12212, #91979, #56629, #92374, #71614, #45298, #3966, #91538, #34795, #13852, #93153, #82532, #71163, #93482 ) ) ;
#61250=FACE_OUTER_BOUND ( 'NONE', #49502, .T. ) ;
#61255=DIRECTION ( 'NONE',  ( -1.000000000000000000, -0.000000000000000000, -0.000000000000000000 ) ) ;
#61261=FILL_AREA_STYLE_COLOUR ( '', #74902 ) ;
#61278=SURFACE_STYLE_USAGE ( .BOTH. , #30773 ) ;
#61288=VERTEX_POINT ( 'NONE', #8216 ) ;
#61304=FACE_OUTER_BOUND ( 'NONE', #36097, .T. ) ;
#61312=CARTESIAN_POINT ( 'NONE',  ( 6.574584770534515066, -50.88238473842280030, -2.499999999999998224 ) ) ;
#61316=CARTESIAN_POINT ( 'NONE',  ( 6.034042420216372271, -36.05779855192275107, 2.750000000000000000 ) ) ;
#61322=CARTESIAN_POINT ( 'NONE',  ( 15.00000000000000000, 77.07179676972447169, -6.500000000000000888 ) ) ;
#61330=LINE ( 'NONE', #22864, #66705 ) ;
#61334=( LENGTH_UNIT ( ) NAMED_UNIT ( * ) SI_UNIT ( .MILLI., .METRE. ) );
#61336=VECTOR ( 'NONE', #19496, 1000.000000000000114 ) ;
#61340=CARTESIAN_POINT ( 'NONE',  ( 11.24699797944280100, 54.09857164847241506, 2.899999999999999467 ) ) ;
#61347=ORIENTED_EDGE ( 'NONE', *, *, #34080, .T. ) ;
#61349=CARTESIAN_POINT ( 'NONE',  ( -8.218815441056078086, -9.362071622917410352, -4.000000000000000888 ) ) ;
#61384=DIRECTION ( 'NONE',  ( -6.938893903907222067E-15, 1.000000000000000000, 0.000000000000000000 ) ) ;
#61391=ORIENTED_EDGE ( 'NONE', *, *, #3243, .T. ) ;
#61400=EDGE_CURVE ( 'NONE', #59039, #71742, #61698, .T. ) ;
#61401=MECHANICAL_DESIGN_GEOMETRIC_PRESENTATION_REPRESENTATION('',(#48622),#10385);
#61405=EDGE_LOOP ( 'NONE', ( #14773, #3135, #47753, #89561 ) ) ;
#61423=EDGE_LOOP ( 'NONE', ( #20696, #65164, #89723, #23900 ) ) ;
#61456=PRESENTATION_STYLE_ASSIGNMENT (( #30463 ) ) ;
#61461=CARTESIAN_POINT ( 'NONE',  ( 4.395886034088992034, -0.8422402087801302839, -4.000000000000000000 ) ) ;
#61482=DIRECTION ( 'NONE',  ( 0.02970531260815257105, -0.9995586998285053149, 1.111794303139694811E-13 ) ) ;
#61483=SURFACE_STYLE_USAGE ( .BOTH. , #38508 ) ;
#61486=FILL_AREA_STYLE_COLOUR ( '', #97993 ) ;
#61498=VERTEX_POINT ( 'NONE', #77675 ) ;
#61502=AXIS2_PLACEMENT_3D ( 'NONE', #75571, #68571, #16057 ) ;
#61505=DIRECTION ( 'NONE',  ( -0.000000000000000000, 0.000000000000000000, 1.000000000000000000 ) ) ;
#61510=SURFACE_STYLE_USAGE ( .BOTH. , #74 ) ;
#61533=EDGE_LOOP ( 'NONE', ( #52496, #38510, #81083, #61662, #55522, #80356 ) ) ;
#61540=CARTESIAN_POINT ( 'NONE',  ( 4.130000000000002558, 1.019547802438464768, 2.750000000000000000 ) ) ;
#61546=EDGE_LOOP ( 'NONE', ( #82206, #51917, #52403, #74421 ) ) ;
#61550=SURFACE_SIDE_STYLE ('',( #53063 ) ) ;
#61563=DIRECTION ( 'NONE',  ( 0.000000000000000000, 0.000000000000000000, -1.000000000000000000 ) ) ;
#61568=ORIENTED_EDGE ( 'NONE', *, *, #87719, .T. ) ;
#61574=CARTESIAN_POINT ( 'NONE',  ( -7.118731320094870973, -71.92838106472885329, -3.750000000000000000 ) ) ;
#61576=LINE ( 'NONE', #54078, #51722 ) ;
#61585=LINE ( 'NONE', #29603, #29001 ) ;
#61605=TOROIDAL_SURFACE ( 'NONE', #976, 2.250000000000001332, 0.2500000000000000000 ) ;
#61609=ORIENTED_EDGE ( 'NONE', *, *, #10623, .F. ) ;
#61614=CARTESIAN_POINT ( 'NONE',  ( -11.51383254013138746, -65.37322064362177798, 4.000000000000000000 ) ) ;
#61627=ORIENTED_EDGE ( 'NONE', *, *, #58471, .F. ) ;
#61632=LINE ( 'NONE', #23677, #51009 ) ;
#61633=EDGE_CURVE ( 'NONE', #21334, #43301, #10624, .T. ) ;
#61644=CARTESIAN_POINT ( 'NONE',  ( -3.335590168189929816, -2.700456006050037328, 2.500000000000000000 ) ) ;
#61657=VECTOR ( 'NONE', #4470, 1000.000000000000000 ) ;
#61659=DIRECTION ( 'NONE',  ( 0.6246950475544238435, 0.7808688094430307203, 0.000000000000000000 ) ) ;
#61660=EDGE_CURVE ( 'NONE', #41466, #33199, #24107, .T. ) ;
#61662=ORIENTED_EDGE ( 'NONE', *, *, #90871, .T. ) ;
#61676=CARTESIAN_POINT ( 'NONE',  ( 3.969999999999999751, 37.25000000000000000, -3.750000000000000000 ) ) ;
#61677=( GEOMETRIC_REPRESENTATION_CONTEXT ( 3 ) GLOBAL_UNCERTAINTY_ASSIGNED_CONTEXT ( ( #75123 ) ) GLOBAL_UNIT_ASSIGNED_CONTEXT ( ( #2327, #16325, #39325 ) ) REPRESENTATION_CONTEXT ( 'NONE', 'WORKASPACE' ) );
#61678=AXIS2_PLACEMENT_3D ( 'NONE', #2773, #55245, #55755 ) ;
#61696=FACE_BOUND ( 'NONE', #41960, .T. ) ;
#61698=CIRCLE ( 'NONE', #28161, 0.2500000000000002220 ) ;
#61700=CIRCLE ( 'NONE', #26596, 0.5000000000000000000 ) ;
#61716=DIRECTION ( 'NONE',  ( 0.000000000000000000, 1.000000000000000000, 0.000000000000000000 ) ) ;
#61740=CARTESIAN_POINT ( 'NONE',  ( 18.00000000000000000, 78.65120189252176885, 3.750000044091261309 ) ) ;
#61743=CARTESIAN_POINT ( 'NONE',  ( 6.879999999999995453, 43.00000000000000000, 6.500000000000000888 ) ) ;
#61759=VECTOR ( 'NONE', #55150, 1000.000000000000000 ) ;
#61761=ORIENTED_EDGE ( 'NONE', *, *, #84025, .T. ) ;
#61764=FACE_OUTER_BOUND ( 'NONE', #79783, .T. ) ;
#61769=( NAMED_UNIT ( * ) SI_UNIT ( $, .STERADIAN. ) SOLID_ANGLE_UNIT ( ) );
#61773=CIRCLE ( 'NONE', #66572, 0.2500000000000002220 ) ;
#61777=CARTESIAN_POINT ( 'NONE',  ( -8.900000000000000355, 75.76920769491746910, 3.000000000000000000 ) ) ;
#61784=ORIENTED_EDGE ( 'NONE', *, *, #56818, .T. ) ;
#61790=DIRECTION ( 'NONE',  ( 0.8070303256584298035, -0.5905099943842175847, 0.000000000000000000 ) ) ;
#61791=CARTESIAN_POINT ( 'NONE',  ( -3.500000492100856953, 0.08994241822825245480, -2.750000000000000888 ) ) ;
#61795=CYLINDRICAL_SURFACE ( 'NONE', #19949, 0.2500000000000002220 ) ;
#61800=( GEOMETRIC_REPRESENTATION_CONTEXT ( 3 ) GLOBAL_UNCERTAINTY_ASSIGNED_CONTEXT ( ( #42432 ) ) GLOBAL_UNIT_ASSIGNED_CONTEXT ( ( #21396, #5898, #44379 ) ) REPRESENTATION_CONTEXT ( 'NONE', 'WORKASPACE' ) );
#61803=CARTESIAN_POINT ( 'NONE',  ( 5.678900477192378560, -28.62996443916036782, -2.749999999998390177 ) ) ;
#61806=VECTOR ( 'NONE', #38934, 1000.000000000000000 ) ;
#61807=CARTESIAN_POINT ( 'NONE',  ( 6.905552584538047434, -69.44516986195191066, 2.750000000000000444 ) ) ;
#61837=CARTESIAN_POINT ( 'NONE',  ( 8.880000000000020322, 80.07179676972448590, 4.250000000000000000 ) ) ;
#61843=CARTESIAN_POINT ( 'NONE',  ( 6.879999999999995453, 43.00000000000000000, -6.500000000000000888 ) ) ;
#61858=DIRECTION ( 'NONE',  ( -1.000000000000000000, 0.000000000000000000, 0.000000000000000000 ) ) ;
#61874=CARTESIAN_POINT ( 'NONE',  ( 4.573751236499521866, -6.413519960490759786, 4.000000000000000000 ) ) ;
#61875=EDGE_CURVE ( 'NONE', #73541, #14052, #148, .T. ) ;
#61879=AXIS2_PLACEMENT_3D ( 'NONE', #87371, #19854, #57848 ) ;
#61881=DIRECTION ( 'NONE',  ( 0.000000000000000000, -1.000000000000000000, 0.000000000000000000 ) ) ;
#61883=ORIENTED_EDGE ( 'NONE', *, *, #51385, .T. ) ;
#61892=CIRCLE ( 'NONE', #46001, 3.000000000000000888 ) ;
#61900=ORIENTED_EDGE ( 'NONE', *, *, #19665, .T. ) ;
#61909=DIRECTION ( 'NONE',  ( -0.9961946980917462113, 0.08715574274765140739, -0.000000000000000000 ) ) ;
#61917=VECTOR ( 'NONE', #25144, 1000.000000000000000 ) ;
#61923=DIRECTION ( 'NONE',  ( 1.000000000000000000, 0.000000000000000000, 0.000000000000000000 ) ) ;
#61929=DIRECTION ( 'NONE',  ( 0.000000000000000000, -1.000000000000000000, 0.000000000000000000 ) ) ;
#61931=CARTESIAN_POINT ( 'NONE',  ( 4.395712687476568625, -0.8323168404034876344, 2.500000000000000000 ) ) ;
#61934=DIRECTION ( 'NONE',  ( 0.000000000000000000, 0.000000000000000000, 1.000000000000000000 ) ) ;
#61957=DIRECTION ( 'NONE',  ( -0.000000000000000000, -0.000000000000000000, 1.000000000000000000 ) ) ;
#61971=ADVANCED_FACE ( 'NONE', ( #92096 ), #37629, .T. ) ;
#61985=DIRECTION ( 'NONE',  ( 0.000000000000000000, -1.000000000000000000, 0.000000000000000000 ) ) ;
#61989=AXIS2_PLACEMENT_3D ( 'NONE', #53258, #45769, #30249 ) ;
#61992=ORIENTED_EDGE ( 'NONE', *, *, #57443, .T. ) ;
#62017=VERTEX_POINT ( 'NONE', #9089 ) ;
#62032=ORIENTED_EDGE ( 'NONE', *, *, #51544, .T. ) ;
#62036=LINE ( 'NONE', #92536, #1142 ) ;
#62037=DIRECTION ( 'NONE',  ( 0.000000000000000000, 0.000000000000000000, -1.000000000000000000 ) ) ;
#62041=MECHANICAL_DESIGN_GEOMETRIC_PRESENTATION_REPRESENTATION('',(#44496),#33275);
#62042=PRESENTATION_STYLE_ASSIGNMENT (( #78043 ) ) ;
#62047=ORIENTED_EDGE ( 'NONE', *, *, #16828, .T. ) ;
#62055=CARTESIAN_POINT ( 'NONE',  ( 4.219999999999999751, 10.25000000000000000, -2.750000000000000000 ) ) ;
#62064=CARTESIAN_POINT ( 'NONE',  ( -7.045329894599615450, -66.66420243593404393, -2.750000000000000444 ) ) ;
#62072=FACE_OUTER_BOUND ( 'NONE', #43367, .T. ) ;
#62073=( NAMED_UNIT ( * ) SI_UNIT ( $, .STERADIAN. ) SOLID_ANGLE_UNIT ( ) );
#62074=SURFACE_STYLE_USAGE ( .BOTH. , #1118 ) ;
#62093=COLOUR_RGB ( '', 0.72549020, 0.75294118, 0.79215686) ;
#62097=SURFACE_SIDE_STYLE ('',( #38630 ) ) ;
#62104=CARTESIAN_POINT ( 'NONE',  ( -8.159331231882687163, -4.163042900874275531, 4.000000000000000000 ) ) ;
#62113=AXIS2_PLACEMENT_3D ( 'NONE', #20316, #27306, #65299 ) ;
#62118=ORIENTED_EDGE ( 'NONE', *, *, #56748, .T. ) ;
#62124=CARTESIAN_POINT ( 'NONE',  ( 9.879999999999990123, 20.99999999999999645, -1.249999999999987121 ) ) ;
#62126=AXIS2_PLACEMENT_3D ( 'NONE', #62642, #93147, #70663 ) ;
#62145=ORIENTED_EDGE ( 'NONE', *, *, #78041, .F. ) ;
#62146=CARTESIAN_POINT ( 'NONE',  ( 8.991948000357622206, -4.139826107003811373, 4.000000000000000000 ) ) ;
#62148=DIRECTION ( 'NONE',  ( 1.000000000000000000, 0.000000000000000000, -0.000000000000000000 ) ) ;
#62151=CARTESIAN_POINT ( 'NONE',  ( -3.635384400432159158, -3.854802480546752896, 3.750000000000000444 ) ) ;
#62154=CARTESIAN_POINT ( 'NONE',  ( -9.990730578767625047, 46.91630561652144138, 0.000000000000000000 ) ) ;
#62155=DIRECTION ( 'NONE',  ( -1.000000000000000000, 0.000000000000000000, 0.000000000000000000 ) ) ;
#62159=CARTESIAN_POINT ( 'NONE',  ( 8.879999999999991900, 76.07179676972447169, 4.250000000000000000 ) ) ;
#62167=CARTESIAN_POINT ( 'NONE',  ( 6.910409932112633768, -84.29236789246745332, -2.750000000000000000 ) ) ;
#62170=DIRECTION ( 'NONE',  ( 0.000000000000000000, -1.000000000000000000, 0.000000000000000000 ) ) ;
#62175=CARTESIAN_POINT ( 'NONE',  ( 0.000000000000000000, 40.74999999999999289, 4.000000000000000000 ) ) ;
#62178=LINE ( 'NONE', #39710, #7350 ) ;
#62186=( NAMED_UNIT ( * ) PLANE_ANGLE_UNIT ( ) SI_UNIT ( $, .RADIAN. ) );
#62192=EDGE_CURVE ( 'NONE', #23594, #52793, #41578, .T. ) ;
#62200=PLANE ( 'NONE',  #23224 ) ;
#62217=DIRECTION ( 'NONE',  ( -1.000000000000000000, -0.000000000000000000, -0.000000000000000000 ) ) ;
#62220=CIRCLE ( 'NONE', #89346, 8.000000000000007105 ) ;
#62223=ORIENTED_EDGE ( 'NONE', *, *, #39998, .F. ) ;
#62226=SURFACE_STYLE_FILL_AREA ( #71225 ) ;
#62235=CARTESIAN_POINT ( 'NONE',  ( 4.469999999999999751, 37.00000000000000000, -4.000000000000000000 ) ) ;
#62240=CARTESIAN_POINT ( 'NONE',  ( -6.031993939708439889, -39.82530731230075105, 3.749999999999193090 ) ) ;
#62254=EDGE_LOOP ( 'NONE', ( #32400, #37609, #85030, #17957 ) ) ;
#62266=DIRECTION ( 'NONE',  ( 0.9975640502598257520, -0.06975647374410356982, 0.000000000000000000 ) ) ;
#62271=EDGE_CURVE ( 'NONE', #70565, #35851, #57625, .T. ) ;
#62277=CARTESIAN_POINT ( 'NONE',  ( -3.750000000000000000, 10.25000000000000000, 3.750000000000000000 ) ) ;
#62278=CARTESIAN_POINT ( 'NONE',  ( -5.329637805456036936, -28.67156944097240512, -2.750000000000000000 ) ) ;
#62284=AXIS2_PLACEMENT_3D ( 'NONE', #45555, #95223, #2794 ) ;
#62290=CARTESIAN_POINT ( 'NONE',  ( -8.000343251535921851, 84.06932101904432386, 3.750000000000000000 ) ) ;
#62292=EDGE_LOOP ( 'NONE', ( #46275, #10298, #40040 ) ) ;
#62293=CARTESIAN_POINT ( 'NONE',  ( 4.656459206270717743, -8.255604869861873141, 2.750000000000000000 ) ) ;
#62302=CARTESIAN_POINT ( 'NONE',  ( 8.880000000000000782, 1.116573172248542834E-15, -6.250000000000000000 ) ) ;
#62305=CARTESIAN_POINT ( 'NONE',  ( -8.468261785896212146, -9.345432893202591629, -3.750000000000000000 ) ) ;
#62308=ADVANCED_FACE ( 'NONE', ( #36526 ), #42537, .F. ) ;
#62324=DIRECTION ( 'NONE',  ( 1.000000000000000000, 0.000000000000000000, 0.000000000000000000 ) ) ;
#62330=DIRECTION ( 'NONE',  ( -2.569960705150826877E-16, 1.000000000000000000, 0.000000000000000000 ) ) ;
#62348=MECHANICAL_DESIGN_GEOMETRIC_PRESENTATION_REPRESENTATION('',(#49569),#12816);
#62361=CARTESIAN_POINT ( 'NONE',  ( 4.906778809679744668, -8.256987753881587011, 4.000000000000000000 ) ) ;
#62363=DIRECTION ( 'NONE',  ( -1.000000000000000000, 0.000000000000000000, 0.000000000000000000 ) ) ;
#62367=CARTESIAN_POINT ( 'NONE',  ( -4.021969307579355224, -6.415483651463646630, -4.000000000000000000 ) ) ;
#62370=VERTEX_POINT ( 'NONE', #58017 ) ;
#62391=CARTESIAN_POINT ( 'NONE',  ( -11.48810437782082694, -88.25603173497155751, 3.750000000000001332 ) ) ;
#62394=CARTESIAN_POINT ( 'NONE',  ( -7.750000000000000000, 79.82179676972448590, 6.250000000000000000 ) ) ;
#62397=SURFACE_SIDE_STYLE ('',( #93402 ) ) ;
#62415=DIRECTION ( 'NONE',  ( -0.000000000000000000, -0.000000000000000000, 1.000000000000000000 ) ) ;
#62417=CARTESIAN_POINT ( 'NONE',  ( 6.757497259948273438, -58.30388498758458127, 2.750000000000000000 ) ) ;
#62435=ADVANCED_FACE ( 'NONE', ( #89024 ), #33710, .T. ) ;
#62436=SURFACE_STYLE_FILL_AREA ( #25462 ) ;
#62438=CARTESIAN_POINT ( 'NONE',  ( 4.471658927162282637, -3.629165645957387554, -4.000000000000000000 ) ) ;
#62454=( GEOMETRIC_REPRESENTATION_CONTEXT ( 3 ) GLOBAL_UNCERTAINTY_ASSIGNED_CONTEXT ( ( #35266 ) ) GLOBAL_UNIT_ASSIGNED_CONTEXT ( ( #55945, #40457, #17943 ) ) REPRESENTATION_CONTEXT ( 'NONE', 'WORKASPACE' ) );
#62462=EDGE_LOOP ( 'NONE', ( #89376, #35415, #59486, #21390 ) ) ;
#62463=PRESENTATION_STYLE_ASSIGNMENT (( #32469 ) ) ;
#62464=DIRECTION ( 'NONE',  ( -0.000000000000000000, -0.000000000000000000, 1.000000000000000000 ) ) ;
#62469=ADVANCED_FACE ( 'NONE', ( #12530 ), #69486, .F. ) ;
#62471=CARTESIAN_POINT ( 'NONE',  ( 0.000000000000000000, 99.99999999999998579, 7.750000000000000000 ) ) ;
#62473=VERTEX_POINT ( 'NONE', #76976 ) ;
#62474=COLOUR_RGB ( '', 0.08235294, 0.09019608, 0.10196078) ;
#62495=CARTESIAN_POINT ( 'NONE',  ( 0.000000000000000000, -97.00000000000000000, -4.000000000000000000 ) ) ;
#62497=ORIENTED_EDGE ( 'NONE', *, *, #91988, .T. ) ;
#62499=DIRECTION ( 'NONE',  ( 0.000000000000000000, 0.000000000000000000, -1.000000000000000000 ) ) ;
#62510=ORIENTED_EDGE ( 'NONE', *, *, #655, .F. ) ;
#62522=EDGE_LOOP ( 'NONE', ( #50238, #18359, #87291, #78047 ) ) ;
#62523=( GEOMETRIC_REPRESENTATION_CONTEXT ( 3 ) GLOBAL_UNCERTAINTY_ASSIGNED_CONTEXT ( ( #12489 ) ) GLOBAL_UNIT_ASSIGNED_CONTEXT ( ( #17357, #18822, #10826 ) ) REPRESENTATION_CONTEXT ( 'NONE', 'WORKASPACE' ) );
#62536=FACE_OUTER_BOUND ( 'NONE', #57675, .T. ) ;
#62553=MECHANICAL_DESIGN_GEOMETRIC_PRESENTATION_REPRESENTATION('',(#70570),#69006);
#62555=CARTESIAN_POINT ( 'NONE',  ( -6.560019409699617832, -50.64698701990471363, -3.750000000000000000 ) ) ;
#62563=FACE_OUTER_BOUND ( 'NONE', #27820, .T. ) ;
#62566=LINE ( 'NONE', #69106, #92719 ) ;
#62572=SURFACE_STYLE_USAGE ( .BOTH. , #63070 ) ;
#62606=FACE_OUTER_BOUND ( 'NONE', #24738, .T. ) ;
#62620=MECHANICAL_DESIGN_GEOMETRIC_PRESENTATION_REPRESENTATION('',(#94609),#75411);
#62624=COLOUR_RGB ( '', 0.72549020, 0.75294118, 0.79215686) ;
#62632=CIRCLE ( 'NONE', #41890, 0.2500000000000002220 ) ;
#62636=( GEOMETRIC_REPRESENTATION_CONTEXT ( 3 ) GLOBAL_UNCERTAINTY_ASSIGNED_CONTEXT ( ( #8138 ) ) GLOBAL_UNIT_ASSIGNED_CONTEXT ( ( #18710, #73159, #78716 ) ) REPRESENTATION_CONTEXT ( 'NONE', 'WORKASPACE' ) );
#62642=CARTESIAN_POINT ( 'NONE',  ( -8.000000000000000000, 0.000000000000000000, 4.000000000000000000 ) ) ;
#62645=DIRECTION ( 'NONE',  ( 1.000000000000000000, 2.081668171172167567E-14, 0.000000000000000000 ) ) ;
#62646=DIRECTION ( 'NONE',  ( 1.000000000000000000, 0.000000000000000000, 0.000000000000000000 ) ) ;
#62647=AXIS2_PLACEMENT_3D ( 'NONE', #92417, #59943, #77403 ) ;
#62656=CARTESIAN_POINT ( 'NONE',  ( 18.00000000000000000, 78.80384757729335377, -3.750000000000000000 ) ) ;
#62662=CARTESIAN_POINT ( 'NONE',  ( 4.380000000000000782, 0.09086787938152994515, -2.750000000000000888 ) ) ;
#62673=LINE ( 'NONE', #9688, #53932 ) ;
#62676=DIRECTION ( 'NONE',  ( 0.08715574274765139351, 0.9961946980917461003, 0.000000000000000000 ) ) ;
#62686=AXIS2_PLACEMENT_3D ( 'NONE', #26422, #65404, #97917 ) ;
#62711=ADVANCED_FACE ( 'NONE', ( #21525 ), #31951, .F. ) ;
#62717=CARTESIAN_POINT ( 'NONE',  ( -11.88139889192316900, -91.33459011216928047, 3.750000000000000000 ) ) ;
#62728=CARTESIAN_POINT ( 'NONE',  ( 18.00000000000000000, 77.07179676972447169, 4.250000000000000000 ) ) ;
#62732=CARTESIAN_POINT ( 'NONE',  ( -5.331138373844170886, -28.69357394137554707, 4.000000000000000000 ) ) ;
#62733=VERTEX_POINT ( 'NONE', #85471 ) ;
#62734=CARTESIAN_POINT ( 'NONE',  ( -19.89999999999999858, 92.00000000000000000, 7.750000000000000000 ) ) ;
#62755=EDGE_CURVE ( 'NONE', #40169, #68676, #2492, .T. ) ;
#62759=TOROIDAL_SURFACE ( 'NONE', #33981, 0.5000000000000000000, 0.2500000000000000000 ) ;
#62763=EDGE_LOOP ( 'NONE', ( #44890, #60284, #85567, #45171 ) ) ;
#62771=VECTOR ( 'NONE', #45196, 1000.000000000000114 ) ;
#62773=CIRCLE ( 'NONE', #37248, 0.2500000000000002220 ) ;
#62783=EDGE_CURVE ( 'NONE', #14585, #38399, #55964, .T. ) ;
#62784=CARTESIAN_POINT ( 'NONE',  ( 0.000000000000000000, -97.00000000000000000, 3.750000000000000000 ) ) ;
#62793=CARTESIAN_POINT ( 'NONE',  ( 4.380000000000002558, 0.09086787937427767692, 2.750000000000001332 ) ) ;
#62802=CARTESIAN_POINT ( 'NONE',  ( -7.749999999999996447, 83.99999999999994316, 3.750000000000000000 ) ) ;
#62803=VECTOR ( 'NONE', #6744, 1000.000000000000000 ) ;
#62808=CIRCLE ( 'NONE', #38848, 0.2500000000000034972 ) ;
#62815=CARTESIAN_POINT ( 'NONE',  ( -10.06059601896260247, 88.97539449291203084, -5.490105317800711759 ) ) ;
#62823=SURFACE_SIDE_STYLE ('',( #876 ) ) ;
#62824=CARTESIAN_POINT ( 'NONE',  ( -6.430724159521294503, -88.51069574204372259, -4.000000000000000000 ) ) ;
#62835=SURFACE_SIDE_STYLE ('',( #32330 ) ) ;
#62844=DIRECTION ( 'NONE',  ( 0.6246950475544237324, 0.7808688094430306093, 0.000000000000000000 ) ) ;
#62846=CIRCLE ( 'NONE', #24548, 0.2500000000000002220 ) ;
#62867=FILL_AREA_STYLE_COLOUR ( '', #82808 ) ;
#62874=ORIENTED_EDGE ( 'NONE', *, *, #36631, .F. ) ;
#62891=ORIENTED_EDGE ( 'NONE', *, *, #83578, .T. ) ;
#62896=CARTESIAN_POINT ( 'NONE',  ( -11.58017868921325189, -84.10256047875394358, 3.750000000000000888 ) ) ;
#62905=CARTESIAN_POINT ( 'NONE',  ( -7.750000000000000000, 41.24999999999999289, 4.000000000000000000 ) ) ;
#62908=CARTESIAN_POINT ( 'NONE',  ( 0.000000000000000000, 36.75000000000000000, -2.500000000000000000 ) ) ;
#62920=LINE ( 'NONE', #10911, #69148 ) ;
#62921=CARTESIAN_POINT ( 'NONE',  ( 4.323026924237980850, -6.401461444700509595, 2.500000000000000000 ) ) ;
#62923=ORIENTED_EDGE ( 'NONE', *, *, #91320, .T. ) ;
#62941=PRESENTATION_STYLE_ASSIGNMENT (( #70957 ) ) ;
#62944=CARTESIAN_POINT ( 'NONE',  ( 6.564124673094354101, -0.5742864948665229452, 3.000000000000000000 ) ) ;
#62997=DIRECTION ( 'NONE',  ( 0.9961946980917453232, -0.08715574274766037244, 0.000000000000000000 ) ) ;
#63019=AXIS2_PLACEMENT_3D ( 'NONE', #77624, #70637, #63118 ) ;
#63050=VERTEX_POINT ( 'NONE', #75813 ) ;
#63057=CARTESIAN_POINT ( 'NONE',  ( -8.118176716543592519, 86.25458391402874270, 4.292297935673070164 ) ) ;
#63064=DIRECTION ( 'NONE',  ( 0.6246950475544238435, 0.7808688094430307203, 0.000000000000000000 ) ) ;
#63065=DIRECTION ( 'NONE',  ( -4.205390244792255888E-16, 1.000000000000000000, 0.000000000000000000 ) ) ;
#63069=CARTESIAN_POINT ( 'NONE',  ( 8.629999999999995453, 40.74999999999999289, 4.250000000000000000 ) ) ;
#63070=SURFACE_SIDE_STYLE ('',( #32573 ) ) ;
#63075=SURFACE_STYLE_USAGE ( .BOTH. , #22766 ) ;
#63087=PRESENTATION_STYLE_ASSIGNMENT (( #32592 ) ) ;
#63094=ORIENTED_EDGE ( 'NONE', *, *, #83639, .F. ) ;
#63109=DIRECTION ( 'NONE',  ( 0.000000000000000000, 0.000000000000000000, -1.000000000000000000 ) ) ;
#63112=ORIENTED_EDGE ( 'NONE', *, *, #29295, .F. ) ;
#63118=DIRECTION ( 'NONE',  ( 0.000000000000000000, -1.000000000000000000, 0.000000000000000000 ) ) ;
#63120=EDGE_CURVE ( 'NONE', #55896, #75803, #63801, .T. ) ;
#63121=STYLED_ITEM ( 'NONE', ( #51839 ), #84999 ) ;
#63138=CARTESIAN_POINT ( 'NONE',  ( -3.500000000000000444, 1.019547802438453887, 2.499999999999999556 ) ) ;
#63141=FACE_OUTER_BOUND ( 'NONE', #31114, .T. ) ;
#63156=ORIENTED_EDGE ( 'NONE', *, *, #63417, .T. ) ;
#63178=AXIS2_PLACEMENT_3D ( 'NONE', #34316, #78363, #87820 ) ;
#63180=VERTEX_POINT ( 'NONE', #20647 ) ;
#63188=UNCERTAINTY_MEASURE_WITH_UNIT (LENGTH_MEASURE( 1.000000000000000082E-05 ), #49725, 'distance_accuracy_value', 'NONE');
#63200=DIRECTION ( 'NONE',  ( -0.000000000000000000, 0.000000000000000000, 1.000000000000000000 ) ) ;
#63202=EDGE_CURVE ( 'NONE', #82102, #8279, #46501, .T. ) ;
#63204=UNCERTAINTY_MEASURE_WITH_UNIT (LENGTH_MEASURE( 1.000000000000000082E-05 ), #38628, 'distance_accuracy_value', 'NONE');
#63224=CARTESIAN_POINT ( 'NONE',  ( -7.037696230105376927, -86.26312365675100580, 3.750000000000000000 ) ) ;
#63243=VERTEX_POINT ( 'NONE', #44113 ) ;
#63250=ORIENTED_EDGE ( 'NONE', *, *, #41239, .F. ) ;
#63263=DIRECTION ( 'NONE',  ( -1.000000000000000000, -0.000000000000000000, -0.000000000000000000 ) ) ;
#63267=CARTESIAN_POINT ( 'NONE',  ( 9.779999999999990479, 18.09999999999999787, 0.000000000000000000 ) ) ;
#63277=VECTOR ( 'NONE', #66103, 1000.000000000000114 ) ;
#63293=EDGE_LOOP ( 'NONE', ( #42821, #82196, #54532, #76396 ) ) ;
#63297=CARTESIAN_POINT ( 'NONE',  ( -7.754961693898215991, 84.52280956283338753, -4.000000000000000000 ) ) ;
#63300=VECTOR ( 'NONE', #3970, 1000.000000000000000 ) ;
#63305=VERTEX_POINT ( 'NONE', #35134 ) ;
#63311=DIRECTION ( 'NONE',  ( 0.000000000000000000, 0.000000000000000000, -1.000000000000000000 ) ) ;
#63320=ADVANCED_FACE ( 'NONE', ( #29115 ), #51135, .T. ) ;
#63332=CIRCLE ( 'NONE', #69693, 3.000000000000002665 ) ;
#63351=LINE ( 'NONE', #93855, #31723 ) ;
#63362=EDGE_LOOP ( 'NONE', ( #92984, #97322, #80614 ) ) ;
#63379=VERTEX_POINT ( 'NONE', #98142 ) ;
#63389=LINE ( 'NONE', #64363, #53487 ) ;
#63392=CARTESIAN_POINT ( 'NONE',  ( 17.99999999999999645, 99.99999999999998579, 8.000000000000000000 ) ) ;
#63398=DIRECTION ( 'NONE',  ( 1.000000000000000000, -0.000000000000000000, -0.000000000000000000 ) ) ;
#63401=ORIENTED_EDGE ( 'NONE', *, *, #33837, .F. ) ;
#63408=VECTOR ( 'NONE', #22583, 1000.000000000000114 ) ;
#63410=DIRECTION ( 'NONE',  ( 0.000000000000000000, 0.000000000000000000, -1.000000000000000000 ) ) ;
#63411=CARTESIAN_POINT ( 'NONE',  ( 6.905507196109046397, -69.44000359832128311, 2.750000000000000000 ) ) ;
#63417=EDGE_CURVE ( 'NONE', #88425, #21334, #61585, .T. ) ;
#63418=FACE_OUTER_BOUND ( 'NONE', #24148, .T. ) ;
#63431=DIRECTION ( 'NONE',  ( 1.000000000000000000, 0.000000000000000000, 0.000000000000000000 ) ) ;
#63452=EDGE_CURVE ( 'NONE', #12785, #62370, #75328, .T. ) ;
#63454=VECTOR ( 'NONE', #43398, 1000.000000000000000 ) ;
#63459=EDGE_LOOP ( 'NONE', ( #42702, #30267, #28305, #2438 ) ) ;
#63460=( NAMED_UNIT ( * ) SI_UNIT ( $, .STERADIAN. ) SOLID_ANGLE_UNIT ( ) );
#63461=DIRECTION ( 'NONE',  ( 1.000000000000000000, 2.569960705150826877E-16, -0.000000000000000000 ) ) ;
#63471=( GEOMETRIC_REPRESENTATION_CONTEXT ( 3 ) GLOBAL_UNCERTAINTY_ASSIGNED_CONTEXT ( ( #54350 ) ) GLOBAL_UNIT_ASSIGNED_CONTEXT ( ( #21620, #83093, #53574 ) ) REPRESENTATION_CONTEXT ( 'NONE', 'WORKASPACE' ) );
#63485=CARTESIAN_POINT ( 'NONE',  ( -10.07524202709548611, -32.17782673090250256, -3.750000000000000444 ) ) ;
#63499=AXIS2_PLACEMENT_3D ( 'NONE', #92204, #69700, #75719 ) ;
#63506=ORIENTED_EDGE ( 'NONE', *, *, #27201, .T. ) ;
#63511=FACE_OUTER_BOUND ( 'NONE', #41446, .T. ) ;
#63518=ORIENTED_EDGE ( 'NONE', *, *, #5361, .T. ) ;
#63519=CARTESIAN_POINT ( 'NONE',  ( 4.219999999999999751, 10.00000000000000000, -2.750000000000000000 ) ) ;
#63526=DIRECTION ( 'NONE',  ( 1.000000000000000000, -0.000000000000000000, -0.000000000000000000 ) ) ;
#63533=DIRECTION ( 'NONE',  ( 1.000000000000000000, 0.000000000000000000, 0.000000000000000000 ) ) ;
#63534=( GEOMETRIC_REPRESENTATION_CONTEXT ( 3 ) GLOBAL_UNCERTAINTY_ASSIGNED_CONTEXT ( ( #85222 ) ) GLOBAL_UNIT_ASSIGNED_CONTEXT ( ( #75035, #60027, #91016 ) ) REPRESENTATION_CONTEXT ( 'NONE', 'WORKASPACE' ) );
#63544=DIRECTION ( 'NONE',  ( 1.000000000000000000, -0.000000000000000000, -0.000000000000000000 ) ) ;
#63552=VECTOR ( 'NONE', #67779, 1000.000000000000000 ) ;
#63554=AXIS2_PLACEMENT_3D ( 'NONE', #10241, #92743, #54732 ) ;
#63559=FILL_AREA_STYLE_COLOUR ( '', #47650 ) ;
#63564=CARTESIAN_POINT ( 'NONE',  ( -3.499999999999998668, 1.019547802438465434, -3.750000000000000000 ) ) ;
#63567=ORIENTED_EDGE ( 'NONE', *, *, #8602, .T. ) ;
#63592=ADVANCED_FACE ( 'NONE', ( #10568 ), #56075, .T. ) ;
#63599=ORIENTED_EDGE ( 'NONE', *, *, #6932, .F. ) ;
#63606=CARTESIAN_POINT ( 'NONE',  ( 4.219999999999999751, 10.25000000000000000, 4.000000000000000000 ) ) ;
#63610=EDGE_LOOP ( 'NONE', ( #8450, #34594, #96762 ) ) ;
#63618=AXIS2_PLACEMENT_3D ( 'NONE', #5796, #57792, #80802 ) ;
#63624=CARTESIAN_POINT ( 'NONE',  ( 11.10658183845692015, -52.67641232763506309, 4.000000000000000888 ) ) ;
#63628=CARTESIAN_POINT ( 'NONE',  ( 1.350000000000004086, 98.50000000000000000, -8.000000000000000000 ) ) ;
#63637=SURFACE_SIDE_STYLE ('',( #58099 ) ) ;
#63643=( BOUNDED_SURFACE ( )  B_SPLINE_SURFACE ( 3, 2, ( 
 ( #47304, #94662, #46820 ),
 ( #45852, #76342, #68851 ),
 ( #77804, #9319, #92813 ),
 ( #26171, #24343, #56662 ),
 ( #15853, #3183, #30832 ),
 ( #37869, #7859, #384 ),
 ( #87151, #45346, #62305 ),
 ( #69336, #46338, #38846 ),
 ( #33649, #64145, #75850 ),
 ( #8340, #60839, #31809 ),
 ( #23359, #7370, #53842 ),
 ( #91338, #16337, #54316 ),
 ( #84353, #84830, #8825 ),
 ( #68365, #39340, #98882 ),
 ( #22865, #41193, #1358 ),
 ( #71673, #53336, #66124 ),
 ( #43133, #42650, #73126 ),
 ( #28132, #4668, #27637 ),
 ( #49162, #50643, #3678 ),
 ( #73625, #58632, #89131 ),
 ( #65629, #5148, #34140 ),
 ( #34634, #95654, #58122 ),
 ( #20642, #97160, #42171 ),
 ( #36123, #51131, #43627 ),
 ( #81621, #19159, #41681 ),
 ( #12634, #57642, #59115 ),
 ( #88630, #35638, #80146 ),
 ( #50142, #72634, #13130 ) ),
 .UNSPECIFIED., .F., .F., .F. ) 
 B_SPLINE_SURFACE_WITH_KNOTS ( ( 4, 2, 2, 2, 2, 2, 2, 2, 2, 2, 2, 2, 2, 4 ),
 ( 3, 3 ),
 ( 0.000000000000000000, 0.003117204018079801700, 0.006234408036159603400, 0.01246881607231920680, 0.02493763214463841360, 0.03740644821695762040, 0.04987526428927682720, 0.06234408036159603400, 0.07481289643391524080, 0.08728171250623445454, 0.09351612054239405447, 0.09663332456047385444, 0.09819192656951375442, 0.09975052857855365440 ),
 ( 0.000000000000000000, 1.000000000000000000 ),
 .UNSPECIFIED. ) 
 GEOMETRIC_REPRESENTATION_ITEM ( )  RATIONAL_B_SPLINE_SURFACE ( (
 ( 1.000000000000000000, 0.7071067811865475727, 1.000000000000000000),
 ( 1.000000000000000000, 0.7071067811865475727, 1.000000000000000000),
 ( 1.000000000000000000, 0.7071067811865475727, 1.000000000000000000),
 ( 1.000000000000000000, 0.7071067811865475727, 1.000000000000000000),
 ( 1.000000000000000000, 0.7071067811865475727, 1.000000000000000000),
 ( 1.000000000000000000, 0.7071067811865475727, 1.000000000000000000),
 ( 1.000000000000000000, 0.7071067811865475727, 1.000000000000000000),
 ( 1.000000000000000000, 0.7071067811865475727, 1.000000000000000000),
 ( 1.000000000000000000, 0.7071067811865471286, 1.000000000000000000),
 ( 1.000000000000000000, 0.7071067811865471286, 1.000000000000000000),
 ( 1.000000000000000000, 0.7071067811865475727, 1.000000000000000000),
 ( 1.000000000000000000, 0.7071067811865475727, 1.000000000000000000),
 ( 1.000000000000000000, 0.7071067811865482389, 1.000000000000000000),
 ( 1.000000000000000000, 0.7071067811865482389, 1.000000000000000000),
 ( 1.000000000000000000, 0.7071067811865473507, 1.000000000000000000),
 ( 1.000000000000000000, 0.7071067811865473507, 1.000000000000000000),
 ( 1.000000000000000000, 0.7071067811865475727, 1.000000000000000000),
 ( 1.000000000000000000, 0.7071067811865475727, 1.000000000000000000),
 ( 1.000000000000000000, 0.7071067811865475727, 1.000000000000000000),
 ( 1.000000000000000000, 0.7071067811865475727, 1.000000000000000000),
 ( 1.000000000000000000, 0.7071067811865475727, 1.000000000000000000),
 ( 1.000000000000000000, 0.7071067811865475727, 1.000000000000000000),
 ( 1.000000000000000000, 0.7071067811865475727, 1.000000000000000000),
 ( 1.000000000000000000, 0.7071067811865475727, 1.000000000000000000),
 ( 1.000000000000000000, 0.7071067811865520136, 1.000000000000000000),
 ( 1.000000000000000000, 0.7071067811865520136, 1.000000000000000000),
 ( 1.000000000000000000, 0.7071067811865445751, 1.000000000000000000),
 ( 1.000000000000000000, 0.7071067811865445751, 1.000000000000000000) ) ) 
 REPRESENTATION_ITEM ( '' )  SURFACE ( )  );
#63650=DIRECTION ( 'NONE',  ( 0.000000000000000000, 0.000000000000000000, -1.000000000000000000 ) ) ;
#63652=CARTESIAN_POINT ( 'NONE',  ( 6.879999999999995453, 43.00000000000000000, -6.500000000000000888 ) ) ;
#63668=EDGE_LOOP ( 'NONE', ( #37311, #34434, #94830, #67543 ) ) ;
#63670=EDGE_CURVE ( 'NONE', #63050, #18880, #54252, .T. ) ;
#63679=EDGE_LOOP ( 'NONE', ( #93356, #97468, #24911, #87080 ) ) ;
#63690=CIRCLE ( 'NONE', #60494, 0.2500000000000002220 ) ;
#63694=ORIENTED_EDGE ( 'NONE', *, *, #45398, .F. ) ;
#63702=( LENGTH_UNIT ( ) NAMED_UNIT ( * ) SI_UNIT ( .MILLI., .METRE. ) );
#63709=CARTESIAN_POINT ( 'NONE',  ( 18.00000000000000000, 78.20644475923570837, 3.828778322547196300 ) ) ;
#63712=CARTESIAN_POINT ( 'NONE',  ( -3.772435417270453506, -6.430908609835228162, 3.750000000000806466 ) ) ;
#63737=DIRECTION ( 'NONE',  ( -1.000000000000000000, -0.000000000000000000, -0.000000000000000000 ) ) ;
#63751=( LENGTH_UNIT ( ) NAMED_UNIT ( * ) SI_UNIT ( .MILLI., .METRE. ) );
#63776=CARTESIAN_POINT ( 'NONE',  ( -18.00000000000000355, 75.73428692542562146, 3.000000000000000000 ) ) ;
#63780=EDGE_CURVE ( 'NONE', #58411, #40169, #6680, .T. ) ;
#63798=DIRECTION ( 'NONE',  ( 1.000000000000000000, 0.000000000000000000, -0.000000000000000000 ) ) ;
#63801=B_SPLINE_CURVE_WITH_KNOTS ( 'NONE', 3,
 ( #90308, #22338, #77283, #52325, #90810, #69804, #14338, #37344, #1327, #31779, #67834, #351, #52126, #88142, #36128, #20143, #72639, #19654 ),
 .UNSPECIFIED., .F., .F.,
 ( 4, 2, 2, 2, 2, 2, 2, 2, 4 ),
 ( 2.168404344971008868E-18, 0.002783576088282441099, 0.005567152176564879595, 0.01113430435312975572, 0.02226860870625951144, 0.04453721741251901595, 0.06680582611877852739, 0.07794013047190828658, 0.08907443482503803189 ),
 .UNSPECIFIED. ) ;
#63803=DIRECTION ( 'NONE',  ( 0.000000000000000000, 0.000000000000000000, -1.000000000000000000 ) ) ;
#63814=CARTESIAN_POINT ( 'NONE',  ( -9.024359497401759356, 75.07164295747612925, 3.000000000000000000 ) ) ;
#63826=ORIENTED_EDGE ( 'NONE', *, *, #4812, .T. ) ;
#63833=CARTESIAN_POINT ( 'NONE',  ( 0.000000000000000000, 91.25000000000000000, 8.000000000000000000 ) ) ;
#63846=DIRECTION ( 'NONE',  ( 0.000000000000000000, 0.000000000000000000, 1.000000000000000000 ) ) ;
#63847=DIRECTION ( 'NONE',  ( 0.06975647374412534407, 0.9975640502598241977, 0.000000000000000000 ) ) ;
#63849=CIRCLE ( 'NONE', #76640, 3.940000000000000835 ) ;
#63851=VECTOR ( 'NONE', #83394, 1000.000000000000114 ) ;
#63854=ORIENTED_EDGE ( 'NONE', *, *, #25686, .F. ) ;
#63865=CARTESIAN_POINT ( 'NONE',  ( -15.00000000000004974, 91.25000000000000000, -7.750000000000000000 ) ) ;
#63870=EDGE_CURVE ( 'NONE', #70565, #11027, #67534, .T. ) ;
#63872=VERTEX_POINT ( 'NONE', #84011 ) ;
#63876=EDGE_CURVE ( 'NONE', #74806, #34483, #52, .T. ) ;
#63879=EDGE_CURVE ( 'NONE', #37066, #38896, #3479, .T. ) ;
#63894=CARTESIAN_POINT ( 'NONE',  ( -7.750000000000000000, 40.99999999999999289, 4.250000000000000000 ) ) ;
#63900=CIRCLE ( 'NONE', #46370, 0.5000000000000004441 ) ;
#63902=EDGE_CURVE ( 'NONE', #95826, #70674, #17814, .T. ) ;
#63904=CARTESIAN_POINT ( 'NONE',  ( 11.10000000000000142, 98.49999999999998579, -8.525133428036873795 ) ) ;
#63905=CARTESIAN_POINT ( 'NONE',  ( -4.535014064424438551, -17.52590857052339146, -2.499999999999193534 ) ) ;
#63910=AXIS2_PLACEMENT_3D ( 'NONE', #40955, #96422, #3447 ) ;
#63912=CARTESIAN_POINT ( 'NONE',  ( 4.823529266124356063, -6.402884419280910677, -4.000000000000000000 ) ) ;
#63933=( NAMED_UNIT ( * ) PLANE_ANGLE_UNIT ( ) SI_UNIT ( $, .RADIAN. ) );
#63938=VECTOR ( 'NONE', #65135, 1000.000000000000000 ) ;
#63953=DIRECTION ( 'NONE',  ( 0.000000000000000000, 0.000000000000000000, -1.000000000000000000 ) ) ;
#63958=CARTESIAN_POINT ( 'NONE',  ( -11.60530215607347948, -82.03068034365578853, -3.750000000000000000 ) ) ;
#63974=VERTEX_POINT ( 'NONE', #60013 ) ;
#63977=CIRCLE ( 'NONE', #70429, 0.5000000000000004441 ) ;
#63981=AXIS2_PLACEMENT_3D ( 'NONE', #76496, #45500, #19439 ) ;
#63996=ORIENTED_EDGE ( 'NONE', *, *, #44473, .F. ) ;
#63998=DIRECTION ( 'NONE',  ( 0.000000000000000000, 1.000000000000000000, -0.000000000000000000 ) ) ;
#64003=( NAMED_UNIT ( * ) SI_UNIT ( $, .STERADIAN. ) SOLID_ANGLE_UNIT ( ) );
#64029=CARTESIAN_POINT ( 'NONE',  ( 7.361080431567760485, -0.6440110890646428832, 3.000000000000000000 ) ) ;
#64047=CARTESIAN_POINT ( 'NONE',  ( -3.521924875522737253, -0.8399941893316781316, -3.750000000000001332 ) ) ;
#64074=SURFACE_STYLE_USAGE ( .BOTH. , #41121 ) ;
#64081=CARTESIAN_POINT ( 'NONE',  ( 8.880000000000000782, 1.019547802438458550, -3.750000000000000000 ) ) ;
#64082=VERTEX_POINT ( 'NONE', #12938 ) ;
#64106=CIRCLE ( 'NONE', #41802, 0.2500000000000000000 ) ;
#64108=CARTESIAN_POINT ( 'NONE',  ( -4.000000000000000000, 10.25000000000000000, -2.750000000000000000 ) ) ;
#64109=EDGE_LOOP ( 'NONE', ( #2781, #13562, #8712, #61900 ) ) ;
#64110=CARTESIAN_POINT ( 'NONE',  ( 8.959592931194404031, -9.312622102008740299, 4.000000000000000000 ) ) ;
#64114=( GEOMETRIC_REPRESENTATION_CONTEXT ( 3 ) GLOBAL_UNCERTAINTY_ASSIGNED_CONTEXT ( ( #42310 ) ) GLOBAL_UNIT_ASSIGNED_CONTEXT ( ( #60788, #84306, #68803 ) ) REPRESENTATION_CONTEXT ( 'NONE', 'WORKASPACE' ) );
#64115=CARTESIAN_POINT ( 'NONE',  ( -3.711005778769052021, -5.293034685380286319, 2.750000000000000000 ) ) ;
#64123=CIRCLE ( 'NONE', #76914, 0.2500000000000002220 ) ;
#64127=( NAMED_UNIT ( * ) SI_UNIT ( $, .STERADIAN. ) SOLID_ANGLE_UNIT ( ) );
#64139=CARTESIAN_POINT ( 'NONE',  ( 6.579634127946654587, -87.99828267815715321, 3.250000000000000888 ) ) ;
#64145=CARTESIAN_POINT ( 'NONE',  ( -9.206646936938154724, -19.70874149522700591, -4.000000000000000888 ) ) ;
#64160=CARTESIAN_POINT ( 'NONE',  ( 8.879999999999995453, 40.99999999999999289, -3.750000000000000000 ) ) ;
#64161=UNCERTAINTY_MEASURE_WITH_UNIT (LENGTH_MEASURE( 1.000000000000000082E-05 ), #36300, 'distance_accuracy_value', 'NONE');
#64167=DIRECTION ( 'NONE',  ( -0.000000000000000000, -0.000000000000000000, -1.000000000000000000 ) ) ;
#64173=CARTESIAN_POINT ( 'NONE',  ( 9.779999999999990479, 20.99999999999999645, 3.000000000000000000 ) ) ;
#64181=CARTESIAN_POINT ( 'NONE',  ( 12.24319267753454099, 54.01141590572476048, -2.899999999999999467 ) ) ;
#64187=SURFACE_SIDE_STYLE ('',( #40727 ) ) ;
#64194=AXIS2_PLACEMENT_3D ( 'NONE', #93042, #91069, #40051 ) ;
#64199=CARTESIAN_POINT ( 'NONE',  ( -4.262581423003701353, -13.85606188143274231, 3.749999999999193090 ) ) ;
#64201=DIRECTION ( 'NONE',  ( 0.000000000000000000, 0.000000000000000000, -1.000000000000000000 ) ) ;
#64213=EDGE_LOOP ( 'NONE', ( #81686, #50914, #58365, #71157 ) ) ;
#64226=ADVANCED_FACE ( 'NONE', ( #84409 ), #8399, .T. ) ;
#64232=DIRECTION ( 'NONE',  ( -1.000000000000000000, 0.000000000000000000, -0.000000000000000000 ) ) ;
#64239=CARTESIAN_POINT ( 'NONE',  ( -18.89999999999999147, 91.25000000000000000, 8.000000000000000000 ) ) ;
#64248=CARTESIAN_POINT ( 'NONE',  ( -8.636324037029986300, 86.94567068113131825, 4.522730969307667159 ) ) ;
#64251=ORIENTED_EDGE ( 'NONE', *, *, #18631, .F. ) ;
#64258=CIRCLE ( 'NONE', #21184, 0.2499999999999999445 ) ;
#64261=DIRECTION ( 'NONE',  ( -1.000000000000000000, 0.000000000000000000, 0.000000000000000000 ) ) ;
#64266=CARTESIAN_POINT ( 'NONE',  ( 8.979999999999991545, 21.00000000000000000, 2.900000000000000355 ) ) ;
#64270=STYLED_ITEM ( 'NONE', ( #56217 ), #73599 ) ;
#64271=CARTESIAN_POINT ( 'NONE',  ( -3.771300335753330568, -6.411622728200643273, 2.749999999999999556 ) ) ;
#64275=DIRECTION ( 'NONE',  ( 1.000000000000000000, 0.000000000000000000, 0.000000000000000000 ) ) ;
#64282=EDGE_LOOP ( 'NONE', ( #25886, #36916, #8059, #46387 ) ) ;
#64283=LINE ( 'NONE', #86324, #78166 ) ;
#64299=UNCERTAINTY_MEASURE_WITH_UNIT (LENGTH_MEASURE( 1.000000000000000082E-05 ), #77680, 'distance_accuracy_value', 'NONE');
#64311=CARTESIAN_POINT ( 'NONE',  ( 0.4400000000000020006, 1.019547802438468986, 2.500000000000000000 ) ) ;
#64321=CARTESIAN_POINT ( 'NONE',  ( -19.64999999999999858, 92.00000000000000000, -7.750000000000000000 ) ) ;
#64335=STYLED_ITEM ( 'NONE', ( #89019 ), #93070 ) ;
#64343=CARTESIAN_POINT ( 'NONE',  ( -6.000000000000000000, 78.07179676972447169, 6.500000000000000888 ) ) ;
#64360=CARTESIAN_POINT ( 'NONE',  ( -11.07412464642555250, -96.03934428903617970, 3.750000000000000888 ) ) ;
#64363=CARTESIAN_POINT ( 'NONE',  ( -8.000000000000000000, 75.73428692542562146, 3.000000000000000000 ) ) ;
#64364=AXIS2_PLACEMENT_3D ( 'NONE', #74116, #11659, #57644 ) ;
#64366=CARTESIAN_POINT ( 'NONE',  ( -6.000000000000009770, 40.74999999999999289, -4.000000000000000000 ) ) ;
#64383=DIRECTION ( 'NONE',  ( -0.000000000000000000, -0.000000000000000000, 1.000000000000000000 ) ) ;
#64387=CARTESIAN_POINT ( 'NONE',  ( 11.35674369515838933, -65.10150209588266534, 3.750000000000001332 ) ) ;
#64398=CARTESIAN_POINT ( 'NONE',  ( -3.770608837273494274, -6.399801140528821541, -2.500000000000403677 ) ) ;
#64403=FACE_OUTER_BOUND ( 'NONE', #50709, .T. ) ;
#64406=CARTESIAN_POINT ( 'NONE',  ( 6.905642986259637794, -69.45547628558860254, -3.750000000000000000 ) ) ;
#64418=ORIENTED_EDGE ( 'NONE', *, *, #65634, .T. ) ;
#64419=DIRECTION ( 'NONE',  ( 0.000000000000000000, 0.000000000000000000, -1.000000000000000000 ) ) ;
#64421=UNCERTAINTY_MEASURE_WITH_UNIT (LENGTH_MEASURE( 1.000000000000000082E-05 ), #90700, 'distance_accuracy_value', 'NONE');
#64429=DIRECTION ( 'NONE',  ( 1.000000000000000000, 0.000000000000000000, 0.000000000000000000 ) ) ;
#64430=CARTESIAN_POINT ( 'NONE',  ( -10.29975640502598289, 43.93058911311638326, -2.900000000000000799 ) ) ;
#64441=ORIENTED_EDGE ( 'NONE', *, *, #734, .F. ) ;
#64476=CARTESIAN_POINT ( 'NONE',  ( -4.285591316845102305, -17.54293119412275104, 2.499999999999998668 ) ) ;
#64492=DIRECTION ( 'NONE',  ( -0.000000000000000000, -0.000000000000000000, 1.000000000000000000 ) ) ;
#64499=ORIENTED_EDGE ( 'NONE', *, *, #7243, .T. ) ;
#64531=CARTESIAN_POINT ( 'NONE',  ( 18.00000000000000000, 78.50170875364489120, -3.769097879698134257 ) ) ;
#64532=TOROIDAL_SURFACE ( 'NONE', #93309, 2.899999999999999911, 0.1000000000000000056 ) ;
#64538=( NAMED_UNIT ( * ) SI_UNIT ( $, .STERADIAN. ) SOLID_ANGLE_UNIT ( ) );
#64540=ORIENTED_EDGE ( 'NONE', *, *, #28646, .F. ) ;
#64542=VECTOR ( 'NONE', #39954, 1000.000000000000000 ) ;
#64549=DIRECTION ( 'NONE',  ( 0.000000000000000000, 1.000000000000000000, 0.000000000000000000 ) ) ;
#64551=DIRECTION ( 'NONE',  ( 0.000000000000000000, 0.000000000000000000, 1.000000000000000000 ) ) ;
#64553=EDGE_CURVE ( 'NONE', #67870, #55759, #6747, .T. ) ;
#64561=DIRECTION ( 'NONE',  ( -0.9961946980917453232, 0.08715574274766037244, 0.000000000000000000 ) ) ;
#64571=DIRECTION ( 'NONE',  ( -0.000000000000000000, 0.000000000000000000, 1.000000000000000000 ) ) ;
#64578=EDGE_CURVE ( 'NONE', #71601, #36015, #95736, .T. ) ;
#64580=VECTOR ( 'NONE', #54354, 1000.000000000000000 ) ;
#64587=EDGE_LOOP ( 'NONE', ( #18661, #201, #54260, #21260, #85716 ) ) ;
#64595=EDGE_LOOP ( 'NONE', ( #3250, #95881, #40096, #84643 ) ) ;
#64596=DIRECTION ( 'NONE',  ( 0.9999509640662961329, 0.009903002720634834083, 0.000000000000000000 ) ) ;
#64605=CARTESIAN_POINT ( 'NONE',  ( -7.079946287805722882, -69.52844923516938991, 3.749999999999999112 ) ) ;
#64606=SURFACE_STYLE_FILL_AREA ( #34114 ) ;
#64619=ORIENTED_EDGE ( 'NONE', *, *, #83673, .T. ) ;
#64621=DIRECTION ( 'NONE',  ( 1.000000000000000000, 0.000000000000000000, 0.000000000000000000 ) ) ;
#64637=EDGE_CURVE ( 'NONE', #2203, #70379, #78763, .T. ) ;
#64653=CARTESIAN_POINT ( 'NONE',  ( 4.380000000000000782, 1.019547802438464545, 2.750000000000000000 ) ) ;
#64662=ORIENTED_EDGE ( 'NONE', *, *, #81605, .F. ) ;
#64664=EDGE_CURVE ( 'NONE', #71742, #11450, #74703, .T. ) ;
#64667=CARTESIAN_POINT ( 'NONE',  ( -6.000000000000014211, 80.07179676972448590, 6.250000000000000000 ) ) ;
#64674=DIRECTION ( 'NONE',  ( -6.938893903907222067E-15, 0.000000000000000000, -1.000000000000000000 ) ) ;
#64687=FILL_AREA_STYLE_COLOUR ( '', #82685 ) ;
#64708=DIRECTION ( 'NONE',  ( -0.000000000000000000, 0.000000000000000000, 1.000000000000000000 ) ) ;
#64710=COLOUR_RGB ( '', 0.08235294, 0.09019608, 0.10196078) ;
#64713=STYLED_ITEM ( 'NONE', ( #59248 ), #49810 ) ;
#64726=FACE_OUTER_BOUND ( 'NONE', #66934, .T. ) ;
#64734=( GEOMETRIC_REPRESENTATION_CONTEXT ( 3 ) GLOBAL_UNCERTAINTY_ASSIGNED_CONTEXT ( ( #91109 ) ) GLOBAL_UNIT_ASSIGNED_CONTEXT ( ( #88551, #96070, #87566 ) ) REPRESENTATION_CONTEXT ( 'NONE', 'WORKASPACE' ) );
#64736=( BOUNDED_SURFACE ( )  B_SPLINE_SURFACE ( 3, 2, ( 
 ( #13546, #58542, #80567 ),
 ( #57069, #19078, #49553 ),
 ( #66546, #12557, #12062 ),
 ( #72553, #4582, #43539 ),
 ( #35552, #66041, #4084 ),
 ( #27550, #58044, #50556 ),
 ( #74035, #5565, #34549 ),
 ( #97074, #89543, #54005 ),
 ( #75028, #60519, #22541 ),
 ( #37044, #53013, #91010 ),
 ( #83032, #67542, #554 ),
 ( #90516, #29513, #98056 ),
 ( #16011, #38524, #60021 ),
 ( #22050, #52041, #44532 ),
 ( #15541, #82531, #30014 ),
 ( #38038, #69022, #83527 ),
 ( #84515, #52525, #14548 ),
 ( #45019, #15046, #77000 ),
 ( #45518, #68035, #75524 ),
 ( #90029, #14049, #7039 ),
 ( #29026, #91520, #46025 ),
 ( #76018, #37544, #7548 ) ),
 .UNSPECIFIED., .F., .F., .F. ) 
 B_SPLINE_SURFACE_WITH_KNOTS ( ( 4, 2, 2, 2, 2, 2, 2, 2, 2, 2, 4 ),
 ( 3, 3 ),
 ( 0.000000000000000000, 0.002789288213736775251, 0.005578576427473550502, 0.01115715285494710100, 0.02231430570989420201, 0.03347145856484130128, 0.04462861141978840401, 0.06694291712968260255, 0.07810006998462970529, 0.08367864641210326360, 0.08925722283957680803 ),
 ( 0.000000000000000000, 1.000000000000000000 ),
 .UNSPECIFIED. ) 
 GEOMETRIC_REPRESENTATION_ITEM ( )  RATIONAL_B_SPLINE_SURFACE ( (
 ( 1.000000000000000000, 0.7071067811865482389, 1.000000000000000000),
 ( 1.000000000000000000, 0.7071067811865482389, 1.000000000000000000),
 ( 1.000000000000000000, 0.7071067811865482389, 1.000000000000000000),
 ( 1.000000000000000000, 0.7071067811865482389, 1.000000000000000000),
 ( 1.000000000000000000, 0.7071067811865475727, 1.000000000000000000),
 ( 1.000000000000000000, 0.7071067811865475727, 1.000000000000000000),
 ( 1.000000000000000000, 0.7071067811865463515, 1.000000000000000000),
 ( 1.000000000000000000, 0.7071067811865463515, 1.000000000000000000),
 ( 1.000000000000000000, 0.7071067811865477948, 1.000000000000000000),
 ( 1.000000000000000000, 0.7071067811865477948, 1.000000000000000000),
 ( 1.000000000000000000, 0.7071067811865475727, 1.000000000000000000),
 ( 1.000000000000000000, 0.7071067811865475727, 1.000000000000000000),
 ( 1.000000000000000000, 0.7071067811865475727, 1.000000000000000000),
 ( 1.000000000000000000, 0.7071067811865475727, 1.000000000000000000),
 ( 1.000000000000000000, 0.7071067811865487940, 1.000000000000000000),
 ( 1.000000000000000000, 0.7071067811865487940, 1.000000000000000000),
 ( 1.000000000000000000, 0.7071067811865456854, 1.000000000000000000),
 ( 1.000000000000000000, 0.7071067811865456854, 1.000000000000000000),
 ( 1.000000000000000000, 0.7071067811865475727, 1.000000000000000000),
 ( 1.000000000000000000, 0.7071067811865475727, 1.000000000000000000),
 ( 1.000000000000000000, 0.7071067811865475727, 1.000000000000000000),
 ( 1.000000000000000000, 0.7071067811865475727, 1.000000000000000000) ) ) 
 REPRESENTATION_ITEM ( '' )  SURFACE ( )  );
#64738=CARTESIAN_POINT ( 'NONE',  ( -13.01808377376653247, 90.72591000949749684, 7.552080394870894331 ) ) ;
#64740=AXIS2_PLACEMENT_3D ( 'NONE', #36228, #27237, #35731 ) ;
#64751=SURFACE_STYLE_FILL_AREA ( #20262 ) ;
#64754=SURFACE_STYLE_FILL_AREA ( #49760 ) ;
#64756=EDGE_CURVE ( 'NONE', #11943, #96670, #25882, .T. ) ;
#64759=FACE_OUTER_BOUND ( 'NONE', #91795, .T. ) ;
#64765=CARTESIAN_POINT ( 'NONE',  ( -8.051923691749143686, 84.95650211105896688, -3.789018682291705797 ) ) ;
#64792=DIRECTION ( 'NONE',  ( -0.000000000000000000, -0.000000000000000000, 1.000000000000000000 ) ) ;
#64802=EDGE_LOOP ( 'NONE', ( #84039, #14081, #65575, #18029 ) ) ;
#64809=ORIENTED_EDGE ( 'NONE', *, *, #90170, .F. ) ;
#64810=CIRCLE ( 'NONE', #63178, 10.65000000000026326 ) ;
#64822=ORIENTED_EDGE ( 'NONE', *, *, #17762, .T. ) ;
#64824=ORIENTED_EDGE ( 'NONE', *, *, #76713, .F. ) ;
#64836=ORIENTED_EDGE ( 'NONE', *, *, #44571, .F. ) ;
#64847=DIRECTION ( 'NONE',  ( 1.000000000000000000, 0.000000000000000000, 0.000000000000000000 ) ) ;
#64849=CARTESIAN_POINT ( 'NONE',  ( -7.750000000000000000, 40.74999999999999289, -3.750000000000000000 ) ) ;
#64852=DIRECTION ( 'NONE',  ( -1.257402221000611116E-16, 1.000000000000000000, 0.000000000000000000 ) ) ;
#64858=SURFACE_STYLE_USAGE ( .BOTH. , #43839 ) ;
#64868=DIRECTION ( 'NONE',  ( 0.000000000000000000, 0.000000000000000000, 1.000000000000000000 ) ) ;
#64871=CARTESIAN_POINT ( 'NONE',  ( 11.29340449002647162, -89.90880494512830978, 3.750000000000000444 ) ) ;
#64887=CARTESIAN_POINT ( 'NONE',  ( 6.934035614004487869, -73.16521313705239038, -3.750000000000000000 ) ) ;
#64899=ORIENTED_EDGE ( 'NONE', *, *, #32843, .T. ) ;
#64901=DIRECTION ( 'NONE',  ( -0.000000000000000000, -1.000000000000000000, 0.000000000000000000 ) ) ;
#64904=( GEOMETRIC_REPRESENTATION_CONTEXT ( 3 ) GLOBAL_UNCERTAINTY_ASSIGNED_CONTEXT ( ( #2250 ) ) GLOBAL_UNIT_ASSIGNED_CONTEXT ( ( #55656, #46665, #54162 ) ) REPRESENTATION_CONTEXT ( 'NONE', 'WORKASPACE' ) );
#64912=LINE ( 'NONE', #2000, #44862 ) ;
#64915=DIRECTION ( 'NONE',  ( 0.8070303256584299145, -0.5905099943842175847, 0.000000000000000000 ) ) ;
#64922=AXIS2_PLACEMENT_3D ( 'NONE', #64958, #16661, #77633 ) ;
#64925=DIRECTION ( 'NONE',  ( -0.000000000000000000, -1.000000000000000000, -0.000000000000000000 ) ) ;
#64927=ORIENTED_EDGE ( 'NONE', *, *, #94961, .F. ) ;
#64928=( GEOMETRIC_REPRESENTATION_CONTEXT ( 3 ) GLOBAL_UNCERTAINTY_ASSIGNED_CONTEXT ( ( #59126 ) ) GLOBAL_UNIT_ASSIGNED_CONTEXT ( ( #65581, #56623, #35082 ) ) REPRESENTATION_CONTEXT ( 'NONE', 'WORKASPACE' ) );
#64932=CARTESIAN_POINT ( 'NONE',  ( 4.380000000000002558, 1.019547802438462547, 3.750000000000000000 ) ) ;
#64953=DIRECTION ( 'NONE',  ( -1.927470528863119542E-16, 1.000000000000000000, 0.000000000000000000 ) ) ;
#64954=VECTOR ( 'NONE', #29202, 1000.000000000000000 ) ;
#64958=CARTESIAN_POINT ( 'NONE',  ( -3.750000000000000000, 10.25000000000000000, 2.750000000000000000 ) ) ;
#64962=ORIENTED_EDGE ( 'NONE', *, *, #1458, .F. ) ;
#64969=AXIS2_PLACEMENT_3D ( 'NONE', #71043, #89473, #49995 ) ;
#64973=EDGE_LOOP ( 'NONE', ( #17877, #63094, #34963, #48500 ) ) ;
#64978=VERTEX_POINT ( 'NONE', #59694 ) ;
#64999=CARTESIAN_POINT ( 'NONE',  ( 4.219999999999999751, 10.00000000000000000, 2.750000000000000000 ) ) ;
#65001=STYLED_ITEM ( 'NONE', ( #10828 ), #30076 ) ;
#65009=CARTESIAN_POINT ( 'NONE',  ( -6.866275848337627608, -80.67678253189124860, -2.500000000000000000 ) ) ;
#65012=( LENGTH_UNIT ( ) NAMED_UNIT ( * ) SI_UNIT ( .MILLI., .METRE. ) );
#65026=( NAMED_UNIT ( * ) PLANE_ANGLE_UNIT ( ) SI_UNIT ( $, .RADIAN. ) );
#65042=TOROIDAL_SURFACE ( 'NONE', #33083, 0.7500000000000008882, 0.2500000000000000000 ) ;
#65044=DIRECTION ( 'NONE',  ( -0.06975647374412544122, -0.9975640502598241977, 0.000000000000000000 ) ) ;
#65045=STYLED_ITEM ( 'NONE', ( #29766 ), #68884 ) ;
#65056=PRESENTATION_STYLE_ASSIGNMENT (( #64074 ) ) ;
#65063=SPHERICAL_SURFACE ( 'NONE', #92398, 0.2500000000000000000 ) ;
#65071=ADVANCED_FACE ( 'NONE', ( #2691 ), #71166, .T. ) ;
#65086=CYLINDRICAL_SURFACE ( 'NONE', #52132, 6.349999999999995204 ) ;
#65087=CIRCLE ( 'NONE', #82676, 1.249999999999987121 ) ;
#65091=CARTESIAN_POINT ( 'NONE',  ( 11.40632860308399366, -69.21585191270298765, 4.000000000000000000 ) ) ;
#65095=ADVANCED_FACE ( 'NONE', ( #18163 ), #75356, .F. ) ;
#65097=STYLED_ITEM ( 'NONE', ( #28186 ), #11973 ) ;
#65098=VERTEX_POINT ( 'NONE', #45083 ) ;
#65099=DIRECTION ( 'NONE',  ( 0.000000000000000000, -0.000000000000000000, -1.000000000000000000 ) ) ;
#65104=CARTESIAN_POINT ( 'NONE',  ( -3.750000000000000888, 1.019547802438465212, 4.000000000000000000 ) ) ;
#65115=CIRCLE ( 'NONE', #90682, 0.2500000000000002220 ) ;
#65125=DIRECTION ( 'NONE',  ( 0.000000000000000000, 0.000000000000000000, -1.000000000000000000 ) ) ;
#65127=CARTESIAN_POINT ( 'NONE',  ( -6.000000000000014211, 80.07179676972448590, -6.500000000000000888 ) ) ;
#65133=CARTESIAN_POINT ( 'NONE',  ( 14.99999999999997691, 80.32179676972448590, 4.250000000000000000 ) ) ;
#65135=DIRECTION ( 'NONE',  ( 0.000000000000000000, -0.000000000000000000, 1.000000000000000000 ) ) ;
#65148=UNCERTAINTY_MEASURE_WITH_UNIT (LENGTH_MEASURE( 1.000000000000000082E-05 ), #87270, 'distance_accuracy_value', 'NONE');
#65163=FACE_OUTER_BOUND ( 'NONE', #24394, .T. ) ;
#65164=ORIENTED_EDGE ( 'NONE', *, *, #52775, .T. ) ;
#65167=ORIENTED_EDGE ( 'NONE', *, *, #73729, .F. ) ;
#65181=SPHERICAL_SURFACE ( 'NONE', #73109, 0.2500000000000000000 ) ;
#65182=AXIS2_PLACEMENT_3D ( 'NONE', #52905, #61881, #54379 ) ;
#65184=EDGE_LOOP ( 'NONE', ( #48121, #51622, #41632, #40021 ) ) ;
#65194=AXIS2_PLACEMENT_3D ( 'NONE', #58055, #27563, #20065 ) ;
#65197=VERTEX_POINT ( 'NONE', #35614 ) ;
#65212=DIRECTION ( 'NONE',  ( 1.000000000000000000, 0.000000000000000000, -0.000000000000000000 ) ) ;
#65218=PLANE ( 'NONE',  #60191 ) ;
#65223=SURFACE_SIDE_STYLE ('',( #34732 ) ) ;
#65232=CARTESIAN_POINT ( 'NONE',  ( -11.21074626900200677, 89.89919991260448739, 6.510369878059174553 ) ) ;
#65260=CYLINDRICAL_SURFACE ( 'NONE', #85522, 2.000000000000001776 ) ;
#65276=CARTESIAN_POINT ( 'NONE',  ( -7.750000000000000000, 0.000000000000000000, -3.750000000000000000 ) ) ;
#65277=( NAMED_UNIT ( * ) SI_UNIT ( $, .STERADIAN. ) SOLID_ANGLE_UNIT ( ) );
#65280=CIRCLE ( 'NONE', #9414, 10.09999999999999787 ) ;
#65291=DIRECTION ( 'NONE',  ( 1.000000000000000000, 2.569960705150826877E-16, -0.000000000000000000 ) ) ;
#65295=CARTESIAN_POINT ( 'NONE',  ( -5.999999999999994671, 43.00000000000000000, 6.500000000000000888 ) ) ;
#65299=DIRECTION ( 'NONE',  ( 0.000000000000000000, 0.000000000000000000, 1.000000000000000000 ) ) ;
#65303=ORIENTED_EDGE ( 'NONE', *, *, #4857, .T. ) ;
#65306=FACE_OUTER_BOUND ( 'NONE', #12022, .T. ) ;
#65307=VERTEX_POINT ( 'NONE', #75588 ) ;
#65335=ORIENTED_EDGE ( 'NONE', *, *, #45830, .T. ) ;
#65340=DIRECTION ( 'NONE',  ( 0.000000000000000000, 0.000000000000000000, 1.000000000000000000 ) ) ;
#65354=( LENGTH_UNIT ( ) NAMED_UNIT ( * ) SI_UNIT ( .MILLI., .METRE. ) );
#65358=CARTESIAN_POINT ( 'NONE',  ( -3.999999999999994671, 43.00000000000000711, 4.250000000000000000 ) ) ;
#65373=ORIENTED_EDGE ( 'NONE', *, *, #95318, .F. ) ;
#65392=DIRECTION ( 'NONE',  ( -1.000000000000000000, 0.000000000000000000, -0.000000000000000000 ) ) ;
#65399=DIRECTION ( 'NONE',  ( 1.000000000000000000, 0.000000000000000000, 0.000000000000000000 ) ) ;
#65404=DIRECTION ( 'NONE',  ( 0.000000000000000000, -0.000000000000000000, -1.000000000000000000 ) ) ;
#65407=DIRECTION ( 'NONE',  ( 0.000000000000000000, 0.000000000000000000, -1.000000000000000000 ) ) ;
#65455=CARTESIAN_POINT ( 'NONE',  ( 14.99999999999998046, 79.82179676972448590, -6.250000000000000000 ) ) ;
#65460=CARTESIAN_POINT ( 'NONE',  ( -8.000000000000000000, 80.07179676972448590, 6.500000000000000888 ) ) ;
#65481=UNCERTAINTY_MEASURE_WITH_UNIT (LENGTH_MEASURE( 1.000000000000000082E-05 ), #35171, 'distance_accuracy_value', 'NONE');
#65490=CARTESIAN_POINT ( 'NONE',  ( -4.000000000000000000, 78.07179676972445748, -4.250000000000000000 ) ) ;
#65511=CYLINDRICAL_SURFACE ( 'NONE', #15122, 0.2500000000000002220 ) ;
#65523=CARTESIAN_POINT ( 'NONE',  ( 17.97400638239511750, 77.67876782659151047, -4.131022355321664286 ) ) ;
#65529=DIRECTION ( 'NONE',  ( 1.000000000000000000, -0.000000000000000000, -0.000000000000000000 ) ) ;
#65546=EDGE_LOOP ( 'NONE', ( #18160, #53566, #70981, #57332 ) ) ;
#65550=CARTESIAN_POINT ( 'NONE',  ( -13.73866367547691958, 90.95360148970608805, 7.920681552399385872 ) ) ;
#65556=AXIS2_PLACEMENT_3D ( 'NONE', #98040, #13027, #66527 ) ;
#65570=EDGE_CURVE ( 'NONE', #40043, #538, #20913, .T. ) ;
#65572=ORIENTED_EDGE ( 'NONE', *, *, #95766, .T. ) ;
#65575=ORIENTED_EDGE ( 'NONE', *, *, #4652, .F. ) ;
#65581=( LENGTH_UNIT ( ) NAMED_UNIT ( * ) SI_UNIT ( .MILLI., .METRE. ) );
#65583=VECTOR ( 'NONE', #86560, 1000.000000000000000 ) ;
#65585=DIRECTION ( 'NONE',  ( -0.000000000000000000, -0.000000000000000000, -1.000000000000000000 ) ) ;
#65594=DIRECTION ( 'NONE',  ( -0.000000000000000000, 1.000000000000000000, 0.000000000000000000 ) ) ;
#65596=CARTESIAN_POINT ( 'NONE',  ( -3.499999999999998668, 1.019547802438465434, 3.750000000000000000 ) ) ;
#65612=AXIS2_PLACEMENT_3D ( 'NONE', #80539, #95544, #43515 ) ;
#65613=ORIENTED_EDGE ( 'NONE', *, *, #69598, .F. ) ;
#65620=CARTESIAN_POINT ( 'NONE',  ( 1.379999999999981908, 20.99999999999999645, 0.000000000000000000 ) ) ;
#65623=DIRECTION ( 'NONE',  ( -1.483861936729427615E-16, 1.000000000000000000, 0.000000000000000000 ) ) ;
#65629=CARTESIAN_POINT ( 'NONE',  ( -11.17367748615327372, -90.30033005415631919, -4.000000000000000000 ) ) ;
#65631=LINE ( 'NONE', #72152, #63938 ) ;
#65634=EDGE_CURVE ( 'NONE', #48124, #10040, #61121, .T. ) ;
#65647=EDGE_CURVE ( 'NONE', #8190, #30537, #14830, .T. ) ;
#65648=CARTESIAN_POINT ( 'NONE',  ( 17.99999999999999645, 91.28723161455539525, -8.000000000000000000 ) ) ;
#65649=CARTESIAN_POINT ( 'NONE',  ( 6.673414917871782315, -55.62670566514463388, 3.750000000000001776 ) ) ;
#65660=DIRECTION ( 'NONE',  ( 1.000000000000000000, 0.000000000000000000, 0.000000000000000000 ) ) ;
#65663=ORIENTED_EDGE ( 'NONE', *, *, #82988, .F. ) ;
#65664=CIRCLE ( 'NONE', #9730, 0.5000000000000004441 ) ;
#65672=CARTESIAN_POINT ( 'NONE',  ( -10.60846096436510422, -98.07574024450978811, 4.000000000000000000 ) ) ;
#65679=DIRECTION ( 'NONE',  ( 0.000000000000000000, 0.000000000000000000, -1.000000000000000000 ) ) ;
#65681=EDGE_LOOP ( 'NONE', ( #83786, #68294, #48787, #17639 ) ) ;
#65682=DIRECTION ( 'NONE',  ( -0.000000000000000000, -1.000000000000000000, 0.000000000000000000 ) ) ;
#65703=MECHANICAL_DESIGN_GEOMETRIC_PRESENTATION_REPRESENTATION('',(#89625),#78500);
#65706=CARTESIAN_POINT ( 'NONE',  ( -8.000000000000000000, 40.99999999999999289, -6.250000000000000000 ) ) ;
#65710=DIRECTION ( 'NONE',  ( 0.000000000000000000, 0.000000000000000000, -1.000000000000000000 ) ) ;
#65722=FACE_OUTER_BOUND ( 'NONE', #64802, .T. ) ;
#65723=( NAMED_UNIT ( * ) PLANE_ANGLE_UNIT ( ) SI_UNIT ( $, .RADIAN. ) );
#65726=FACE_OUTER_BOUND ( 'NONE', #75267, .T. ) ;
#65732=CARTESIAN_POINT ( 'NONE',  ( -11.93818897418494984, 90.30657785595315090, 6.860068911468413688 ) ) ;
#65760=CARTESIAN_POINT ( 'NONE',  ( -13.42719148503548610, 90.83520141667820269, -7.724461209138739903 ) ) ;
#65762=DIRECTION ( 'NONE',  ( 1.000000000000000000, 0.000000000000000000, 0.000000000000000000 ) ) ;
#65767=DIRECTION ( 'NONE',  ( 1.000000000000000000, -0.000000000000000000, -0.000000000000000000 ) ) ;
#65792=DIRECTION ( 'NONE',  ( 1.000000000000000000, 0.000000000000000000, 0.000000000000000000 ) ) ;
#65806=CARTESIAN_POINT ( 'NONE',  ( 6.432108699068923130, -88.20011490510430008, 3.750000000000000000 ) ) ;
#65809=VECTOR ( 'NONE', #81067, 1000.000000000000000 ) ;
#65815=EDGE_LOOP ( 'NONE', ( #98581, #58558, #82242, #95273 ) ) ;
#65822=CARTESIAN_POINT ( 'NONE',  ( -14.89999999999999680, 98.49999999999998579, 8.000000000000000000 ) ) ;
#65852=CARTESIAN_POINT ( 'NONE',  ( 9.779999999999990479, 20.99999999999999645, 0.000000000000000000 ) ) ;
#65858=CARTESIAN_POINT ( 'NONE',  ( 4.630000000000003446, 1.019547802438462547, -4.000000000000000000 ) ) ;
#65869=ORIENTED_EDGE ( 'NONE', *, *, #50727, .F. ) ;
#65871=PRESENTATION_STYLE_ASSIGNMENT (( #27874 ) ) ;
#65872=DIRECTION ( 'NONE',  ( -0.000000000000000000, 0.000000000000000000, 1.000000000000000000 ) ) ;
#65875=CIRCLE ( 'NONE', #25928, 0.2500000000000002220 ) ;
#65878=CARTESIAN_POINT ( 'NONE',  ( 8.879999999999991900, 21.00000000000000000, 0.000000000000000000 ) ) ;
#65886=CARTESIAN_POINT ( 'NONE',  ( 7.155633850256548634, -69.45312897839663435, -4.000000000000000000 ) ) ;
#65887=CARTESIAN_POINT ( 'NONE',  ( -11.17367748577515130, -90.30033005412217051, -3.999999999999999112 ) ) ;
#65899=LINE ( 'NONE', #34910, #1420 ) ;
#65910=CARTESIAN_POINT ( 'NONE',  ( 8.879999999999991900, 76.07179676972447169, 4.250000000000000000 ) ) ;
#65913=DIRECTION ( 'NONE',  ( 0.08715574274765114371, 0.9961946980917462113, 0.000000000000000000 ) ) ;
#65916=CIRCLE ( 'NONE', #27586, 3.000000000000000888 ) ;
#65920=AXIS2_PLACEMENT_3D ( 'NONE', #95276, #25336, #18309 ) ;
#65927=ADVANCED_FACE ( 'NONE', ( #55338 ), #77834, .T. ) ;
#65928=CARTESIAN_POINT ( 'NONE',  ( -3.750000000000000000, 10.00000000000000000, -3.750000000000000000 ) ) ;
#65929=CARTESIAN_POINT ( 'NONE',  ( -6.000000000000009770, 41.24999999999999289, 6.500000000000000888 ) ) ;
#65931=DIRECTION ( 'NONE',  ( -1.000000000000000000, 0.000000000000000000, 0.000000000000000000 ) ) ;
#65954=ORIENTED_EDGE ( 'NONE', *, *, #93876, .T. ) ;
#65980=MECHANICAL_DESIGN_GEOMETRIC_PRESENTATION_REPRESENTATION('',(#64335),#22910);
#65983=DIRECTION ( 'NONE',  ( 0.000000000000000000, 0.000000000000000000, -1.000000000000000000 ) ) ;
#65994=PRESENTATION_STYLE_ASSIGNMENT (( #12506 ) ) ;
#65999=ORIENTED_EDGE ( 'NONE', *, *, #90170, .T. ) ;
#66000=SURFACE_STYLE_USAGE ( .BOTH. , #1713 ) ;
#66011=SURFACE_STYLE_USAGE ( .BOTH. , #23620 ) ;
#66013=CARTESIAN_POINT ( 'NONE',  ( -13.11254139118232231, 91.00000000000000000, -8.000000000000000000 ) ) ;
#66015=ADVANCED_FACE ( 'NONE', ( #77342 ), #38876, .T. ) ;
#66016=ADVANCED_FACE ( 'NONE', ( #4315 ), #62759, .T. ) ;
#66021=CARTESIAN_POINT ( 'NONE',  ( 18.00000000000000000, 77.07179676972447169, -4.250000000000000000 ) ) ;
#66041=CARTESIAN_POINT ( 'NONE',  ( -3.628626192036342069, -3.642031182891574126, -4.000000000000000000 ) ) ;
#66043=ORIENTED_EDGE ( 'NONE', *, *, #69638, .F. ) ;
#66049=CARTESIAN_POINT ( 'NONE',  ( -9.000000000000003553, 80.99999999999994316, 1.249999999999987121 ) ) ;
#66051=CARTESIAN_POINT ( 'NONE',  ( -4.249999999999999112, 78.07179676972445748, 6.500000000000000888 ) ) ;
#66054=CARTESIAN_POINT ( 'NONE',  ( 3.969999999999999751, 10.25000000000000000, -2.500000000000000000 ) ) ;
#66061=SURFACE_STYLE_USAGE ( .BOTH. , #11590 ) ;
#66067=DIRECTION ( 'NONE',  ( 1.000000000000000000, 0.000000000000000000, 0.000000000000000000 ) ) ;
#66080=FACE_OUTER_BOUND ( 'NONE', #55725, .T. ) ;
#66082=CARTESIAN_POINT ( 'NONE',  ( 4.219999999999999751, 36.75000000000000000, 3.750000000000000000 ) ) ;
#66090=ORIENTED_EDGE ( 'NONE', *, *, #65634, .F. ) ;
#66091=FILL_AREA_STYLE_COLOUR ( '', #89179 ) ;
#66097=ORIENTED_EDGE ( 'NONE', *, *, #82546, .T. ) ;
#66103=DIRECTION ( 'NONE',  ( 0.8070303256584298035, -0.5905099943842175847, 0.000000000000000000 ) ) ;
#66115=FACE_BOUND ( 'NONE', #80822, .T. ) ;
#66124=CARTESIAN_POINT ( 'NONE',  ( -11.51381718487224681, -65.37259455511993167, -3.750000000000000000 ) ) ;
#66140=CARTESIAN_POINT ( 'NONE',  ( 17.97713247904330558, 91.14635076194878138, -8.000000000000000000 ) ) ;
#66148=DIRECTION ( 'NONE',  ( 1.000000000000000000, 0.000000000000000000, 0.000000000000000000 ) ) ;
#66151=DIRECTION ( 'NONE',  ( -0.000000000000000000, 1.000000000000000000, -0.000000000000000000 ) ) ;
#66154=EDGE_LOOP ( 'NONE', ( #45038, #24554, #6346, #94034 ) ) ;
#66163=CARTESIAN_POINT ( 'NONE',  ( -16.80847703285585482, 99.89644660940670917, 8.000000000000001776 ) ) ;
#66176=ORIENTED_EDGE ( 'NONE', *, *, #73827, .F. ) ;
#66182=COLOUR_RGB ( '', 0.31764706, 0.68627451, 0.89019608) ;
#66183=VECTOR ( 'NONE', #86919, 1000.000000000000000 ) ;
#66187=STYLED_ITEM ( 'NONE', ( #31570 ), #95230 ) ;
#66197=FACE_OUTER_BOUND ( 'NONE', #12665, .T. ) ;
#66204=DIRECTION ( 'NONE',  ( 1.000000000000000000, 0.000000000000000000, 0.000000000000000000 ) ) ;
#66209=EDGE_CURVE ( 'NONE', #26872, #62733, #71818, .T. ) ;
#66212=CARTESIAN_POINT ( 'NONE',  ( 14.99999999999997868, 80.07179676972448590, 6.500000000000000888 ) ) ;
#66216=CARTESIAN_POINT ( 'NONE',  ( -4.250000000000000000, 10.00000000000000000, -4.000000000000000000 ) ) ;
#66217=SURFACE_SIDE_STYLE ('',( #8565 ) ) ;
#66227=ORIENTED_EDGE ( 'NONE', *, *, #62783, .T. ) ;
#66232=FACE_OUTER_BOUND ( 'NONE', #10855, .T. ) ;
#66247=ORIENTED_EDGE ( 'NONE', *, *, #68773, .F. ) ;
#66252=CARTESIAN_POINT ( 'NONE',  ( -11.21074626900200677, 89.89919991260448739, -6.510369878059174553 ) ) ;
#66265=DIRECTION ( 'NONE',  ( -0.000000000000000000, -0.000000000000000000, 1.000000000000000000 ) ) ;
#66270=SURFACE_SIDE_STYLE ('',( #60259 ) ) ;
#66276=FACE_OUTER_BOUND ( 'NONE', #71537, .T. ) ;
#66302=CARTESIAN_POINT ( 'NONE',  ( -3.499999999999998668, 1.019547802438465434, -2.500000000000000000 ) ) ;
#66305=ORIENTED_EDGE ( 'NONE', *, *, #42164, .F. ) ;
#66315=DIRECTION ( 'NONE',  ( -1.000000000000000000, -0.000000000000000000, -0.000000000000000000 ) ) ;
#66319=VECTOR ( 'NONE', #49083, 1000.000000000000114 ) ;
#66320=ORIENTED_EDGE ( 'NONE', *, *, #96097, .F. ) ;
#66347=ADVANCED_FACE ( 'NONE', ( #7772 ), #6277, .T. ) ;
#66350=DIRECTION ( 'NONE',  ( 0.6038238647437427220, -0.7971177707001206869, 0.000000000000000000 ) ) ;
#66364=CARTESIAN_POINT ( 'NONE',  ( 7.079515573063599021, -88.00917032380691296, -4.000000000000000000 ) ) ;
#66367=CARTESIAN_POINT ( 'NONE',  ( -9.886043635230025828, 89.00072246145502675, 5.688751881067944716 ) ) ;
#66369=AXIS2_PLACEMENT_3D ( 'NONE', #56343, #10348, #40848 ) ;
#66372=ADVANCED_FACE ( 'NONE', ( #74769 ), #67274, .T. ) ;
#66375=CARTESIAN_POINT ( 'NONE',  ( -8.000000000000000000, 80.99999999999994316, 0.000000000000000000 ) ) ;
#66388=FACE_OUTER_BOUND ( 'NONE', #96088, .T. ) ;
#66397=AXIS2_PLACEMENT_3D ( 'NONE', #14427, #5933, #98437 ) ;
#66398=UNCERTAINTY_MEASURE_WITH_UNIT (LENGTH_MEASURE( 1.000000000000000082E-05 ), #75256, 'distance_accuracy_value', 'NONE');
#66399=AXIS2_PLACEMENT_3D ( 'NONE', #64321, #93358, #94832 ) ;
#66402=EDGE_CURVE ( 'NONE', #76544, #19964, #30363, .T. ) ;
#66403=DIRECTION ( 'NONE',  ( 1.000000000000000000, 0.000000000000000000, 0.000000000000000000 ) ) ;
#66425=PLANE ( 'NONE',  #36110 ) ;
#66444=AXIS2_PLACEMENT_3D ( 'NONE', #49148, #72618, #58612 ) ;
#66457=AXIS2_PLACEMENT_3D ( 'NONE', #51251, #68731, #75231 ) ;
#66465=AXIS2_PLACEMENT_3D ( 'NONE', #89247, #49756, #43740 ) ;
#66470=CARTESIAN_POINT ( 'NONE',  ( 4.906773990575423738, -8.256880746075376365, 3.999999999999999112 ) ) ;
#66475=UNCERTAINTY_MEASURE_WITH_UNIT (LENGTH_MEASURE( 1.000000000000000082E-05 ), #67377, 'distance_accuracy_value', 'NONE');
#66493=CARTESIAN_POINT ( 'NONE',  ( -6.581680125707231710, -88.31141629936868753, 3.750000000000000000 ) ) ;
#66500=ADVANCED_FACE ( 'NONE', ( #84742 ), #12810, .T. ) ;
#66502=ORIENTED_EDGE ( 'NONE', *, *, #92365, .T. ) ;
#66516=( NAMED_UNIT ( * ) PLANE_ANGLE_UNIT ( ) SI_UNIT ( $, .RADIAN. ) );
#66521=CIRCLE ( 'NONE', #69745, 6.599999999999995204 ) ;
#66527=DIRECTION ( 'NONE',  ( 0.000000000000000000, 2.602085213965208275E-15, -1.000000000000000000 ) ) ;
#66528=CARTESIAN_POINT ( 'NONE',  ( 9.879999999999990123, 20.99999999999999645, 0.000000000000000000 ) ) ;
#66533=EDGE_CURVE ( 'NONE', #10040, #35492, #22401, .T. ) ;
#66541=DIRECTION ( 'NONE',  ( -2.569960705150826877E-16, 1.000000000000000000, 0.000000000000000000 ) ) ;
#66545=CARTESIAN_POINT ( 'NONE',  ( 11.13575493849772258, -94.04002841299546844, -3.749999999999999556 ) ) ;
#66546=CARTESIAN_POINT ( 'NONE',  ( -3.522141228383032008, -0.8488377519105428926, -3.750000000000000000 ) ) ;
#66558=CARTESIAN_POINT ( 'NONE',  ( -10.09048698379360687, 46.92328126389585208, -2.900000000000000355 ) ) ;
#66564=ORIENTED_EDGE ( 'NONE', *, *, #54141, .F. ) ;
#66572=AXIS2_PLACEMENT_3D ( 'NONE', #91062, #7594, #22096 ) ;
#66573=AXIS2_PLACEMENT_3D ( 'NONE', #72069, #12058, #26565 ) ;
#66574=AXIS2_PLACEMENT_3D ( 'NONE', #72506, #49027, #33035 ) ;
#66577=ORIENTED_EDGE ( 'NONE', *, *, #11961, .T. ) ;
#66590=DIRECTION ( 'NONE',  ( 0.000000000000000000, 0.000000000000000000, -1.000000000000000000 ) ) ;
#66591=ORIENTED_EDGE ( 'NONE', *, *, #44311, .T. ) ;
#66596=STYLED_ITEM ( 'NONE', ( #17421 ), #30369 ) ;
#66598=ORIENTED_EDGE ( 'NONE', *, *, #46303, .T. ) ;
#66601=PRESENTATION_STYLE_ASSIGNMENT (( #57610 ) ) ;
#66614=EDGE_CURVE ( 'NONE', #70343, #44664, #25610, .T. ) ;
#66615=ORIENTED_EDGE ( 'NONE', *, *, #87848, .F. ) ;
#66631=CARTESIAN_POINT ( 'NONE',  ( 8.629999999999995453, 41.24999999999999289, 6.250000000000000000 ) ) ;
#66637=CIRCLE ( 'NONE', #84215, 10.90000000000026326 ) ;
#66661=CARTESIAN_POINT ( 'NONE',  ( 4.864290147400408770, -17.52197929146259270, 2.500000000000000444 ) ) ;
#66664=EDGE_LOOP ( 'NONE', ( #70214, #68949, #30177, #42234 ) ) ;
#66672=CARTESIAN_POINT ( 'NONE',  ( -11.01435017095933588, -93.41041245700012041, 4.000000000000000000 ) ) ;
#66679=DIRECTION ( 'NONE',  ( -1.000000000000000000, 0.000000000000000000, 0.000000000000000000 ) ) ;
#66682=VERTEX_POINT ( 'NONE', #48693 ) ;
#66690=AXIS2_PLACEMENT_3D ( 'NONE', #41609, #49089, #27558 ) ;
#66694=VERTEX_POINT ( 'NONE', #64173 ) ;
#66705=VECTOR ( 'NONE', #23850, 1000.000000000000000 ) ;
#66725=DIRECTION ( 'NONE',  ( -0.000000000000000000, 1.000000000000000000, 0.000000000000000000 ) ) ;
#66745=( LENGTH_UNIT ( ) NAMED_UNIT ( * ) SI_UNIT ( .MILLI., .METRE. ) );
#66754=ORIENTED_EDGE ( 'NONE', *, *, #1051, .F. ) ;
#66757=DIRECTION ( 'NONE',  ( 1.000000000000000000, 0.000000000000000000, 0.000000000000000000 ) ) ;
#66765=FILL_AREA_STYLE ('',( #34780 ) ) ;
#66774=SURFACE_SIDE_STYLE ('',( #49791 ) ) ;
#66781=STYLED_ITEM ( 'NONE', ( #93570 ), #58821 ) ;
#66783=ORIENTED_EDGE ( 'NONE', *, *, #84928, .F. ) ;
#66785=CARTESIAN_POINT ( 'NONE',  ( 4.219999999999999751, 37.00000000000000000, -3.750000000000000000 ) ) ;
#66790=CARTESIAN_POINT ( 'NONE',  ( 15.00000000000000000, 77.07179676972447169, 6.250000000000000000 ) ) ;
#66793=CARTESIAN_POINT ( 'NONE',  ( 6.579634127946608402, -87.99828267815712479, -2.500000000000000000 ) ) ;
#66797=ORIENTED_EDGE ( 'NONE', *, *, #71039, .F. ) ;
#66799=EDGE_LOOP ( 'NONE', ( #33348, #9465, #1311, #21726 ) ) ;
#66805=ORIENTED_EDGE ( 'NONE', *, *, #35235, .F. ) ;
#66821=AXIS2_PLACEMENT_3D ( 'NONE', #35930, #90397, #65931 ) ;
#66825=DIRECTION ( 'NONE',  ( 0.000000000000000000, 0.000000000000000000, 1.000000000000000000 ) ) ;
#66834=CARTESIAN_POINT ( 'NONE',  ( -4.250000000000000000, 78.07179676972445748, -6.500000000000000888 ) ) ;
#66838=COLOUR_RGB ( '', 0.09019608, 0.27058824, 0.51372549) ;
#66842=ORIENTED_EDGE ( 'NONE', *, *, #9045, .T. ) ;
#66844=DIRECTION ( 'NONE',  ( 0.000000000000000000, -0.000000000000000000, -1.000000000000000000 ) ) ;
#66853=EDGE_CURVE ( 'NONE', #24454, #93321, #87184, .T. ) ;
#66855=DIRECTION ( 'NONE',  ( 0.7971177707001174673, 0.6038238647437470519, -0.000000000000000000 ) ) ;
#66860=VECTOR ( 'NONE', #21213, 1000.000000000000000 ) ;
#66868=LINE ( 'NONE', #58869, #86631 ) ;
#66872=DIRECTION ( 'NONE',  ( 1.000000000000000000, 0.000000000000000000, 0.000000000000000000 ) ) ;
#66873=ORIENTED_EDGE ( 'NONE', *, *, #56818, .F. ) ;
#66910=CIRCLE ( 'NONE', #42993, 0.2500000000000002220 ) ;
#66915=COLOUR_RGB ( '', 0.40784314, 0.44705882, 0.49803922) ;
#66923=CARTESIAN_POINT ( 'NONE',  ( 4.380000000000000782, 0.08775168532224617013, 3.750000000000000000 ) ) ;
#66924=( NAMED_UNIT ( * ) PLANE_ANGLE_UNIT ( ) SI_UNIT ( $, .RADIAN. ) );
#66925=( LENGTH_UNIT ( ) NAMED_UNIT ( * ) SI_UNIT ( .MILLI., .METRE. ) );
#66930=LINE ( 'NONE', #29408, #58844 ) ;
#66934=EDGE_LOOP ( 'NONE', ( #43258, #63694, #11573, #19485 ) ) ;
#66949=EDGE_CURVE ( 'NONE', #16898, #44301, #50166, .T. ) ;
#66962=CARTESIAN_POINT ( 'NONE',  ( -6.787853370348936544, -86.25412202734867151, 2.500000000000000888 ) ) ;
#66965=CARTESIAN_POINT ( 'NONE',  ( 10.68821231714948539, -97.11200166802359490, 4.000000000000000000 ) ) ;
#66967=ORIENTED_EDGE ( 'NONE', *, *, #73798, .T. ) ;
#66981=CARTESIAN_POINT ( 'NONE',  ( 3.969999999999999751, 10.25000000000000000, 2.750000000000000000 ) ) ;
#66989=SURFACE_STYLE_FILL_AREA ( #82482 ) ;
#66996=ORIENTED_EDGE ( 'NONE', *, *, #60606, .F. ) ;
#67000=CARTESIAN_POINT ( 'NONE',  ( 0.000000000000000000, -97.00000000000000000, -2.500000000000000000 ) ) ;
#67006=AXIS2_PLACEMENT_3D ( 'NONE', #61843, #59873, #16360 ) ;
#67024=CARTESIAN_POINT ( 'NONE',  ( 17.82110031882830725, 91.00000000000001421, 8.000000000000001776 ) ) ;
#67027=ORIENTED_EDGE ( 'NONE', *, *, #76054, .T. ) ;
#67040=CARTESIAN_POINT ( 'NONE',  ( 9.113212362719171011, -7.248705549479112165, -3.749999999999999112 ) ) ;
#67041=SURFACE_SIDE_STYLE ('',( #44030 ) ) ;
#67047=SURFACE_STYLE_USAGE ( .BOTH. , #13052 ) ;
#67066=EDGE_CURVE ( 'NONE', #80552, #92371, #63900, .T. ) ;
#67079=FACE_OUTER_BOUND ( 'NONE', #37167, .T. ) ;
#67083=CARTESIAN_POINT ( 'NONE',  ( 8.879999999999991900, 27.04366094290857347, 2.900000000000000355 ) ) ;
#67084=COLOUR_RGB ( '', 0.31764706, 0.68627451, 0.89019608) ;
#67089=PLANE ( 'NONE',  #11672 ) ;
#67092=EDGE_LOOP ( 'NONE', ( #78737, #72896, #52639, #90650 ) ) ;
#67127=AXIS2_PLACEMENT_3D ( 'NONE', #28281, #75261, #75754 ) ;
#67162=DIRECTION ( 'NONE',  ( 0.000000000000000000, 0.000000000000000000, 1.000000000000000000 ) ) ;
#67170=AXIS2_PLACEMENT_3D ( 'NONE', #55065, #40080, #9087 ) ;
#67173=ORIENTED_EDGE ( 'NONE', *, *, #80208, .T. ) ;
#67177=MECHANICAL_DESIGN_GEOMETRIC_PRESENTATION_REPRESENTATION('',(#9814),#97536);
#67187=CIRCLE ( 'NONE', #16081, 9.999999999999998224 ) ;
#67212=AXIS2_PLACEMENT_3D ( 'NONE', #73771, #74765, #96303 ) ;
#67228=DIRECTION ( 'NONE',  ( -0.9975640502598243087, 0.06975647374412544122, 0.000000000000000000 ) ) ;
#67237=CARTESIAN_POINT ( 'NONE',  ( -8.000000000000000000, 80.32179676972448590, 3.750000000000000000 ) ) ;
#67246=CYLINDRICAL_SURFACE ( 'NONE', #56894, 0.2500000000000002220 ) ;
#67247=( GEOMETRIC_REPRESENTATION_CONTEXT ( 3 ) GLOBAL_UNCERTAINTY_ASSIGNED_CONTEXT ( ( #7132 ) ) GLOBAL_UNIT_ASSIGNED_CONTEXT ( ( #61334, #37378, #53846 ) ) REPRESENTATION_CONTEXT ( 'NONE', 'WORKASPACE' ) );
#67248=CARTESIAN_POINT ( 'NONE',  ( -6.000000000000009770, 41.24999999999999289, -6.500000000000000888 ) ) ;
#67253=ORIENTED_EDGE ( 'NONE', *, *, #40114, .T. ) ;
#67258=CARTESIAN_POINT ( 'NONE',  ( -13.01808377376649339, 90.72591000950063744, -7.552080394871468094 ) ) ;
#67264=CARTESIAN_POINT ( 'NONE',  ( 9.261738776797663775, -15.50721619310240662, -4.000000000000000000 ) ) ;
#67274=CYLINDRICAL_SURFACE ( 'NONE', #70360, 0.2500000000000002220 ) ;
#67279=VECTOR ( 'NONE', #32947, 1000.000000000000000 ) ;
#67280=ORIENTED_EDGE ( 'NONE', *, *, #31605, .T. ) ;
#67282=CARTESIAN_POINT ( 'NONE',  ( -5.999999999999994671, 43.00000000000000000, 4.000000000000000000 ) ) ;
#67291=MECHANICAL_DESIGN_GEOMETRIC_PRESENTATION_REPRESENTATION('',(#35366),#24184);
#67294=CARTESIAN_POINT ( 'NONE',  ( -4.021995598252596338, -6.415937870593706904, 4.000000000000000000 ) ) ;
#67302=ORIENTED_EDGE ( 'NONE', *, *, #46382, .T. ) ;
#67318=MECHANICAL_DESIGN_GEOMETRIC_PRESENTATION_REPRESENTATION('',(#22651),#80091);
#67329=DIRECTION ( 'NONE',  ( -1.257402221000611116E-16, 1.000000000000000000, 0.000000000000000000 ) ) ;
#67341=CARTESIAN_POINT ( 'NONE',  ( 0.000000000000000000, 0.000000000000000000, 0.000000000000000000 ) ) ;
#67345=CARTESIAN_POINT ( 'NONE',  ( 6.660444548080930893, -84.28805632650643531, -2.500000000000001332 ) ) ;
#67355=FACE_OUTER_BOUND ( 'NONE', #18648, .T. ) ;
#67362=CARTESIAN_POINT ( 'NONE',  ( 10.83696084481538691, -98.17058944465519232, -3.750000000000000000 ) ) ;
#67363=DIRECTION ( 'NONE',  ( 1.000000000000000000, 0.000000000000000000, 0.000000000000000000 ) ) ;
#67377=( LENGTH_UNIT ( ) NAMED_UNIT ( * ) SI_UNIT ( .MILLI., .METRE. ) );
#67415=AXIS2_PLACEMENT_3D ( 'NONE', #19238, #65212, #65710 ) ;
#67419=DIRECTION ( 'NONE',  ( -1.000000000000000000, 0.000000000000000000, 0.000000000000000000 ) ) ;
#67422=LINE ( 'NONE', #52416, #1406 ) ;
#67425=DIRECTION ( 'NONE',  ( 0.000000000000000000, 0.000000000000000000, 1.000000000000000000 ) ) ;
#67429=VECTOR ( 'NONE', #29086, 1000.000000000000000 ) ;
#67433=ORIENTED_EDGE ( 'NONE', *, *, #59118, .T. ) ;
#67437=AXIS2_PLACEMENT_3D ( 'NONE', #68978, #70451, #92935 ) ;
#67440=DIRECTION ( 'NONE',  ( -1.000000000000000000, 0.000000000000000000, 0.000000000000000000 ) ) ;
#67442=FACE_OUTER_BOUND ( 'NONE', #3480, .T. ) ;
#67453=VERTEX_POINT ( 'NONE', #70112 ) ;
#67458=CARTESIAN_POINT ( 'NONE',  ( -7.079903288604985079, -69.52484394646408816, 2.500000000000000000 ) ) ;
#67464=VERTEX_POINT ( 'NONE', #1637 ) ;
#67466=AXIS2_PLACEMENT_3D ( 'NONE', #89451, #73449, #13450 ) ;
#67472=CARTESIAN_POINT ( 'NONE',  ( -8.000343251535921851, 84.06932101904432386, 3.750000000000000000 ) ) ;
#67479=CARTESIAN_POINT ( 'NONE',  ( 6.903457398626329677, -84.61157762779829739, -2.750000000000000000 ) ) ;
#67494=VERTEX_POINT ( 'NONE', #46130 ) ;
#67515=DIRECTION ( 'NONE',  ( 0.000000000000000000, 1.000000000000000000, 0.000000000000000000 ) ) ;
#67519=ADVANCED_FACE ( 'NONE', ( #77107 ), #54107, .F. ) ;
#67523=CARTESIAN_POINT ( 'NONE',  ( 17.97699586832901986, 91.14602379785867470, 8.000000000000000000 ) ) ;
#67524=( NAMED_UNIT ( * ) PLANE_ANGLE_UNIT ( ) SI_UNIT ( $, .RADIAN. ) );
#67534=LINE ( 'NONE', #45011, #19453 ) ;
#67541=CARTESIAN_POINT ( 'NONE',  ( 11.44532407938881136, -77.50611495452966437, -3.750000000000000000 ) ) ;
#67542=CARTESIAN_POINT ( 'NONE',  ( -5.331138373842556177, -28.69357394138843986, -4.000000000001612932 ) ) ;
#67543=ORIENTED_EDGE ( 'NONE', *, *, #13905, .T. ) ;
#67550=CARTESIAN_POINT ( 'NONE',  ( 8.879999999999991900, 20.99999999999999645, 0.000000000000000000 ) ) ;
#67551=CARTESIAN_POINT ( 'NONE',  ( -8.854007681965594401, 87.37522428062922586, -4.483348028979307287 ) ) ;
#67556=FACE_OUTER_BOUND ( 'NONE', #63362, .T. ) ;
#67561=ORIENTED_EDGE ( 'NONE', *, *, #88395, .F. ) ;
#67574=ORIENTED_EDGE ( 'NONE', *, *, #17170, .T. ) ;
#67582=VERTEX_POINT ( 'NONE', #73043 ) ;
#67589=EDGE_CURVE ( 'NONE', #86221, #8055, #69790, .T. ) ;
#67590=CARTESIAN_POINT ( 'NONE',  ( 9.261744320279156284, -15.50732398184426764, 3.999999999999999112 ) ) ;
#67594=( NAMED_UNIT ( * ) SI_UNIT ( $, .STERADIAN. ) SOLID_ANGLE_UNIT ( ) );
#67613=AXIS2_PLACEMENT_3D ( 'NONE', #6957, #21467, #69426 ) ;
#67614=ORIENTED_EDGE ( 'NONE', *, *, #13242, .F. ) ;
#67620=CARTESIAN_POINT ( 'NONE',  ( -3.711005778769052021, -5.293034685380286319, -2.750000000000000444 ) ) ;
#67629=FACE_OUTER_BOUND ( 'NONE', #48611, .T. ) ;
#67633=CARTESIAN_POINT ( 'NONE',  ( 8.879999999999999005, 20.99999999999999645, 0.000000000000000000 ) ) ;
#67639=VECTOR ( 'NONE', #16354, 1000.000000000000000 ) ;
#67649=DIRECTION ( 'NONE',  ( 0.8070303256584299145, -0.5905099943842175847, 0.000000000000000000 ) ) ;
#67662=DIRECTION ( 'NONE',  ( 1.000000000000000000, 0.000000000000000000, 0.000000000000000000 ) ) ;
#67669=CARTESIAN_POINT ( 'NONE',  ( -8.081444665679372363, -7.288330178580077146, 4.000000000000000000 ) ) ;
#67682=FILL_AREA_STYLE ('',( #35313 ) ) ;
#67722=CARTESIAN_POINT ( 'NONE',  ( -3.750000000000000000, 10.00000000000000000, 2.500000000000000000 ) ) ;
#67725=EDGE_CURVE ( 'NONE', #40043, #30756, #37901, .T. ) ;
#67729=CARTESIAN_POINT ( 'NONE',  ( 8.879999999999991900, 20.99999999999999645, -1.249999999999987121 ) ) ;
#67730=B_SPLINE_CURVE_WITH_KNOTS ( 'NONE', 3,
 ( #17998, #80462, #87951, #78493, #25988, #48480, #40509, #10007, #86971, #32983, #63485, #10489, #3491, #93989, #41000, #71499, #49957, #56962, #33461, #63958, #18484, #87463, #18978, #49457, #79962, #11466, #35935, #5947, #36437, #14437 ),
 .UNSPECIFIED., .F., .F.,
 ( 4, 2, 2, 2, 2, 2, 2, 2, 2, 2, 2, 2, 2, 2, 4 ),
 ( -6.000000000268970806E-08, 0.003118256826059614614, 0.006236573652119231474, 0.01247320730423846606, 0.02494647460847693524, 0.03741974191271540962, 0.04989300921695387359, 0.06236627652119233756, 0.07483954382543078765, 0.08107617747755001270, 0.08731281112966925162, 0.09354944478178846279, 0.09666776160784808225, 0.09822692002087787810, 0.09978607843390764620 ),
 .UNSPECIFIED. ) ;
#67738=LINE ( 'NONE', #62175, #44356 ) ;
#67749=DIRECTION ( 'NONE',  ( -1.000000000000000000, 0.000000000000000000, 0.000000000000000000 ) ) ;
#67753=ORIENTED_EDGE ( 'NONE', *, *, #74466, .T. ) ;
#67758=CARTESIAN_POINT ( 'NONE',  ( -9.000000000000001776, 80.99999999999994316, 0.000000000000000000 ) ) ;
#67759=LINE ( 'NONE', #53731, #80726 ) ;
#67766=CARTESIAN_POINT ( 'NONE',  ( 11.10657215102223638, -52.67603735982828539, -4.000000000003583800 ) ) ;
#67779=DIRECTION ( 'NONE',  ( -0.000000000000000000, -0.000000000000000000, -1.000000000000000000 ) ) ;
#67792=VECTOR ( 'NONE', #54564, 1000.000000000000000 ) ;
#67795=( NAMED_UNIT ( * ) SI_UNIT ( $, .STERADIAN. ) SOLID_ANGLE_UNIT ( ) );
#67804=( LENGTH_UNIT ( ) NAMED_UNIT ( * ) SI_UNIT ( .MILLI., .METRE. ) );
#67807=ADVANCED_FACE ( 'NONE', ( #27054 ), #25130, .T. ) ;
#67816=( NAMED_UNIT ( * ) PLANE_ANGLE_UNIT ( ) SI_UNIT ( $, .RADIAN. ) );
#67823=STYLED_ITEM ( 'NONE', ( #1668 ), #52391 ) ;
#67834=CARTESIAN_POINT ( 'NONE',  ( 6.034057809536170325, -36.05796335879009007, -3.750000000000000444 ) ) ;
#67841=( LENGTH_UNIT ( ) NAMED_UNIT ( * ) SI_UNIT ( .MILLI., .METRE. ) );
#67849=CARTESIAN_POINT ( 'NONE',  ( 4.471066085527736433, -3.611416924289630348, -2.500000000000000000 ) ) ;
#67863=DIRECTION ( 'NONE',  ( 0.6246950475544238435, 0.7808688094430307203, 0.000000000000000000 ) ) ;
#67868=EDGE_CURVE ( 'NONE', #29547, #84748, #20247, .T. ) ;
#67869=DIRECTION ( 'NONE',  ( -0.000000000000000000, -0.000000000000000000, -1.000000000000000000 ) ) ;
#67870=VERTEX_POINT ( 'NONE', #75025 ) ;
#67903=CARTESIAN_POINT ( 'NONE',  ( 9.050000000000002487, 99.99999999999998579, 8.000000000000000000 ) ) ;
#67915=PRESENTATION_STYLE_ASSIGNMENT (( #91389 ) ) ;
#67920=CARTESIAN_POINT ( 'NONE',  ( 6.829574850505125028, -88.00372650098209704, 3.750000000000000000 ) ) ;
#67921=FACE_OUTER_BOUND ( 'NONE', #49194, .T. ) ;
#67931=ORIENTED_EDGE ( 'NONE', *, *, #46064, .T. ) ;
#67954=CARTESIAN_POINT ( 'NONE',  ( -6.867320125558078914, -58.36821204062274404, 2.750000000000000000 ) ) ;
#67987=CIRCLE ( 'NONE', #90297, 2.999999999999997780 ) ;
#68018=SURFACE_STYLE_FILL_AREA ( #41590 ) ;
#68035=CARTESIAN_POINT ( 'NONE',  ( -7.116171662430651246, -80.69120418497929847, -3.999999999998387956 ) ) ;
#68041=DIRECTION ( 'NONE',  ( -0.08715574274765093554, -0.9961946980917463224, 0.000000000000000000 ) ) ;
#68052=ORIENTED_EDGE ( 'NONE', *, *, #2682, .T. ) ;
#68053=CARTESIAN_POINT ( 'NONE',  ( 3.969999999999999751, 10.25000000000000000, -3.750000000000000000 ) ) ;
#68072=EDGE_LOOP ( 'NONE', ( #87631, #77183, #89655, #64824 ) ) ;
#68077=LINE ( 'NONE', #67083, #63408 ) ;
#68084=ADVANCED_FACE ( 'NONE', ( #5062 ), #7639, .T. ) ;
#68087=VERTEX_POINT ( 'NONE', #45014 ) ;
#68088=DIRECTION ( 'NONE',  ( 0.000000000000000000, 0.000000000000000000, 1.000000000000000000 ) ) ;
#68093=ORIENTED_EDGE ( 'NONE', *, *, #87137, .T. ) ;
#68125=MECHANICAL_DESIGN_GEOMETRIC_PRESENTATION_REPRESENTATION('',(#42561),#44111);
#68131=TOROIDAL_SURFACE ( 'NONE', #2698, 2.900000000000001243, 0.1000000000000000056 ) ;
#68134=LINE ( 'NONE', #73770, #97430 ) ;
#68136=ORIENTED_EDGE ( 'NONE', *, *, #95309, .F. ) ;
#68150=LINE ( 'NONE', #60131, #16416 ) ;
#68162=CARTESIAN_POINT ( 'NONE',  ( -11.58061176254664915, -84.07454167686761082, 4.000000000000000000 ) ) ;
#68168=( NAMED_UNIT ( * ) PLANE_ANGLE_UNIT ( ) SI_UNIT ( $, .RADIAN. ) );
#68172=EDGE_LOOP ( 'NONE', ( #45557, #66754, #96386, #24254 ) ) ;
#68174=ORIENTED_EDGE ( 'NONE', *, *, #82620, .T. ) ;
#68175=CYLINDRICAL_SURFACE ( 'NONE', #15784, 0.2500000000000002220 ) ;
#68187=EDGE_CURVE ( 'NONE', #31750, #79829, #20393, .T. ) ;
#68196=FACE_OUTER_BOUND ( 'NONE', #26525, .T. ) ;
#68199=ADVANCED_FACE ( 'NONE', ( #76996 ), #54970, .T. ) ;
#68204=EDGE_CURVE ( 'NONE', #34917, #11450, #96998, .T. ) ;
#68205=TOROIDAL_SURFACE ( 'NONE', #56974, 1.750000000000000888, 0.2500000000000000000 ) ;
#68206=CARTESIAN_POINT ( 'NONE',  ( -4.249999999999994671, 43.00000000000000711, 6.250000000000000000 ) ) ;
#68208=EDGE_CURVE ( 'NONE', #90212, #3379, #13981, .T. ) ;
#68209=DIRECTION ( 'NONE',  ( 0.000000000000000000, 0.000000000000000000, 1.000000000000000000 ) ) ;
#68211=DIRECTION ( 'NONE',  ( 0.000000000000000000, 0.000000000000000000, 1.000000000000000000 ) ) ;
#68212=CARTESIAN_POINT ( 'NONE',  ( -18.89999999999999503, 98.99999999999998579, -7.750000000000000000 ) ) ;
#68221=DIRECTION ( 'NONE',  ( 1.000000000000000000, 0.000000000000000000, 0.000000000000000000 ) ) ;
#68228=AXIS2_PLACEMENT_3D ( 'NONE', #34053, #25606, #49551 ) ;
#68234=CARTESIAN_POINT ( 'NONE',  ( 9.779999999999990479, 20.99999999999999645, 0.000000000000000000 ) ) ;
#68258=AXIS2_PLACEMENT_3D ( 'NONE', #77833, #9345, #75877 ) ;
#68262=ORIENTED_EDGE ( 'NONE', *, *, #78485, .F. ) ;
#68264=CARTESIAN_POINT ( 'NONE',  ( 10.93739314626210479, -97.13232482346681707, -3.750000000000000000 ) ) ;
#68293=SURFACE_STYLE_FILL_AREA ( #14306 ) ;
#68294=ORIENTED_EDGE ( 'NONE', *, *, #59826, .F. ) ;
#68302=CARTESIAN_POINT ( 'NONE',  ( -45.24390243902436737, 36.19512195121945553, -8.000000000000000000 ) ) ;
#68307=ORIENTED_EDGE ( 'NONE', *, *, #37815, .F. ) ;
#68317=CARTESIAN_POINT ( 'NONE',  ( -8.000343251535921851, 84.06932101904432386, 3.750000000000000000 ) ) ;
#68342=CARTESIAN_POINT ( 'NONE',  ( 6.655516370393623760, -69.44235516214573067, -2.500000000000000000 ) ) ;
#68354=DIRECTION ( 'NONE',  ( -0.000000000000000000, -0.000000000000000000, -1.000000000000000000 ) ) ;
#68359=( NAMED_UNIT ( * ) SI_UNIT ( $, .STERADIAN. ) SOLID_ANGLE_UNIT ( ) );
#68364=VECTOR ( 'NONE', #17745, 1000.000000000000000 ) ;
#68365=CARTESIAN_POINT ( 'NONE',  ( -10.91025143197891545, -52.91559880499231383, -3.999999999999998224 ) ) ;
#68371=DIRECTION ( 'NONE',  ( 1.000000000000000000, 0.000000000000000000, -0.000000000000000000 ) ) ;
#68378=LINE ( 'NONE', #22882, #59836 ) ;
#68383=LINE ( 'NONE', #68875, #78269 ) ;
#68419=CARTESIAN_POINT ( 'NONE',  ( -7.322384435959399696, -84.40865712959146094, -4.000000000000000000 ) ) ;
#68421=CARTESIAN_POINT ( 'NONE',  ( -8.000000000000000000, 75.73428692542562146, -2.900000000000000799 ) ) ;
#68426=STYLED_ITEM ( 'NONE', ( #91787 ), #14192 ) ;
#68437=EDGE_CURVE ( 'NONE', #44632, #26502, #69017, .T. ) ;
#68443=ADVANCED_FACE ( 'NONE', ( #15537 ), #548, .F. ) ;
#68458=CARTESIAN_POINT ( 'NONE',  ( 17.75000000000000000, 84.07179676972448590, 12.00000000000000000 ) ) ;
#68502=ORIENTED_EDGE ( 'NONE', *, *, #93027, .F. ) ;
#68511=DIRECTION ( 'NONE',  ( -0.9995586998285053149, -0.02970531260815256758, 0.000000000000000000 ) ) ;
#68537=CARTESIAN_POINT ( 'NONE',  ( -8.051738205446245189, 84.95449735710290895, -3.788866803286884632 ) ) ;
#68542=SURFACE_STYLE_FILL_AREA ( #38538 ) ;
#68564=ORIENTED_EDGE ( 'NONE', *, *, #24297, .T. ) ;
#68567=AXIS2_PLACEMENT_3D ( 'NONE', #84284, #44776, #91769 ) ;
#68571=DIRECTION ( 'NONE',  ( 1.000000000000000000, -0.000000000000000000, -0.000000000000000000 ) ) ;
#68572=CARTESIAN_POINT ( 'NONE',  ( 10.85666693323940102, -52.68303261961045081, 4.000000000000000000 ) ) ;
#68580=CARTESIAN_POINT ( 'NONE',  ( -7.750000000000000000, 79.82179676972448590, -6.250000000000000000 ) ) ;
#68592=EDGE_CURVE ( 'NONE', #30756, #52027, #57070, .T. ) ;
#68596=DIRECTION ( 'NONE',  ( 1.000000000000000000, 0.000000000000000000, 0.000000000000000000 ) ) ;
#68605=CARTESIAN_POINT ( 'NONE',  ( -6.445967608602039434, -48.01283281809150338, -3.750000000000000000 ) ) ;
#68635=( NAMED_UNIT ( * ) PLANE_ANGLE_UNIT ( ) SI_UNIT ( $, .RADIAN. ) );
#68637=EDGE_CURVE ( 'NONE', #8141, #39290, #23563, .T. ) ;
#68640=ORIENTED_EDGE ( 'NONE', *, *, #51720, .T. ) ;
#68645=CARTESIAN_POINT ( 'NONE',  ( -11.35564645740952372, -81.99443000160049166, 4.000000000000000000 ) ) ;
#68657=DIRECTION ( 'NONE',  ( 0.000000000000000000, -4.510281037539694659E-14, 1.000000000000000000 ) ) ;
#68669=DIRECTION ( 'NONE',  ( -0.000000000000000000, -0.000000000000000000, -1.000000000000000000 ) ) ;
#68676=VERTEX_POINT ( 'NONE', #27799 ) ;
#68682=CARTESIAN_POINT ( 'NONE',  ( -6.871316085749032965, -73.24163895400424451, 2.499999999999998224 ) ) ;
#68711=VERTEX_POINT ( 'NONE', #72797 ) ;
#68712=DIRECTION ( 'NONE',  ( -0.5905099943842175847, -0.8070303256584298035, 0.000000000000000000 ) ) ;
#68731=DIRECTION ( 'NONE',  ( -0.000000000000000000, -0.000000000000000000, -1.000000000000000000 ) ) ;
#68732=LINE ( 'NONE', #77201, #62803 ) ;
#68742=CYLINDRICAL_SURFACE ( 'NONE', #79058, 1.249999999999987121 ) ;
#68747=ORIENTED_EDGE ( 'NONE', *, *, #97379, .F. ) ;
#68749=CARTESIAN_POINT ( 'NONE',  ( 11.13643110663977431, -94.02619357115823107, -4.000000000000000000 ) ) ;
#68765=COLOUR_RGB ( '', 0.66274510, 0.83137255, 0.94901961) ;
#68767=CARTESIAN_POINT ( 'NONE',  ( -3.750000000000000000, 10.25000000000000000, 2.500000000000000000 ) ) ;
#68773=EDGE_CURVE ( 'NONE', #3379, #31285, #94112, .T. ) ;
#68781=EDGE_LOOP ( 'NONE', ( #48729, #93919, #80927, #74145 ) ) ;
#68790=PRESENTATION_STYLE_ASSIGNMENT (( #37805 ) ) ;
#68798=EDGE_CURVE ( 'NONE', #65197, #72511, #44773, .T. ) ;
#68800=ORIENTED_EDGE ( 'NONE', *, *, #72416, .T. ) ;
#68803=( NAMED_UNIT ( * ) SI_UNIT ( $, .STERADIAN. ) SOLID_ANGLE_UNIT ( ) );
#68804=SURFACE_STYLE_USAGE ( .BOTH. , #37819 ) ;
#68806=AXIS2_PLACEMENT_3D ( 'NONE', #74169, #89189, #28192 ) ;
#68811=CARTESIAN_POINT ( 'NONE',  ( -8.924603092375777535, 75.06466731010172566, -2.900000000000000799 ) ) ;
#68821=SURFACE_STYLE_USAGE ( .BOTH. , #29318 ) ;
#68825=AXIS2_PLACEMENT_3D ( 'NONE', #81864, #79547, #32556 ) ;
#68830=ADVANCED_FACE ( 'NONE', ( #22789 ), #37303, .T. ) ;
#68834=CARTESIAN_POINT ( 'NONE',  ( 4.441081520790487680, -2.684960557614425092, -2.750000000000000444 ) ) ;
#68838=CARTESIAN_POINT ( 'NONE',  ( 4.920090861810839655, -13.81657824362204678, 2.750000000000000444 ) ) ;
#68851=CARTESIAN_POINT ( 'NONE',  ( -8.000000000000000000, -0.01655697267263257777, -3.750000000000000000 ) ) ;
#68855=LINE ( 'NONE', #74355, #11357 ) ;
#68860=CARTESIAN_POINT ( 'NONE',  ( -7.750000000000000000, 40.99999999999999289, 6.250000000000000000 ) ) ;
#68875=CARTESIAN_POINT ( 'NONE',  ( -9.024359497401759356, 75.07164295747612925, 2.900000000000000355 ) ) ;
#68884=ADVANCED_FACE ( 'NONE', ( #75771 ), #81052, .T. ) ;
#68885=EDGE_CURVE ( 'NONE', #46257, #39257, #2792, .T. ) ;
#68901=ORIENTED_EDGE ( 'NONE', *, *, #70442, .F. ) ;
#68934=COLOUR_RGB ( '', 0.40784314, 0.44705882, 0.49803922) ;
#68941=CARTESIAN_POINT ( 'NONE',  ( 11.24699797944280100, 54.09857164847241506, 0.000000000000000000 ) ) ;
#68944=CARTESIAN_POINT ( 'NONE',  ( 4.630000000000003446, 1.019547802438462547, -4.000000000000000000 ) ) ;
#68949=ORIENTED_EDGE ( 'NONE', *, *, #54646, .T. ) ;
#68952=PLANE ( 'NONE',  #72736 ) ;
#68959=CARTESIAN_POINT ( 'NONE',  ( 4.380000000000000782, -0.01592157648205478476, -3.750000000000000888 ) ) ;
#68973=AXIS2_PLACEMENT_3D ( 'NONE', #51776, #26800, #58266 ) ;
#68978=CARTESIAN_POINT ( 'NONE',  ( -3.750000000000000000, 37.25000000000000000, -3.750000000000000000 ) ) ;
#68986=DIRECTION ( 'NONE',  ( 0.000000000000000000, -1.000000000000000000, 0.000000000000000000 ) ) ;
#69004=CARTESIAN_POINT ( 'NONE',  ( -8.024359497401761132, 75.03672218798435267, 3.000000000000000000 ) ) ;
#69006=( GEOMETRIC_REPRESENTATION_CONTEXT ( 3 ) GLOBAL_UNCERTAINTY_ASSIGNED_CONTEXT ( ( #83385 ) ) GLOBAL_UNIT_ASSIGNED_CONTEXT ( ( #5455, #21934, #81428 ) ) REPRESENTATION_CONTEXT ( 'NONE', 'WORKASPACE' ) );
#69009=CYLINDRICAL_SURFACE ( 'NONE', #54850, 0.2500000000000002220 ) ;
#69017=LINE ( 'NONE', #62471, #79422 ) ;
#69022=CARTESIAN_POINT ( 'NONE',  ( -7.080143328636912869, -69.54337233422656084, -3.999999999999999556 ) ) ;
#69033=CARTESIAN_POINT ( 'NONE',  ( 0.4400000000000020006, 1.019547802438468986, -4.000000000000000000 ) ) ;
#69047=VECTOR ( 'NONE', #6946, 1000.000000000000000 ) ;
#69049=VERTEX_POINT ( 'NONE', #69759 ) ;
#69066=ORIENTED_EDGE ( 'NONE', *, *, #68208, .T. ) ;
#69067=ORIENTED_EDGE ( 'NONE', *, *, #75307, .T. ) ;
#69071=CIRCLE ( 'NONE', #8405, 0.2500000000000002220 ) ;
#69083=EDGE_CURVE ( 'NONE', #92042, #20156, #93725, .T. ) ;
#69096=CARTESIAN_POINT ( 'NONE',  ( -6.560019409699617832, -50.64698701990471363, -2.750000000000000444 ) ) ;
#69098=CYLINDRICAL_SURFACE ( 'NONE', #7115, 0.1000000000000001166 ) ;
#69099=AXIS2_PLACEMENT_3D ( 'NONE', #49373, #8917, #77904 ) ;
#69104=( LENGTH_UNIT ( ) NAMED_UNIT ( * ) SI_UNIT ( .MILLI., .METRE. ) );
#69106=CARTESIAN_POINT ( 'NONE',  ( 17.75000000000000711, 43.00000000000000000, 6.500000000000000888 ) ) ;
#69107=SURFACE_STYLE_FILL_AREA ( #15133 ) ;
#69112=EDGE_CURVE ( 'NONE', #59804, #45794, #7703, .T. ) ;
#69114=UNCERTAINTY_MEASURE_WITH_UNIT (LENGTH_MEASURE( 1.000000000000000082E-05 ), #57296, 'distance_accuracy_value', 'NONE');
#69133=PRESENTATION_STYLE_ASSIGNMENT (( #92605 ) ) ;
#69141=CARTESIAN_POINT ( 'NONE',  ( -11.58061176244991053, -84.07454167686546498, 3.750000000000000000 ) ) ;
#69146=COLOUR_RGB ( '', 0.66274510, 0.83137255, 0.94901961) ;
#69148=VECTOR ( 'NONE', #64383, 1000.000000000000000 ) ;
#69157=ORIENTED_EDGE ( 'NONE', *, *, #30598, .T. ) ;
#69164=( LENGTH_UNIT ( ) NAMED_UNIT ( * ) SI_UNIT ( .MILLI., .METRE. ) );
#69178=CARTESIAN_POINT ( 'NONE',  ( -6.732636091893173358, -88.11213685669363826, 2.500000000000000000 ) ) ;
#69181=CIRCLE ( 'NONE', #21284, 0.2499999999999997224 ) ;
#69183=AXIS2_PLACEMENT_3D ( 'NONE', #16430, #8915, #39431 ) ;
#69189=CARTESIAN_POINT ( 'NONE',  ( 12.24319267753454099, 54.01141590572475337, -2.900000000000000799 ) ) ;
#69192=CARTESIAN_POINT ( 'NONE',  ( -3.500000000000000444, -0.04521315095527938394, 2.750000000000000000 ) ) ;
#69204=ADVANCED_FACE ( 'NONE', ( #55743 ), #51411, .T. ) ;
#69208=VERTEX_POINT ( 'NONE', #96704 ) ;
#69213=DIRECTION ( 'NONE',  ( 1.000000000000000000, -0.000000000000000000, -0.000000000000000000 ) ) ;
#69215=FILL_AREA_STYLE_COLOUR ( '', #11818 ) ;
#69220=AXIS2_PLACEMENT_3D ( 'NONE', #8798, #63263, #17302 ) ;
#69224=CARTESIAN_POINT ( 'NONE',  ( 6.579634127946653699, -87.99828267815712479, 2.750000000000002665 ) ) ;
#69231=ORIENTED_EDGE ( 'NONE', *, *, #12330, .F. ) ;
#69237=( LENGTH_UNIT ( ) NAMED_UNIT ( * ) SI_UNIT ( .MILLI., .METRE. ) );
#69238=DIRECTION ( 'NONE',  ( 0.8070303256584298035, -0.5905099943842175847, 0.000000000000000000 ) ) ;
#69246=( NAMED_UNIT ( * ) SI_UNIT ( $, .STERADIAN. ) SOLID_ANGLE_UNIT ( ) );
#69258=UNCERTAINTY_MEASURE_WITH_UNIT (LENGTH_MEASURE( 1.000000000000000082E-05 ), #21545, 'distance_accuracy_value', 'NONE');
#69262=CARTESIAN_POINT ( 'NONE',  ( 14.99999999999997868, 80.07179676972448590, 6.500000000000000888 ) ) ;
#69283=FILL_AREA_STYLE ('',( #80820 ) ) ;
#69284=ORIENTED_EDGE ( 'NONE', *, *, #66853, .F. ) ;
#69290=EDGE_CURVE ( 'NONE', #23479, #93500, #53937, .T. ) ;
#69301=( LENGTH_UNIT ( ) NAMED_UNIT ( * ) SI_UNIT ( .MILLI., .METRE. ) );
#69304=CARTESIAN_POINT ( 'NONE',  ( 4.600000000000003197, 98.49999999999998579, 8.000000000000000000 ) ) ;
#69311=CARTESIAN_POINT ( 'NONE',  ( -6.030799524552431734, -39.80423606248630364, -2.750000000000000000 ) ) ;
#69322=CARTESIAN_POINT ( 'NONE',  ( 4.221206346829659672, -3.619822760609359591, -2.500000000000000000 ) ) ;
#69324=ADVANCED_FACE ( 'NONE', ( #72682 ), #65181, .F. ) ;
#69326=CARTESIAN_POINT ( 'NONE',  ( 4.380000000000002558, 1.019547802438462547, 2.750000000000000000 ) ) ;
#69336=CARTESIAN_POINT ( 'NONE',  ( -8.647966315087309397, -15.58183027064585779, -4.000000000000000000 ) ) ;
#69352=EDGE_CURVE ( 'NONE', #74689, #55012, #35686, .T. ) ;
#69355=CARTESIAN_POINT ( 'NONE',  ( -3.750000000000000000, 10.00000000000000000, 3.750000000000000000 ) ) ;
#69367=FILL_AREA_STYLE_COLOUR ( '', #30782 ) ;
#69374=LINE ( 'NONE', #896, #64580 ) ;
#69385=CIRCLE ( 'NONE', #96734, 8.000000000000007105 ) ;
#69391=CARTESIAN_POINT ( 'NONE',  ( 6.757940885659567520, -58.32678904743372073, 3.999999999999999556 ) ) ;
#69392=SURFACE_SIDE_STYLE ('',( #54866 ) ) ;
#69396=CARTESIAN_POINT ( 'NONE',  ( -5.580435433942703582, -28.67474180225207547, -3.999999999999998224 ) ) ;
#69410=CARTESIAN_POINT ( 'NONE',  ( 17.74999999999999645, 91.00000000000000000, -8.000000000000000000 ) ) ;
#69412=VECTOR ( 'NONE', #33406, 1000.000000000000000 ) ;
#69423=FILL_AREA_STYLE ('',( #31405 ) ) ;
#69426=DIRECTION ( 'NONE',  ( 1.000000000000000000, 0.000000000000000000, 0.000000000000000000 ) ) ;
#69434=VECTOR ( 'NONE', #97281, 1000.000000000000000 ) ;
#69440=LINE ( 'NONE', #8441, #29628 ) ;
#69446=CARTESIAN_POINT ( 'NONE',  ( 4.400664535130860422, -1.180071741297640253, -2.750000000000000000 ) ) ;
#69447=CARTESIAN_POINT ( 'NONE',  ( 4.471066085529306733, -3.611416924331345868, 2.500000000000000000 ) ) ;
#69449=ORIENTED_EDGE ( 'NONE', *, *, #64578, .F. ) ;
#69453=AXIS2_PLACEMENT_3D ( 'NONE', #59673, #195, #91660 ) ;
#69461=ORIENTED_EDGE ( 'NONE', *, *, #66209, .F. ) ;
#69463=LINE ( 'NONE', #31931, #66183 ) ;
#69464=DIRECTION ( 'NONE',  ( 0.000000000000000000, 0.000000000000000000, -1.000000000000000000 ) ) ;
#69465=DIRECTION ( 'NONE',  ( 0.8070303256584298035, -0.5905099943842175847, 0.000000000000000000 ) ) ;
#69468=CARTESIAN_POINT ( 'NONE',  ( 17.82550711101916008, 78.51652315108729852, 4.000000000000000888 ) ) ;
#69470=ADVANCED_FACE ( 'NONE', ( #35178 ), #34688, .T. ) ;
#69471=CARTESIAN_POINT ( 'NONE',  ( 4.691428608706885051, -2.693193260553968127, -4.000000000000000000 ) ) ;
#69486=SPHERICAL_SURFACE ( 'NONE', #51285, 0.2500000000000000000 ) ;
#69494=DIRECTION ( 'NONE',  ( -0.5901017155107530776, -0.8073289077886820486, 0.000000000000000000 ) ) ;
#69497=EDGE_LOOP ( 'NONE', ( #92245, #2395, #78816, #65167 ) ) ;
#69519=CARTESIAN_POINT ( 'NONE',  ( -9.524127588832328684, 88.37770237764364367, -5.051303975189256334 ) ) ;
#69537=EDGE_CURVE ( 'NONE', #42048, #80996, #20466, .T. ) ;
#69545=ORIENTED_EDGE ( 'NONE', *, *, #71634, .T. ) ;
#69560=CARTESIAN_POINT ( 'NONE',  ( 6.880000000000009663, 40.99999999999999289, 6.250000000000000000 ) ) ;
#69585=FACE_OUTER_BOUND ( 'NONE', #51602, .T. ) ;
#69587=ADVANCED_FACE ( 'NONE', ( #44157 ), #58705, .T. ) ;
#69598=EDGE_CURVE ( 'NONE', #36801, #55896, #74666, .T. ) ;
#69603=AXIS2_PLACEMENT_3D ( 'NONE', #66790, #52766, #59772 ) ;
#69629=CARTESIAN_POINT ( 'NONE',  ( -7.909656209098489654, -4.175824794483175673, 4.000000000000000000 ) ) ;
#69638=EDGE_CURVE ( 'NONE', #19346, #55759, #65115, .T. ) ;
#69640=DIRECTION ( 'NONE',  ( 1.000000000000000000, 0.000000000000000000, 0.000000000000000000 ) ) ;
#69651=CARTESIAN_POINT ( 'NONE',  ( 5.129999999999995453, 43.00000000000000711, 6.500000000000000888 ) ) ;
#69653=VERTEX_POINT ( 'NONE', #58678 ) ;
#69662=CARTESIAN_POINT ( 'NONE',  ( -3.521020805652878671, -6.414291667507525219, 2.500000000000000444 ) ) ;
#69667=CARTESIAN_POINT ( 'NONE',  ( -3.750000000000000000, 37.00000000000000000, -3.750000000000000000 ) ) ;
#69668=ADVANCED_FACE ( 'NONE', ( #15171 ), #4491, .T. ) ;
#69670=CARTESIAN_POINT ( 'NONE',  ( -3.271890209819976025, -0.8418601081563239497, 2.500000000000000888 ) ) ;
#69671=ORIENTED_EDGE ( 'NONE', *, *, #76299, .F. ) ;
#69672=CARTESIAN_POINT ( 'NONE',  ( 8.955817848464572961, -3.107653060326661887, 4.000000000000000000 ) ) ;
#69676=CARTESIAN_POINT ( 'NONE',  ( 9.779999999999988702, 27.00436609429084811, 3.000000000000000000 ) ) ;
#69677=CARTESIAN_POINT ( 'NONE',  ( 1.350000000000004086, 98.49999999999998579, -8.525133428036873795 ) ) ;
#69688=CARTESIAN_POINT ( 'NONE',  ( 6.934003561272774618, -73.15726776830514666, -2.750000000000000444 ) ) ;
#69693=AXIS2_PLACEMENT_3D ( 'NONE', #96611, #80609, #96112 ) ;
#69694=ORIENTED_EDGE ( 'NONE', *, *, #33950, .F. ) ;
#69700=DIRECTION ( 'NONE',  ( -0.000000000000000000, 0.000000000000000000, 1.000000000000000000 ) ) ;
#69732=CARTESIAN_POINT ( 'NONE',  ( 8.862914611804004750, -7.247476534019402727, -4.000000000000000000 ) ) ;
#69740=FILL_AREA_STYLE ('',( #38753 ) ) ;
#69742=AXIS2_PLACEMENT_3D ( 'NONE', #42197, #5673, #66148 ) ;
#69745=AXIS2_PLACEMENT_3D ( 'NONE', #27092, #19605, #12591 ) ;
#69746=ORIENTED_EDGE ( 'NONE', *, *, #48337, .T. ) ;
#69749=CARTESIAN_POINT ( 'NONE',  ( -8.000000000000000000, 1.019547802438466100, 3.750000000000000000 ) ) ;
#69759=CARTESIAN_POINT ( 'NONE',  ( -7.750000000000000000, 80.07179676972448590, 4.250000000000000000 ) ) ;
#69763=VERTEX_POINT ( 'NONE', #55105 ) ;
#69772=SURFACE_SIDE_STYLE ('',( #84771 ) ) ;
#69773=VERTEX_POINT ( 'NONE', #47113 ) ;
#69783=FILL_AREA_STYLE ('',( #54755 ) ) ;
#69786=( NAMED_UNIT ( * ) PLANE_ANGLE_UNIT ( ) SI_UNIT ( $, .RADIAN. ) );
#69790=CIRCLE ( 'NONE', #66573, 0.2500000000000002220 ) ;
#69804=CARTESIAN_POINT ( 'NONE',  ( 4.573266373291863474, -6.401889604903887587, -3.750000000000001776 ) ) ;
#69807=( NAMED_UNIT ( * ) PLANE_ANGLE_UNIT ( ) SI_UNIT ( $, .RADIAN. ) );
#69817=CARTESIAN_POINT ( 'NONE',  ( -10.89045396206093663, 89.68015320059714668, 6.284968870998880242 ) ) ;
#69824=CYLINDRICAL_SURFACE ( 'NONE', #24787, 0.2500000000000002220 ) ;
#69827=SURFACE_STYLE_FILL_AREA ( #18295 ) ;
#69831=DIRECTION ( 'NONE',  ( 0.000000000000000000, 1.000000000000000000, -0.000000000000000000 ) ) ;
#69838=ORIENTED_EDGE ( 'NONE', *, *, #20955, .F. ) ;
#69841=PRESENTATION_STYLE_ASSIGNMENT (( #7378 ) ) ;
#69849=VERTEX_POINT ( 'NONE', #77614 ) ;
#69851=FACE_OUTER_BOUND ( 'NONE', #72027, .T. ) ;
#69858=DIRECTION ( 'NONE',  ( 1.000000000000000000, 0.000000000000000000, 0.000000000000000000 ) ) ;
#69889=CARTESIAN_POINT ( 'NONE',  ( 6.284516029235898138, -36.06297093898795936, 4.000000000000000000 ) ) ;
#69891=PRESENTATION_STYLE_ASSIGNMENT (( #16395 ) ) ;
#69905=DIRECTION ( 'NONE',  ( 0.9975640502598243087, -0.06975647374412535795, 0.000000000000000000 ) ) ;
#69909=EDGE_CURVE ( 'NONE', #76829, #16659, #54125, .T. ) ;
#69920=CARTESIAN_POINT ( 'NONE',  ( -10.86761736821483026, -97.98327470060252153, 3.750000000000000888 ) ) ;
#69928=PRESENTATION_STYLE_ASSIGNMENT (( #71409 ) ) ;
#69944=CARTESIAN_POINT ( 'NONE',  ( 5.113979357112576452, -17.50950876262128730, 2.750000000000000000 ) ) ;
#69956=EDGE_LOOP ( 'NONE', ( #95688, #28602, #10154, #44860, #79415, #73437, #93849, #2067, #27700, #8288, #82647, #39050, #56460, #59977, #14185, #7310, #30173, #81101, #86220, #23521 ) ) ;
#69959=( NAMED_UNIT ( * ) PLANE_ANGLE_UNIT ( ) SI_UNIT ( $, .RADIAN. ) );
#69960=CARTESIAN_POINT ( 'NONE',  ( -3.750000000000000000, 36.75000000000000000, -3.750000000000000000 ) ) ;
#69963=SPHERICAL_SURFACE ( 'NONE', #75238, 0.2500000000000000000 ) ;
#69966=CARTESIAN_POINT ( 'NONE',  ( -7.750355510519348456, 84.07179676972448590, -3.750000000000000000 ) ) ;
#69967=CARTESIAN_POINT ( 'NONE',  ( -8.099999999999999645, 75.73428692542562146, -3.000000000000000000 ) ) ;
#69987=EDGE_LOOP ( 'NONE', ( #39118, #61110, #94045, #46195 ) ) ;
#69989=DIRECTION ( 'NONE',  ( -0.000000000000000000, -0.000000000000000000, 1.000000000000000000 ) ) ;
#69994=VECTOR ( 'NONE', #98735, 1000.000000000000000 ) ;
#69997=CARTESIAN_POINT ( 'NONE',  ( 5.129999999999990123, 76.07179676972444327, 6.250000000000000000 ) ) ;
#70001=VECTOR ( 'NONE', #88299, 1000.000000000000000 ) ;
#70016=ADVANCED_FACE ( 'NONE', ( #92620 ), #73191, .F. ) ;
#70018=DIRECTION ( 'NONE',  ( -0.000000000000000000, 0.000000000000000000, 1.000000000000000000 ) ) ;
#70024=EDGE_CURVE ( 'NONE', #1559, #23534, #54006, .T. ) ;
#70038=ORIENTED_EDGE ( 'NONE', *, *, #79708, .F. ) ;
#70047=ORIENTED_EDGE ( 'NONE', *, *, #68885, .T. ) ;
#70061=CARTESIAN_POINT ( 'NONE',  ( 5.800000000000003375, 99.99999999999998579, 8.000000000000000000 ) ) ;
#70062=EDGE_LOOP ( 'NONE', ( #53648, #28187, #75575, #96830 ) ) ;
#70067=MECHANICAL_DESIGN_GEOMETRIC_PRESENTATION_REPRESENTATION('',(#71635),#1428);
#70068=( NAMED_UNIT ( * ) SI_UNIT ( $, .STERADIAN. ) SOLID_ANGLE_UNIT ( ) );
#70087=PLANE ( 'NONE',  #2151 ) ;
#70090=AXIS2_PLACEMENT_3D ( 'NONE', #87, #13571, #30534 ) ;
#70112=CARTESIAN_POINT ( 'NONE',  ( -9.024359497401759356, 75.07164295747612925, 2.900000000000000355 ) ) ;
#70115=UNCERTAINTY_MEASURE_WITH_UNIT (LENGTH_MEASURE( 1.000000000000000082E-05 ), #15972, 'distance_accuracy_value', 'NONE');
#70148=( NAMED_UNIT ( * ) PLANE_ANGLE_UNIT ( ) SI_UNIT ( $, .RADIAN. ) );
#70149=COLOUR_RGB ( '', 0.40784314, 0.44705882, 0.49803922) ;
#70170=CARTESIAN_POINT ( 'NONE',  ( -3.521809513897764532, -0.8352226969157688918, 2.749999999999798828 ) ) ;
#70173=SURFACE_STYLE_FILL_AREA ( #47661 ) ;
#70174=DIRECTION ( 'NONE',  ( 0.000000000000000000, 0.000000000000000000, -1.000000000000000000 ) ) ;
#70187=CARTESIAN_POINT ( 'NONE',  ( 6.574847571008442415, -50.89175608690136698, -2.750000000000000888 ) ) ;
#70194=SURFACE_STYLE_FILL_AREA ( #78177 ) ;
#70197=DIRECTION ( 'NONE',  ( -1.000000000000000000, 0.000000000000000000, -0.000000000000000000 ) ) ;
#70205=DIRECTION ( 'NONE',  ( -0.000000000000000000, 0.000000000000000000, 1.000000000000000000 ) ) ;
#70214=ORIENTED_EDGE ( 'NONE', *, *, #36318, .T. ) ;
#70226=CARTESIAN_POINT ( 'NONE',  ( 8.991946320728366970, -4.139779132962734032, -3.750000000000000000 ) ) ;
#70227=CIRCLE ( 'NONE', #74997, 0.2500000000000002220 ) ;
#70234=DIRECTION ( 'NONE',  ( 1.000000000000000000, 0.000000000000000000, 0.000000000000000000 ) ) ;
#70236=STYLED_ITEM ( 'NONE', ( #74306 ), #22494 ) ;
#70237=AXIS2_PLACEMENT_3D ( 'NONE', #19952, #25990, #27451 ) ;
#70239=UNCERTAINTY_MEASURE_WITH_UNIT (LENGTH_MEASURE( 1.000000000000000082E-05 ), #33948, 'distance_accuracy_value', 'NONE');
#70244=CARTESIAN_POINT ( 'NONE',  ( 8.880000000000020322, 80.32179676972448590, -4.000000000000000000 ) ) ;
#70253=EDGE_CURVE ( 'NONE', #85496, #49230, #42871, .T. ) ;
#70255=CARTESIAN_POINT ( 'NONE',  ( -3.750000000000000000, 36.75000000000000000, 2.750000000000000000 ) ) ;
#70259=CARTESIAN_POINT ( 'NONE',  ( -4.537879770860196338, -17.56524742836564101, 3.750000000002418954 ) ) ;
#70260=ORIENTED_EDGE ( 'NONE', *, *, #97473, .T. ) ;
#70269=VERTEX_POINT ( 'NONE', #5076 ) ;
#70302=CARTESIAN_POINT ( 'NONE',  ( -7.121361048738320321, -73.24645952185287001, -2.750000000000000444 ) ) ;
#70313=CARTESIAN_POINT ( 'NONE',  ( -8.860528122731230027, 87.38741345285838236, 4.488970891313635470 ) ) ;
#70325=DIRECTION ( 'NONE',  ( -0.9975640502598243087, 0.06975647374412535795, -0.000000000000000000 ) ) ;
#70336=CARTESIAN_POINT ( 'NONE',  ( -9.538220187641574199, 88.39559135149089286, -5.063080553068876277 ) ) ;
#70343=VERTEX_POINT ( 'NONE', #66054 ) ;
#70351=DIRECTION ( 'NONE',  ( -0.000000000000000000, 0.000000000000000000, 1.000000000000000000 ) ) ;
#70359=UNCERTAINTY_MEASURE_WITH_UNIT (LENGTH_MEASURE( 1.000000000000000082E-05 ), #48522, 'distance_accuracy_value', 'NONE');
#70360=AXIS2_PLACEMENT_3D ( 'NONE', #31226, #54227, #39739 ) ;
#70371=AXIS2_PLACEMENT_3D ( 'NONE', #44868, #89392, #6380 ) ;
#70374=TOROIDAL_SURFACE ( 'NONE', #35215, 2.900000000000001243, 0.1000000000000000056 ) ;
#70379=VERTEX_POINT ( 'NONE', #52054 ) ;
#70382=EDGE_LOOP ( 'NONE', ( #12619, #54740, #45688, #10852, #83544, #59784, #58952, #5080, #45622, #30162, #14601, #23106, #96181, #81190 ) ) ;
#70389=CARTESIAN_POINT ( 'NONE',  ( -7.117803565204842364, -58.38168516195393920, -4.000000000000000888 ) ) ;
#70401=CIRCLE ( 'NONE', #68825, 0.2500000000000002220 ) ;
#70402=EDGE_CURVE ( 'NONE', #25656, #93854, #82767, .T. ) ;
#70403=TOROIDAL_SURFACE ( 'NONE', #76743, 4.250000000000001776, 0.2500000000000000000 ) ;
#70409=EDGE_LOOP ( 'NONE', ( #3349, #93652, #24117, #17573, #57958 ) ) ;
#70414=CARTESIAN_POINT ( 'NONE',  ( -10.79817015753363840, -44.62824817291426882, 3.750000000000000888 ) ) ;
#70415=SURFACE_SIDE_STYLE ('',( #9410 ) ) ;
#70417=DIRECTION ( 'NONE',  ( 0.000000000000000000, 0.000000000000000000, -1.000000000000000000 ) ) ;
#70426=CARTESIAN_POINT ( 'NONE',  ( -13.78592789153091225, 90.90750312509719322, 7.843642351634943388 ) ) ;
#70429=AXIS2_PLACEMENT_3D ( 'NONE', #23382, #70351, #69858 ) ;
#70442=EDGE_CURVE ( 'NONE', #2021, #40706, #90759, .T. ) ;
#70451=DIRECTION ( 'NONE',  ( -1.000000000000000000, -0.000000000000000000, -0.000000000000000000 ) ) ;
#70452=DIRECTION ( 'NONE',  ( 1.000000000000000000, 0.000000000000000000, 0.000000000000000000 ) ) ;
#70460=CARTESIAN_POINT ( 'NONE',  ( -8.099999999999999645, 80.99999999999994316, 3.000000000000000000 ) ) ;
#70467=ORIENTED_EDGE ( 'NONE', *, *, #58707, .T. ) ;
#70469=AXIS2_PLACEMENT_3D ( 'NONE', #20389, #96897, #57875 ) ;
#70484=PRESENTATION_STYLE_ASSIGNMENT (( #33436 ) ) ;
#70494=MECHANICAL_DESIGN_GEOMETRIC_PRESENTATION_REPRESENTATION('',(#95972),#83187);
#70497=FACE_OUTER_BOUND ( 'NONE', #5332, .T. ) ;
#70499=VERTEX_POINT ( 'NONE', #6547 ) ;
#70523=ADVANCED_FACE ( 'NONE', ( #67556 ), #1542, .T. ) ;
#70533=DIRECTION ( 'NONE',  ( 0.000000000000000000, 0.000000000000000000, 1.000000000000000000 ) ) ;
#70556=DIRECTION ( 'NONE',  ( -0.000000000000000000, -1.000000000000000000, -0.000000000000000000 ) ) ;
#70565=VERTEX_POINT ( 'NONE', #92502 ) ;
#70570=STYLED_ITEM ( 'NONE', ( #89427 ), #47084 ) ;
#70574=SURFACE_STYLE_FILL_AREA ( #16589 ) ;
#70579=DIRECTION ( 'NONE',  ( -0.000000000000000000, 1.000000000000000000, 0.000000000000000000 ) ) ;
#70580=AXIS2_PLACEMENT_3D ( 'NONE', #56159, #86652, #41165 ) ;
#70593=CYLINDRICAL_SURFACE ( 'NONE', #84639, 10.90000000000026326 ) ;
#70609=DIRECTION ( 'NONE',  ( -0.000000000000000000, 0.000000000000000000, 1.000000000000000000 ) ) ;
#70618=CARTESIAN_POINT ( 'NONE',  ( -16.94999999999999574, 99.99999999999998579, -8.525133428036873795 ) ) ;
#70637=DIRECTION ( 'NONE',  ( 1.000000000000000000, 1.927470528863119542E-16, -0.000000000000000000 ) ) ;
#70643=VECTOR ( 'NONE', #76307, 1000.000000000000000 ) ;
#70644=AXIS2_PLACEMENT_3D ( 'NONE', #33621, #19132, #80120 ) ;
#70646=ORIENTED_EDGE ( 'NONE', *, *, #80880, .T. ) ;
#70657=B_SPLINE_CURVE_WITH_KNOTS ( 'NONE', 3,
 ( #57563, #88061, #10602, #11093, #19573, #12563, #50070, #80574, #65550, #5072, #3118, #71606 ),
 .UNSPECIFIED., .F., .F.,
 ( 4, 2, 2, 2, 2, 4 ),
 ( 0.000000000000000000, 0.0003464182178352352313, 0.0005196273267528502991, 0.0006062318812116581582, 0.0006495341584410644188, 0.0006928364356704708963 ),
 .UNSPECIFIED. ) ;
#70658=COLOUR_RGB ( '', 0.08235294, 0.09019608, 0.10196078) ;
#70661=CARTESIAN_POINT ( 'NONE',  ( -3.638343494402940248, -8.270261767329087021, 2.500000000000001332 ) ) ;
#70662=VERTEX_POINT ( 'NONE', #31502 ) ;
#70663=DIRECTION ( 'NONE',  ( 0.000000000000000000, 0.000000000000000000, 1.000000000000000000 ) ) ;
#70674=VERTEX_POINT ( 'NONE', #92996 ) ;
#70680=CARTESIAN_POINT ( 'NONE',  ( 6.829574850505127692, -88.00372650098204019, -2.750000000000000444 ) ) ;
#70692=DIRECTION ( 'NONE',  ( 1.000000000000000000, 0.000000000000000000, 0.000000000000000000 ) ) ;
#70714=DIRECTION ( 'NONE',  ( 0.6246950475544237324, 0.7808688094430306093, 0.000000000000000000 ) ) ;
#70715=AXIS2_PLACEMENT_3D ( 'NONE', #36621, #15110, #29097 ) ;
#70737=EDGE_LOOP ( 'NONE', ( #77376, #94730, #5220, #50830 ) ) ;
#70738=LINE ( 'NONE', #55730, #27790 ) ;
#70744=PRESENTATION_STYLE_ASSIGNMENT (( #86721 ) ) ;
#70748=B_SPLINE_CURVE_WITH_KNOTS ( 'NONE', 3,
 ( #65648, #96171, #66140, #73640, #79683, #58141 ),
 .UNSPECIFIED., .F., .F.,
 ( 4, 2, 4 ),
 ( 0.000000000000000000, 0.0002092266038752941626, 0.0004184532077505883252 ),
 .UNSPECIFIED. ) ;
#70756=CARTESIAN_POINT ( 'NONE',  ( -7.116171662429844780, -80.69120418497929847, 3.999999999999194422 ) ) ;
#70765=CARTESIAN_POINT ( 'NONE',  ( -3.749999999999994671, 43.00000000000000711, -4.250000000000000000 ) ) ;
#70770=ORIENTED_EDGE ( 'NONE', *, *, #21840, .T. ) ;
#70778=CARTESIAN_POINT ( 'NONE',  ( -1.899999999999997247, 98.49999999999998579, -8.000000000000000000 ) ) ;
#70780=EDGE_CURVE ( 'NONE', #42155, #36998, #41259, .T. ) ;
#70789=VECTOR ( 'NONE', #37134, 1000.000000000000000 ) ;
#70796=CARTESIAN_POINT ( 'NONE',  ( -8.000000000000000000, 80.99999999999994316, -2.900000000000000799 ) ) ;
#70801=DIRECTION ( 'NONE',  ( -1.000000000000000000, 0.000000000000000000, 0.000000000000000000 ) ) ;
#70807=CARTESIAN_POINT ( 'NONE',  ( -8.051923691749143686, 84.95650211105896688, 3.789018682291705797 ) ) ;
#70810=ADVANCED_FACE ( 'NONE', ( #25019 ), #23547, .F. ) ;
#70812=DIRECTION ( 'NONE',  ( 0.000000000000000000, -0.000000000000000000, -1.000000000000000000 ) ) ;
#70821=CARTESIAN_POINT ( 'NONE',  ( 17.99999999999999645, 78.65116497101854520, -3.750000000000000888 ) ) ;
#70826=CIRCLE ( 'NONE', #30834, 0.1000000000000001166 ) ;
#70832=CARTESIAN_POINT ( 'NONE',  ( -3.750000000000000000, 37.00000000000000000, -2.750000000000000000 ) ) ;
#70833=FILL_AREA_STYLE ('',( #78808 ) ) ;
#70841=PRESENTATION_STYLE_ASSIGNMENT (( #9837 ) ) ;
#70856=MECHANICAL_DESIGN_GEOMETRIC_PRESENTATION_REPRESENTATION('',(#93165),#94962);
#70861=CARTESIAN_POINT ( 'NONE',  ( 9.879999999999988347, 26.99999999999999645, 3.000000000000000000 ) ) ;
#70869=STYLED_ITEM ( 'NONE', ( #62463 ), #93184 ) ;
#70878=VERTEX_POINT ( 'NONE', #17517 ) ;
#70929=DIRECTION ( 'NONE',  ( 0.9975640502598243087, -0.06975647374412535795, 0.000000000000000000 ) ) ;
#70938=CARTESIAN_POINT ( 'NONE',  ( 4.406185888756865232, -8.255243720450049949, 2.500000000000000000 ) ) ;
#70952=FILL_AREA_STYLE_COLOUR ( '', #14787 ) ;
#70957=SURFACE_STYLE_USAGE ( .BOTH. , #77947 ) ;
#70958=PRESENTATION_STYLE_ASSIGNMENT (( #40460 ) ) ;
#70959=CARTESIAN_POINT ( 'NONE',  ( -8.900000000000000355, 75.73428692542562146, 2.900000000000000355 ) ) ;
#70972=CARTESIAN_POINT ( 'NONE',  ( -6.581680125707232598, -88.31141629936868753, 2.500000000000000000 ) ) ;
#70981=ORIENTED_EDGE ( 'NONE', *, *, #14605, .F. ) ;
#70982=CARTESIAN_POINT ( 'NONE',  ( 17.75000000000000000, 84.07179676972448590, -12.00000000000000000 ) ) ;
#70992=DIRECTION ( 'NONE',  ( 0.000000000000000000, 0.000000000000000000, 1.000000000000000000 ) ) ;
#70994=ORIENTED_EDGE ( 'NONE', *, *, #27789, .T. ) ;
#71008=CIRCLE ( 'NONE', #10325, 0.2500000000000002220 ) ;
#71012=CARTESIAN_POINT ( 'NONE',  ( -19.89999999999999858, 92.00000000000000000, -7.750000000000000000 ) ) ;
#71020=CIRCLE ( 'NONE', #31094, 1.249999999999987121 ) ;
#71026=ORIENTED_EDGE ( 'NONE', *, *, #67589, .F. ) ;
#71031=( NAMED_UNIT ( * ) PLANE_ANGLE_UNIT ( ) SI_UNIT ( $, .RADIAN. ) );
#71039=EDGE_CURVE ( 'NONE', #8055, #55012, #67730, .T. ) ;
#71043=CARTESIAN_POINT ( 'NONE',  ( -7.750000000000000000, 80.32179676972448590, 4.250000000000000000 ) ) ;
#71056=DIRECTION ( 'NONE',  ( 1.000000000000000000, 0.000000000000000000, 0.000000000000000000 ) ) ;
#71078=CARTESIAN_POINT ( 'NONE',  ( -11.05191079938453491, -57.06817940849906989, 4.000000000000000000 ) ) ;
#71079=( NAMED_UNIT ( * ) SI_UNIT ( $, .STERADIAN. ) SOLID_ANGLE_UNIT ( ) );
#71083=STYLED_ITEM ( 'NONE', ( #98277 ), #7689 ) ;
#71084=CARTESIAN_POINT ( 'NONE',  ( -13.69999999999999751, 99.99999999999998579, 8.000000000000000000 ) ) ;
#71088=DIRECTION ( 'NONE',  ( 0.000000000000000000, -0.000000000000000000, -1.000000000000000000 ) ) ;
#71102=( GEOMETRIC_REPRESENTATION_CONTEXT ( 3 ) GLOBAL_UNCERTAINTY_ASSIGNED_CONTEXT ( ( #81287 ) ) GLOBAL_UNIT_ASSIGNED_CONTEXT ( ( #85310, #9808, #40309 ) ) REPRESENTATION_CONTEXT ( 'NONE', 'WORKASPACE' ) );
#71103=LINE ( 'NONE', #25128, #19393 ) ;
#71124=CARTESIAN_POINT ( 'NONE',  ( 3.969999999999999751, 10.25000000000000000, 2.500000000000000000 ) ) ;
#71126=ORIENTED_EDGE ( 'NONE', *, *, #52183, .T. ) ;
#71135=ORIENTED_EDGE ( 'NONE', *, *, #89073, .T. ) ;
#71150=CARTESIAN_POINT ( 'NONE',  ( -5.328486666281220252, -28.65465727419596931, 2.499999999998389288 ) ) ;
#71152=CARTESIAN_POINT ( 'NONE',  ( -6.732636091893168029, -88.11213685669366669, 3.250000000000000000 ) ) ;
#71157=ORIENTED_EDGE ( 'NONE', *, *, #26397, .F. ) ;
#71163=ORIENTED_EDGE ( 'NONE', *, *, #82772, .T. ) ;
#71166=PLANE ( 'NONE',  #57906 ) ;
#71179=CARTESIAN_POINT ( 'NONE',  ( 1.379999999999981908, 20.99999999999999645, 0.000000000000000000 ) ) ;
#71181=LINE ( 'NONE', #57518, #4489 ) ;
#71225=FILL_AREA_STYLE ('',( #77234 ) ) ;
#71229=DIRECTION ( 'NONE',  ( 1.000000000000000000, 0.000000000000000000, 0.000000000000000000 ) ) ;
#71236=EDGE_CURVE ( 'NONE', #69773, #41505, #66930, .T. ) ;
#71241=ORIENTED_EDGE ( 'NONE', *, *, #4005, .F. ) ;
#71265=( GEOMETRIC_REPRESENTATION_CONTEXT ( 3 ) GLOBAL_UNCERTAINTY_ASSIGNED_CONTEXT ( ( #15139 ) ) GLOBAL_UNIT_ASSIGNED_CONTEXT ( ( #11881, #14355, #54301 ) ) REPRESENTATION_CONTEXT ( 'NONE', 'WORKASPACE' ) );
#71273=AXIS2_PLACEMENT_3D ( 'NONE', #74075, #18632, #51091 ) ;
#71274=CARTESIAN_POINT ( 'NONE',  ( 15.00000000000000000, 77.07179676972447169, -4.250000000000000000 ) ) ;
#71283=SURFACE_STYLE_USAGE ( .BOTH. , #65223 ) ;
#71295=( GEOMETRIC_REPRESENTATION_CONTEXT ( 3 ) GLOBAL_UNCERTAINTY_ASSIGNED_CONTEXT ( ( #40475 ) ) GLOBAL_UNIT_ASSIGNED_CONTEXT ( ( #19141, #3658, #64127 ) ) REPRESENTATION_CONTEXT ( 'NONE', 'WORKASPACE' ) );
#71313=DIRECTION ( 'NONE',  ( 0.9997628902338895340, -0.02177529129954166101, 0.000000000000000000 ) ) ;
#71317=( NAMED_UNIT ( * ) PLANE_ANGLE_UNIT ( ) SI_UNIT ( $, .RADIAN. ) );
#71318=SURFACE_STYLE_FILL_AREA ( #70833 ) ;
#71333=DIRECTION ( 'NONE',  ( -0.000000000000000000, -0.000000000000000000, -1.000000000000000000 ) ) ;
#71335=SURFACE_STYLE_FILL_AREA ( #85843 ) ;
#71337=FILL_AREA_STYLE ('',( #78828 ) ) ;
#71343=MECHANICAL_DESIGN_GEOMETRIC_PRESENTATION_REPRESENTATION('',(#1050),#13810);
#71350=DIRECTION ( 'NONE',  ( -0.000000000000000000, 1.000000000000000000, 0.000000000000000000 ) ) ;
#71374=AXIS2_PLACEMENT_3D ( 'NONE', #41052, #26044, #71056 ) ;
#71384=ORIENTED_EDGE ( 'NONE', *, *, #74797, .T. ) ;
#71394=ORIENTED_EDGE ( 'NONE', *, *, #89313, .F. ) ;
#71402=CARTESIAN_POINT ( 'NONE',  ( -8.469568049931512022, -9.365055636449845622, 3.750000000000000000 ) ) ;
#71409=SURFACE_STYLE_USAGE ( .BOTH. , #62397 ) ;
#71411=ORIENTED_EDGE ( 'NONE', *, *, #47439, .T. ) ;
#71413=DIRECTION ( 'NONE',  ( 1.000000000000000000, 0.000000000000000000, 0.000000000000000000 ) ) ;
#71417=AXIS2_PLACEMENT_3D ( 'NONE', #68580, #111, #68088 ) ;
#71436=AXIS2_PLACEMENT_3D ( 'NONE', #10845, #76508, #23529 ) ;
#71439=EDGE_LOOP ( 'NONE', ( #10537, #31929, #16000, #313 ) ) ;
#71441=LINE ( 'NONE', #85948, #69412 ) ;
#71442=CARTESIAN_POINT ( 'NONE',  ( -5.068142462349377375, -24.94450071862243590, -2.750000000000000000 ) ) ;
#71446=DIRECTION ( 'NONE',  ( -0.000000000000000000, -0.000000000000000000, 1.000000000000000000 ) ) ;
#71465=UNCERTAINTY_MEASURE_WITH_UNIT (LENGTH_MEASURE( 1.000000000000000082E-05 ), #89494, 'distance_accuracy_value', 'NONE');
#71482=STYLED_ITEM ( 'NONE', ( #91588 ), #44265 ) ;
#71498=EDGE_CURVE ( 'NONE', #36998, #22141, #98927, .T. ) ;
#71499=CARTESIAN_POINT ( 'NONE',  ( -11.51437862373891363, -65.40122319151942065, -3.750000000000001332 ) ) ;
#71504=AXIS2_PLACEMENT_3D ( 'NONE', #33701, #64201, #94717 ) ;
#71505=ORIENTED_EDGE ( 'NONE', *, *, #79727, .F. ) ;
#71513=STYLED_ITEM ( 'NONE', ( #28001 ), #58355 ) ;
#71523=ORIENTED_EDGE ( 'NONE', *, *, #66402, .F. ) ;
#71537=EDGE_LOOP ( 'NONE', ( #10013, #56604, #88791 ) ) ;
#71545=ORIENTED_EDGE ( 'NONE', *, *, #84364, .T. ) ;
#71568=FILL_AREA_STYLE ('',( #41073 ) ) ;
#71573=CARTESIAN_POINT ( 'NONE',  ( -10.95094547650107053, -94.44763431416065202, 3.999999999999999112 ) ) ;
#71574=DIRECTION ( 'NONE',  ( 0.000000000000000000, -1.000000000000000000, 0.000000000000000000 ) ) ;
#71579=CARTESIAN_POINT ( 'NONE',  ( -7.750000000000000000, 80.32179676972448590, -3.750000000000000000 ) ) ;
#71587=EDGE_LOOP ( 'NONE', ( #15313, #96845, #79015, #81978 ) ) ;
#71598=SURFACE_STYLE_USAGE ( .BOTH. , #17611 ) ;
#71601=VERTEX_POINT ( 'NONE', #47269 ) ;
#71604=ADVANCED_FACE ( 'NONE', ( #40772 ), #6194, .F. ) ;
#71606=CARTESIAN_POINT ( 'NONE',  ( -13.77612262535527954, 90.93158326518027934, 7.883772450803742338 ) ) ;
#71614=ORIENTED_EDGE ( 'NONE', *, *, #29040, .F. ) ;
#71617=VERTEX_POINT ( 'NONE', #25774 ) ;
#71626=ORIENTED_EDGE ( 'NONE', *, *, #15726, .F. ) ;
#71634=EDGE_CURVE ( 'NONE', #49831, #43714, #60498, .T. ) ;
#71635=STYLED_ITEM ( 'NONE', ( #12811 ), #59675 ) ;
#71641=CARTESIAN_POINT ( 'NONE',  ( 10.83696084481538868, -98.17058944465519232, 4.000000000000000000 ) ) ;
#71645=CARTESIAN_POINT ( 'NONE',  ( -6.841090228438033272, -58.65898919720570603, 3.750000000000000444 ) ) ;
#71657=FACE_OUTER_BOUND ( 'NONE', #90684, .T. ) ;
#71667=FACE_OUTER_BOUND ( 'NONE', #50697, .T. ) ;
#71673=CARTESIAN_POINT ( 'NONE',  ( -11.26386101273796925, -65.37750071430100718, -4.000000000000000000 ) ) ;
#71675=LINE ( 'NONE', #3185, #3293 ) ;
#71677=EDGE_CURVE ( 'NONE', #68087, #62473, #55726, .T. ) ;
#71704=CIRCLE ( 'NONE', #98511, 10.90000000000000036 ) ;
#71706=ORIENTED_EDGE ( 'NONE', *, *, #25227, .F. ) ;
#71710=SURFACE_SIDE_STYLE ('',( #62226 ) ) ;
#71724=CARTESIAN_POINT ( 'NONE',  ( -5.320324007936277688, -24.96642978969368443, 3.999999999999999112 ) ) ;
#71742=VERTEX_POINT ( 'NONE', #27221 ) ;
#71744=AXIS2_PLACEMENT_3D ( 'NONE', #39617, #9596, #24120 ) ;
#71763=( NAMED_UNIT ( * ) PLANE_ANGLE_UNIT ( ) SI_UNIT ( $, .RADIAN. ) );
#71774=CARTESIAN_POINT ( 'NONE',  ( -9.297374403301716939, 88.08016496434417775, 4.860721439949188039 ) ) ;
#71784=PRESENTATION_STYLE_ASSIGNMENT (( #79285 ) ) ;
#71788=( LENGTH_UNIT ( ) NAMED_UNIT ( * ) SI_UNIT ( .MILLI., .METRE. ) );
#71799=LINE ( 'NONE', #2835, #88256 ) ;
#71800=DIRECTION ( 'NONE',  ( 0.000000000000000000, 0.000000000000000000, 1.000000000000000000 ) ) ;
#71807=ORIENTED_EDGE ( 'NONE', *, *, #16284, .F. ) ;
#71808=DIRECTION ( 'NONE',  ( 1.000000000000000000, 0.000000000000000000, 0.000000000000000000 ) ) ;
#71814=CARTESIAN_POINT ( 'NONE',  ( 8.862914611995314829, -7.247476534008700177, -4.000000000000000888 ) ) ;
#71818=LINE ( 'NONE', #3325, #3258 ) ;
#71840=ORIENTED_EDGE ( 'NONE', *, *, #48770, .T. ) ;
#71880=CARTESIAN_POINT ( 'NONE',  ( -15.00000000000000000, 83.99999999999998579, -7.750000000000000000 ) ) ;
#71885=CARTESIAN_POINT ( 'NONE',  ( -13.79463296483944923, 90.89544289844283753, 7.796684565667933775 ) ) ;
#71896=CARTESIAN_POINT ( 'NONE',  ( 6.933985542721516460, -73.15302115705439689, 2.749999999998391065 ) ) ;
#71900=CARTESIAN_POINT ( 'NONE',  ( 8.879999999999999005, -0.01540240839183078247, 3.750000000000000444 ) ) ;
#71913=( LENGTH_UNIT ( ) NAMED_UNIT ( * ) SI_UNIT ( .MILLI., .METRE. ) );
#71919=CIRCLE ( 'NONE', #24049, 0.5000000000000004441 ) ;
#71920=CARTESIAN_POINT ( 'NONE',  ( 6.284516029235898138, -36.06297093898795936, -4.000000000000000000 ) ) ;
#71922=DIRECTION ( 'NONE',  ( 1.000000000000000000, 0.000000000000000000, 0.000000000000000000 ) ) ;
#71923=CARTESIAN_POINT ( 'NONE',  ( -4.787136363774558312, -17.54594992866426395, 4.000000000000000888 ) ) ;
#71926=FACE_OUTER_BOUND ( 'NONE', #84775, .T. ) ;
#71930=CARTESIAN_POINT ( 'NONE',  ( 8.629999999999995453, 41.24999999999999289, 6.500000000000000888 ) ) ;
#71947=EDGE_CURVE ( 'NONE', #6107, #52027, #44506, .T. ) ;
#71973=VERTEX_POINT ( 'NONE', #52204 ) ;
#71985=CYLINDRICAL_SURFACE ( 'NONE', #40984, 0.2500000000000002220 ) ;
#72001=EDGE_LOOP ( 'NONE', ( #75825, #53579, #60772, #92246 ) ) ;
#72009=CARTESIAN_POINT ( 'NONE',  ( 8.879999999999991900, 69.99999999999998579, 6.396446609406726935 ) ) ;
#72016=AXIS2_PLACEMENT_3D ( 'NONE', #17809, #25326, #49279 ) ;
#72027=EDGE_LOOP ( 'NONE', ( #86540, #3409, #94445, #72823 ) ) ;
#72035=CARTESIAN_POINT ( 'NONE',  ( -13.34727560011345027, 90.86036091889431532, 7.765078796629374835 ) ) ;
#72044=CARTESIAN_POINT ( 'NONE',  ( -11.05192081855304309, -57.06859629180129900, -4.000000000000000888 ) ) ;
#72045=CARTESIAN_POINT ( 'NONE',  ( -7.858200837834798946, -3.137962441252946544, 4.000000000000000888 ) ) ;
#72069=CARTESIAN_POINT ( 'NONE',  ( -7.750000000000000000, 1.019547802438458550, -3.750000000000000000 ) ) ;
#72072=CARTESIAN_POINT ( 'NONE',  ( 8.629999999999995453, 43.00000000000000000, 6.500000000000000888 ) ) ;
#72074=ORIENTED_EDGE ( 'NONE', *, *, #44949, .F. ) ;
#72088=( LENGTH_UNIT ( ) NAMED_UNIT ( * ) SI_UNIT ( .MILLI., .METRE. ) );
#72096=LINE ( 'NONE', #63606, #43022 ) ;
#72100=ORIENTED_EDGE ( 'NONE', *, *, #63870, .T. ) ;
#72109=SURFACE_SIDE_STYLE ('',( #20097 ) ) ;
#72111=VERTEX_POINT ( 'NONE', #13712 ) ;
#72114=DIRECTION ( 'NONE',  ( 0.009903002720634835818, -0.9999509640662961329, 0.000000000000000000 ) ) ;
#72116=CARTESIAN_POINT ( 'NONE',  ( -6.000000000000000000, 78.07179676972447169, -4.250000000000000000 ) ) ;
#72118=LINE ( 'NONE', #3646, #31518 ) ;
#72135=ADVANCED_FACE ( 'NONE', ( #44195, #74705 ), #29196, .T. ) ;
#72136=ORIENTED_EDGE ( 'NONE', *, *, #19227, .T. ) ;
#72137=EDGE_CURVE ( 'NONE', #11101, #94992, #87675, .T. ) ;
#72152=CARTESIAN_POINT ( 'NONE',  ( -7.750000000000000000, 80.07179676972448590, -6.500000000000000888 ) ) ;
#72160=AXIS2_PLACEMENT_3D ( 'NONE', #24753, #94211, #56233 ) ;
#72165=ADVANCED_FACE ( 'NONE', ( #32643 ), #85167, .F. ) ;
#72199=VECTOR ( 'NONE', #63526, 1000.000000000000000 ) ;
#72206=STYLED_ITEM ( 'NONE', ( #4423 ), #75723 ) ;
#72207=ORIENTED_EDGE ( 'NONE', *, *, #96222, .F. ) ;
#72213=CARTESIAN_POINT ( 'NONE',  ( 18.00000000000000355, 73.00000000000001421, -6.250000000000000000 ) ) ;
#72217=ORIENTED_EDGE ( 'NONE', *, *, #57021, .F. ) ;
#72238=CARTESIAN_POINT ( 'NONE',  ( -8.900000000000002132, 80.99999999999994316, 0.000000000000000000 ) ) ;
#72242=PLANE ( 'NONE',  #42107 ) ;
#72257=CIRCLE ( 'NONE', #6825, 0.2500000000000002220 ) ;
#72266=DIRECTION ( 'NONE',  ( -0.000000000000000000, 0.000000000000000000, 1.000000000000000000 ) ) ;
#72272=TOROIDAL_SURFACE ( 'NONE', #24193, 3.250000000000001332, 0.2500000000000000000 ) ;
#72286=AXIS2_PLACEMENT_3D ( 'NONE', #75680, #90180, #90677 ) ;
#72291=EDGE_CURVE ( 'NONE', #12076, #74689, #71704, .T. ) ;
#72292=CARTESIAN_POINT ( 'NONE',  ( 11.04400142266738882, -89.88311504653209738, -3.999999999999999112 ) ) ;
#72298=ADVANCED_FACE ( 'NONE', ( #31164 ), #41785, .T. ) ;
#72319=COLOUR_RGB ( '', 0.72549020, 0.75294118, 0.79215686) ;
#72320=ORIENTED_EDGE ( 'NONE', *, *, #30401, .T. ) ;
#72338=CARTESIAN_POINT ( 'NONE',  ( 9.779999999999994031, 1.885066177228129719E-15, 2.900000000000000355 ) ) ;
#72341=EDGE_CURVE ( 'NONE', #16571, #10746, #21832, .T. ) ;
#72357=LINE ( 'NONE', #86884, #13284 ) ;
#72364=VECTOR ( 'NONE', #97979, 1000.000000000000000 ) ;
#72372=VERTEX_POINT ( 'NONE', #475 ) ;
#72377=B_SPLINE_CURVE_WITH_KNOTS ( 'NONE', 3,
 ( #67472, #6971, #90446, #21985, #52460, #37478, #60938, #29946, #60452, #22471, #52947, #83457, #14978, #45449, #75951, #7478, #91449, #22972, #15474, #24444 ),
 .UNSPECIFIED., .F., .F.,
 ( 4, 2, 2, 2, 2, 2, 2, 2, 2, 4 ),
 ( 0.000000000000000000, 0.001321439349356821023, 0.002642878698713642047, 0.003964318048070463070, 0.005285757397427284093, 0.006607196746784105117, 0.007928636096140926140, 0.009250075445497746296, 0.009910795120176157241, 0.01057151479485456819 ),
 .UNSPECIFIED. ) ;
#72382=CARTESIAN_POINT ( 'NONE',  ( 6.933985542757959308, -73.15302115705439689, 2.499999999997586375 ) ) ;
#72391=( GEOMETRIC_REPRESENTATION_CONTEXT ( 3 ) GLOBAL_UNCERTAINTY_ASSIGNED_CONTEXT ( ( #66475 ) ) GLOBAL_UNIT_ASSIGNED_CONTEXT ( ( #67377, #37392, #14892 ) ) REPRESENTATION_CONTEXT ( 'NONE', 'WORKASPACE' ) );
#72393=CARTESIAN_POINT ( 'NONE',  ( -3.500000000000000444, 0.09224605989684696306, -2.750000000000000000 ) ) ;
#72402=CARTESIAN_POINT ( 'NONE',  ( 6.934035614042552531, -73.16521313705239038, -3.999999999998390177 ) ) ;
#72405=DIRECTION ( 'NONE',  ( 0.000000000000000000, 0.000000000000000000, -1.000000000000000000 ) ) ;
#72414=CYLINDRICAL_SURFACE ( 'NONE', #81186, 0.2500000000000002220 ) ;
#72416=EDGE_CURVE ( 'NONE', #23594, #6107, #6961, .T. ) ;
#72423=CARTESIAN_POINT ( 'NONE',  ( -6.000000000000009770, 40.99999999999999289, -4.250000000000000000 ) ) ;
#72426=CYLINDRICAL_SURFACE ( 'NONE', #33448, 0.1000000000000001166 ) ;
#72433=ORIENTED_EDGE ( 'NONE', *, *, #78891, .F. ) ;
#72441=DIRECTION ( 'NONE',  ( -0.000000000000000000, -0.000000000000000000, 1.000000000000000000 ) ) ;
#72454=EDGE_LOOP ( 'NONE', ( #85261, #1129, #19332, #51824, #93526, #43540 ) ) ;
#72463=EDGE_CURVE ( 'NONE', #92371, #42155, #39222, .T. ) ;
#72465=EDGE_CURVE ( 'NONE', #19716, #538, #87257, .T. ) ;
#72472=CARTESIAN_POINT ( 'NONE',  ( -10.44999999999999751, 99.99999999999998579, -8.525133428036873795 ) ) ;
#72493=EDGE_CURVE ( 'NONE', #13062, #16387, #61700, .T. ) ;
#72506=CARTESIAN_POINT ( 'NONE',  ( -3.250000000000000444, 1.019547802438453887, 2.750000000000000444 ) ) ;
#72511=VERTEX_POINT ( 'NONE', #8433 ) ;
#72520=DIRECTION ( 'NONE',  ( 0.000000000000000000, 0.000000000000000000, 1.000000000000000000 ) ) ;
#72552=PLANE ( 'NONE',  #81622 ) ;
#72553=CARTESIAN_POINT ( 'NONE',  ( -3.586264863366058542, -2.711807932106038876, -3.750000000000000000 ) ) ;
#72569=( LENGTH_UNIT ( ) NAMED_UNIT ( * ) SI_UNIT ( .MILLI., .METRE. ) );
#72570=EDGE_CURVE ( 'NONE', #38899, #75564, #46911, .T. ) ;
#72578=AXIS2_PLACEMENT_3D ( 'NONE', #86230, #1283, #17741 ) ;
#72591=DIRECTION ( 'NONE',  ( 0.000000000000000000, 0.000000000000000000, 1.000000000000000000 ) ) ;
#72598=CARTESIAN_POINT ( 'NONE',  ( 11.19532980483368867, -77.48602862273223479, 4.000000000000000000 ) ) ;
#72604=LINE ( 'NONE', #87614, #38029 ) ;
#72605=DIRECTION ( 'NONE',  ( 1.000000000000000000, 0.000000000000000000, 0.000000000000000000 ) ) ;
#72606=CARTESIAN_POINT ( 'NONE',  ( 17.75000000000000355, 78.80384757729336798, 3.750000000000000000 ) ) ;
#72618=DIRECTION ( 'NONE',  ( -0.000000000000000000, -0.000000000000000000, -1.000000000000000000 ) ) ;
#72627=CARTESIAN_POINT ( 'NONE',  ( 4.469999999999999751, 36.75000000000000000, 3.750000000000000000 ) ) ;
#72634=CARTESIAN_POINT ( 'NONE',  ( -10.77730536144846774, -98.63085534186637915, -3.999999999999996447 ) ) ;
#72639=CARTESIAN_POINT ( 'NONE',  ( 6.910406350442640289, -84.29253233655508382, -3.750000000000000444 ) ) ;
#72651=ORIENTED_EDGE ( 'NONE', *, *, #30401, .F. ) ;
#72653=CARTESIAN_POINT ( 'NONE',  ( 6.533420211785746723, -50.31490269211863620, 2.750000000000000000 ) ) ;
#72663=EDGE_CURVE ( 'NONE', #25669, #95488, #10403, .T. ) ;
#72667=ORIENTED_EDGE ( 'NONE', *, *, #51090, .T. ) ;
#72682=FACE_OUTER_BOUND ( 'NONE', #62292, .T. ) ;
#72685=DIRECTION ( 'NONE',  ( -0.000000000000000000, -0.000000000000000000, -1.000000000000000000 ) ) ;
#72686=ORIENTED_EDGE ( 'NONE', *, *, #58130, .F. ) ;
#72701=ORIENTED_EDGE ( 'NONE', *, *, #20806, .F. ) ;
#72707=FACE_OUTER_BOUND ( 'NONE', #84444, .T. ) ;
#72715=ADVANCED_FACE ( 'NONE', ( #17908 ), #10625, .T. ) ;
#72720=ADVANCED_FACE ( 'NONE', ( #47895, #32398 ), #54901, .T. ) ;
#72722=CARTESIAN_POINT ( 'NONE',  ( -10.53011945866294852, -98.59345040283277228, -3.750000000000000000 ) ) ;
#72736=AXIS2_PLACEMENT_3D ( 'NONE', #30438, #90941, #74462 ) ;
#72749=SURFACE_STYLE_USAGE ( .BOTH. , #59231 ) ;
#72752=SURFACE_SIDE_STYLE ('',( #64754 ) ) ;
#72753=SURFACE_STYLE_USAGE ( .BOTH. , #20267 ) ;
#72757=DIRECTION ( 'NONE',  ( 0.7808688094430307203, -0.6246950475544238435, 0.000000000000000000 ) ) ;
#72758=EDGE_LOOP ( 'NONE', ( #77655, #48863, #89424, #34175 ) ) ;
#72761=DIRECTION ( 'NONE',  ( 0.7971177707001108059, 0.6038238647437559337, -1.106223127961422775E-14 ) ) ;
#72768=ORIENTED_EDGE ( 'NONE', *, *, #7540, .T. ) ;
#72775=CARTESIAN_POINT ( 'NONE',  ( 10.69986656896780275, -97.11187948767582157, -3.999999999999999112 ) ) ;
#72778=SURFACE_SIDE_STYLE ('',( #42306 ) ) ;
#72779=DIRECTION ( 'NONE',  ( 0.000000000000000000, 0.000000000000000000, -1.000000000000000000 ) ) ;
#72782=MECHANICAL_DESIGN_GEOMETRIC_PRESENTATION_REPRESENTATION('',(#24859),#39279);
#72792=DIRECTION ( 'NONE',  ( 0.000000000000000000, 0.000000000000000000, -1.000000000000000000 ) ) ;
#72797=CARTESIAN_POINT ( 'NONE',  ( -4.250000000000000000, 10.25000000000000000, 4.000000000000000000 ) ) ;
#72801=ORIENTED_EDGE ( 'NONE', *, *, #52388, .F. ) ;
#72809=ORIENTED_EDGE ( 'NONE', *, *, #21121, .T. ) ;
#72823=ORIENTED_EDGE ( 'NONE', *, *, #30963, .F. ) ;
#72842=DIRECTION ( 'NONE',  ( 1.000000000000000000, 0.000000000000000000, 0.000000000000000000 ) ) ;
#72849=DIRECTION ( 'NONE',  ( -0.000000000000000000, 0.000000000000000000, 1.000000000000000000 ) ) ;
#72864=MECHANICAL_DESIGN_GEOMETRIC_PRESENTATION_REPRESENTATION('',(#87220),#42543);
#72868=CARTESIAN_POINT ( 'NONE',  ( -7.750355510519348456, 84.07179676972448590, -4.000000000000000000 ) ) ;
#72872=PLANE ( 'NONE',  #3154 ) ;
#72885=VERTEX_POINT ( 'NONE', #81351 ) ;
#72887=VECTOR ( 'NONE', #65585, 1000.000000000000000 ) ;
#72889=CARTESIAN_POINT ( 'NONE',  ( -5.809210876199116136, -36.07757871006175776, -2.749999999999193978 ) ) ;
#72896=ORIENTED_EDGE ( 'NONE', *, *, #74405, .T. ) ;
#72897=CARTESIAN_POINT ( 'NONE',  ( 8.629999999999995453, 40.74999999999999289, 4.000000000000000000 ) ) ;
#72899=FILL_AREA_STYLE_COLOUR ( '', #41056 ) ;
#72934=CARTESIAN_POINT ( 'NONE',  ( -8.000000000000000000, 1.019547802438458550, -3.750000000000000000 ) ) ;
#72939=LINE ( 'NONE', #26454, #61657 ) ;
#72966=FACE_OUTER_BOUND ( 'NONE', #56472, .T. ) ;
#72981=STYLED_ITEM ( 'NONE', ( #2626 ), #67807 ) ;
#72990=SURFACE_SIDE_STYLE ('',( #19507 ) ) ;
#73021=DIRECTION ( 'NONE',  ( 1.000000000000000000, 0.000000000000000000, 0.000000000000000000 ) ) ;
#73026=EDGE_CURVE ( 'NONE', #81557, #24768, #17986, .T. ) ;
#73031=CARTESIAN_POINT ( 'NONE',  ( -8.099999999999999645, 80.99999999999994316, 0.000000000000000000 ) ) ;
#73033=ORIENTED_EDGE ( 'NONE', *, *, #28948, .T. ) ;
#73043=CARTESIAN_POINT ( 'NONE',  ( 1.350000000000004086, 98.49999999999998579, 8.000000000000000000 ) ) ;
#73045=EDGE_CURVE ( 'NONE', #16383, #80582, #23959, .T. ) ;
#73050=ORIENTED_EDGE ( 'NONE', *, *, #64578, .T. ) ;
#73061=EDGE_CURVE ( 'NONE', #95449, #61040, #43516, .T. ) ;
#73084=SURFACE_STYLE_FILL_AREA ( #18627 ) ;
#73093=DIRECTION ( 'NONE',  ( -1.000000000000000000, 0.000000000000000000, 0.000000000000000000 ) ) ;
#73094=AXIS2_PLACEMENT_3D ( 'NONE', #4718, #73674, #5205 ) ;
#73100=DIRECTION ( 'NONE',  ( -0.000000000000000000, 0.000000000000000000, 1.000000000000000000 ) ) ;
#73109=AXIS2_PLACEMENT_3D ( 'NONE', #73177, #43183, #73670 ) ;
#73110=CARTESIAN_POINT ( 'NONE',  ( -13.69999999999999751, 99.99999999999998579, -8.525133428036873795 ) ) ;
#73119=FACE_OUTER_BOUND ( 'NONE', #11983, .T. ) ;
#73126=CARTESIAN_POINT ( 'NONE',  ( -11.58434547253664171, -69.53046085282439037, -3.750000000000000000 ) ) ;
#73140=EDGE_CURVE ( 'NONE', #75803, #53272, #46450, .T. ) ;
#73151=STYLED_ITEM ( 'NONE', ( #41820 ), #2776 ) ;
#73152=CARTESIAN_POINT ( 'NONE',  ( -9.990730578767625047, 46.91630561652143427, 2.900000000000000355 ) ) ;
#73157=ORIENTED_EDGE ( 'NONE', *, *, #13212, .T. ) ;
#73158=UNCERTAINTY_MEASURE_WITH_UNIT (LENGTH_MEASURE( 1.000000000000000082E-05 ), #3395, 'distance_accuracy_value', 'NONE');
#73159=( NAMED_UNIT ( * ) PLANE_ANGLE_UNIT ( ) SI_UNIT ( $, .RADIAN. ) );
#73170=CARTESIAN_POINT ( 'NONE',  ( -10.77730536144846596, -98.63085534186639336, 3.750000000000000000 ) ) ;
#73177=CARTESIAN_POINT ( 'NONE',  ( 3.969999999999999751, 10.25000000000000000, 2.750000000000000000 ) ) ;
#73188=( GEOMETRIC_REPRESENTATION_CONTEXT ( 3 ) GLOBAL_UNCERTAINTY_ASSIGNED_CONTEXT ( ( #59269 ) ) GLOBAL_UNIT_ASSIGNED_CONTEXT ( ( #28776, #96812, #11805 ) ) REPRESENTATION_CONTEXT ( 'NONE', 'WORKASPACE' ) );
#73191=TOROIDAL_SURFACE ( 'NONE', #65194, 2.250000000000001332, 0.2500000000000000000 ) ;
#73239=CARTESIAN_POINT ( 'NONE',  ( 6.829574850505126804, -88.00372650098204019, 2.750000000000002665 ) ) ;
#73244=CIRCLE ( 'NONE', #57259, 2.000000000000000888 ) ;
#73252=SURFACE_STYLE_USAGE ( .BOTH. , #72752 ) ;
#73254=VECTOR ( 'NONE', #10131, 1000.000000000000000 ) ;
#73260=CARTESIAN_POINT ( 'NONE',  ( -3.585700530862828028, -2.697939587593689570, 2.750000000000001332 ) ) ;
#73265=CARTESIAN_POINT ( 'NONE',  ( -11.13303098458958296, 89.96146600687833939, -6.578309274437964760 ) ) ;
#73267=CARTESIAN_POINT ( 'NONE',  ( 0.4400000000000020006, 1.019547802438468986, 2.750000000000000000 ) ) ;
#73273=DIRECTION ( 'NONE',  ( -1.000000000000000000, 0.000000000000000000, 0.000000000000000000 ) ) ;
#73289=ORIENTED_EDGE ( 'NONE', *, *, #84582, .T. ) ;
#73297=FACE_OUTER_BOUND ( 'NONE', #9114, .T. ) ;
#73306=EDGE_LOOP ( 'NONE', ( #21534, #27538, #54396, #63567 ) ) ;
#73346=DIRECTION ( 'NONE',  ( 0.000000000000000000, 0.000000000000000000, -1.000000000000000000 ) ) ;
#73362=CARTESIAN_POINT ( 'NONE',  ( -10.19302435262559037, 44.02336987076795083, 0.000000000000000000 ) ) ;
#73374=DIRECTION ( 'NONE',  ( 1.000000000000000000, -0.000000000000000000, -0.000000000000000000 ) ) ;
#73380=CARTESIAN_POINT ( 'NONE',  ( -6.874974626955391521, -78.82095024088569346, -2.500000000000000000 ) ) ;
#73392=DIRECTION ( 'NONE',  ( 0.000000000000000000, -0.000000000000000000, 1.000000000000000000 ) ) ;
#73397=DIRECTION ( 'NONE',  ( -1.000000000000000000, 0.000000000000000000, 0.000000000000000000 ) ) ;
#73400=( NAMED_UNIT ( * ) PLANE_ANGLE_UNIT ( ) SI_UNIT ( $, .RADIAN. ) );
#73407=ORIENTED_EDGE ( 'NONE', *, *, #59118, .F. ) ;
#73408=LINE ( 'NONE', #4936, #30933 ) ;
#73417=ORIENTED_EDGE ( 'NONE', *, *, #1883, .F. ) ;
#73429=CARTESIAN_POINT ( 'NONE',  ( 6.879999999999995453, 43.00000000000000000, -4.250000000000000000 ) ) ;
#73437=ORIENTED_EDGE ( 'NONE', *, *, #81638, .T. ) ;
#73441=TOROIDAL_SURFACE ( 'NONE', #38350, 4.250000000000001776, 0.2500000000000000000 ) ;
#73449=DIRECTION ( 'NONE',  ( 1.000000000000000000, 0.000000000000000000, -0.000000000000000000 ) ) ;
#73452=DIRECTION ( 'NONE',  ( 1.000000000000000000, -0.000000000000000000, 0.000000000000000000 ) ) ;
#73461=CARTESIAN_POINT ( 'NONE',  ( -7.121341127193570486, -73.24353698637885657, 2.750000000000000000 ) ) ;
#73469=CARTESIAN_POINT ( 'NONE',  ( 4.823525747195464675, -6.402798798525323853, 4.000000000000000888 ) ) ;
#73485=AXIS2_PLACEMENT_3D ( 'NONE', #57713, #80721, #73697 ) ;
#73489=CARTESIAN_POINT ( 'NONE',  ( 18.00000000000000000, 78.20644476077552554, 3.828778331633460486 ) ) ;
#73494=EDGE_CURVE ( 'NONE', #82286, #9027, #3576, .T. ) ;
#73509=DIRECTION ( 'NONE',  ( 1.000000000000000000, 0.000000000000000000, 0.000000000000000000 ) ) ;
#73515=CARTESIAN_POINT ( 'NONE',  ( 18.00000000000000000, 77.07179676972447169, -4.250000000000000000 ) ) ;
#73521=LINE ( 'NONE', #59020, #30440 ) ;
#73522=( LENGTH_UNIT ( ) NAMED_UNIT ( * ) SI_UNIT ( .MILLI., .METRE. ) );
#73539=FILL_AREA_STYLE ('',( #51045 ) ) ;
#73541=VERTEX_POINT ( 'NONE', #22901 ) ;
#73554=AXIS2_PLACEMENT_3D ( 'NONE', #88037, #71088, #2613 ) ;
#73558=ORIENTED_EDGE ( 'NONE', *, *, #34321, .T. ) ;
#73568=ORIENTED_EDGE ( 'NONE', *, *, #88988, .T. ) ;
#73576=CARTESIAN_POINT ( 'NONE',  ( -18.00000000000000355, 75.73428692542562146, 3.000000000000000000 ) ) ;
#73581=DIRECTION ( 'NONE',  ( 0.000000000000000000, 0.000000000000000000, 1.000000000000000000 ) ) ;
#73587=EDGE_CURVE ( 'NONE', #60629, #50168, #59435, .T. ) ;
#73596=ORIENTED_EDGE ( 'NONE', *, *, #1051, .T. ) ;
#73599=ADVANCED_FACE ( 'NONE', ( #87187 ), #3712, .F. ) ;
#73604=CARTESIAN_POINT ( 'NONE',  ( 8.879999999999995453, 40.74999999999999289, -3.750000000000000000 ) ) ;
#73607=DIRECTION ( 'NONE',  ( -0.5905099943842175847, -0.8070303256584298035, 0.000000000000000000 ) ) ;
#73614=VECTOR ( 'NONE', #93576, 1000.000000000000114 ) ;
#73625=CARTESIAN_POINT ( 'NONE',  ( -11.23890517432719882, -88.22482801183184620, -4.000000000000000000 ) ) ;
#73630=FILL_AREA_STYLE ('',( #57646 ) ) ;
#73638=ORIENTED_EDGE ( 'NONE', *, *, #92714, .F. ) ;
#73640=CARTESIAN_POINT ( 'NONE',  ( 17.88864439015886276, 91.03707094060693805, -8.000000000000000000 ) ) ;
#73641=CARTESIAN_POINT ( 'NONE',  ( 6.732888861736110009, -58.30752899003807954, 3.750000000000001776 ) ) ;
#73650=TOROIDAL_SURFACE ( 'NONE', #70469, 0.5000000000000000000, 0.2500000000000000000 ) ;
#73653=CARTESIAN_POINT ( 'NONE',  ( 4.323020469704055735, -6.401304200527818011, 2.499999999999999556 ) ) ;
#73664=DIRECTION ( 'NONE',  ( 1.000000000000000000, -0.000000000000000000, -0.000000000000000000 ) ) ;
#73670=DIRECTION ( 'NONE',  ( 1.000000000000000000, 0.000000000000000000, 0.000000000000000000 ) ) ;
#73672=CARTESIAN_POINT ( 'NONE',  ( 8.879999999999991900, 69.99999999999998579, -6.396446609406726935 ) ) ;
#73674=DIRECTION ( 'NONE',  ( 0.000000000000000000, -0.000000000000000000, -1.000000000000000000 ) ) ;
#73697=DIRECTION ( 'NONE',  ( 0.000000000000000000, 0.000000000000000000, -1.000000000000000000 ) ) ;
#73701=ORIENTED_EDGE ( 'NONE', *, *, #27363, .T. ) ;
#73727=CARTESIAN_POINT ( 'NONE',  ( -13.42719148503447357, 90.83520141668820713, 7.724461209138537399 ) ) ;
#73728=VECTOR ( 'NONE', #97089, 1000.000000000000000 ) ;
#73729=EDGE_CURVE ( 'NONE', #52968, #8141, #92858, .T. ) ;
#73756=DIRECTION ( 'NONE',  ( -1.000000000000000000, 0.000000000000000000, 0.000000000000000000 ) ) ;
#73757=DIRECTION ( 'NONE',  ( 1.000000000000000000, 2.569960705150826877E-16, -0.000000000000000000 ) ) ;
#73761=ORIENTED_EDGE ( 'NONE', *, *, #63902, .F. ) ;
#73763=CIRCLE ( 'NONE', #75418, 2.999999999999997780 ) ;
#73770=CARTESIAN_POINT ( 'NONE',  ( 8.880000000000020322, 80.07179676972448590, -6.500000000000000888 ) ) ;
#73771=CARTESIAN_POINT ( 'NONE',  ( 0.000000000000000000, -97.00000000000000000, -2.750000000000000000 ) ) ;
#73773=DIRECTION ( 'NONE',  ( 0.000000000000000000, 0.000000000000000000, 1.000000000000000000 ) ) ;
#73775=DIRECTION ( 'NONE',  ( 1.000000000000000000, 0.000000000000000000, 0.000000000000000000 ) ) ;
#73793=LINE ( 'NONE', #74279, #12658 ) ;
#73798=EDGE_CURVE ( 'NONE', #38896, #538, #68150, .T. ) ;
#73802=VERTEX_POINT ( 'NONE', #89653 ) ;
#73827=EDGE_CURVE ( 'NONE', #97731, #2418, #20169, .T. ) ;
#73831=VERTEX_POINT ( 'NONE', #59145 ) ;
#73837=CARTESIAN_POINT ( 'NONE',  ( -13.80078213431832346, 90.89651191443149969, -7.751965754689354782 ) ) ;
#73846=ORIENTED_EDGE ( 'NONE', *, *, #13123, .F. ) ;
#73857=CARTESIAN_POINT ( 'NONE',  ( -9.098828036256710661, 88.10682954397121591, -5.081100641017341601 ) ) ;
#73868=CARTESIAN_POINT ( 'NONE',  ( 10.94841663143097144, -97.13876569039521769, 3.750000000000000000 ) ) ;
#73870=DIRECTION ( 'NONE',  ( 0.000000000000000000, 1.000000000000000000, -0.000000000000000000 ) ) ;
#73872=( BOUNDED_CURVE ( )  B_SPLINE_CURVE ( 3, ( #28175, #42691, #66163, #74153 ),
 .UNSPECIFIED., .F., .F. ) 
 B_SPLINE_CURVE_WITH_KNOTS ( ( 4, 4 ),
 ( 3.141592653589793116, 4.712388980384696779 ),
 .UNSPECIFIED. ) 
 CURVE ( )  GEOMETRIC_REPRESENTATION_ITEM ( )  RATIONAL_B_SPLINE_CURVE ( ( 1.000000000000000000, 0.8047378541243632721, 0.8047378541243632721, 1.000000000000000000 ) ) 
 REPRESENTATION_ITEM ( '' )  );
#73885=CARTESIAN_POINT ( 'NONE',  ( 4.657035931881701174, -8.268334176800257396, -3.999999999999194866 ) ) ;
#73891=DIRECTION ( 'NONE',  ( 0.000000000000000000, -3.035766082959409891E-14, 1.000000000000000000 ) ) ;
#73903=VECTOR ( 'NONE', #61076, 1000.000000000000000 ) ;
#73921=EDGE_CURVE ( 'NONE', #63872, #35357, #75139, .T. ) ;
#73947=AXIS2_PLACEMENT_3D ( 'NONE', #7949, #77901, #9413 ) ;
#73948=EDGE_CURVE ( 'NONE', #68711, #81557, #37652, .T. ) ;
#73950=ORIENTED_EDGE ( 'NONE', *, *, #41939, .T. ) ;
#73962=CARTESIAN_POINT ( 'NONE',  ( -7.072497013529895682, -84.40007040885102185, 2.750000000000805578 ) ) ;
#73970=VECTOR ( 'NONE', #65392, 1000.000000000000000 ) ;
#73974=CARTESIAN_POINT ( 'NONE',  ( -19.64999999999999858, 92.00000000000000000, 8.000000000000000000 ) ) ;
#73982=DIRECTION ( 'NONE',  ( 0.000000000000000000, -0.000000000000000000, -1.000000000000000000 ) ) ;
#73995=EDGE_LOOP ( 'NONE', ( #17266, #64441, #21441, #58002 ) ) ;
#74033=LINE ( 'NONE', #44028, #33041 ) ;
#74035=CARTESIAN_POINT ( 'NONE',  ( -3.889970118577497082, -8.287734203612162176, -3.750000000000000444 ) ) ;
#74052=FILL_AREA_STYLE ('',( #58559 ) ) ;
#74053=ORIENTED_EDGE ( 'NONE', *, *, #74963, .F. ) ;
#74075=CARTESIAN_POINT ( 'NONE',  ( 0.000000000000000000, 99.99999999999998579, 8.000000000000000000 ) ) ;
#74084=CARTESIAN_POINT ( 'NONE',  ( -4.261098476312686678, -13.83548126352581065, 3.750000000000000888 ) ) ;
#74087=ORIENTED_EDGE ( 'NONE', *, *, #95280, .T. ) ;
#74088=DIRECTION ( 'NONE',  ( -0.06975647374412544122, -0.9975640502598241977, 0.000000000000000000 ) ) ;
#74093=EDGE_CURVE ( 'NONE', #33481, #31750, #9605, .T. ) ;
#74094=DIRECTION ( 'NONE',  ( 0.000000000000000000, -1.000000000000000000, 0.000000000000000000 ) ) ;
#74105=( LENGTH_UNIT ( ) NAMED_UNIT ( * ) SI_UNIT ( .MILLI., .METRE. ) );
#74108=DIRECTION ( 'NONE',  ( 0.9961946980917461003, -0.08715574274765176821, 0.000000000000000000 ) ) ;
#74115=FACE_OUTER_BOUND ( 'NONE', #2986, .T. ) ;
#74116=CARTESIAN_POINT ( 'NONE',  ( 0.000000000000000000, -97.00000000000000000, 2.750000000000000000 ) ) ;
#74117=CARTESIAN_POINT ( 'NONE',  ( -8.124115902427741176, 75.04369783535875627, 2.900000000000000355 ) ) ;
#74145=ORIENTED_EDGE ( 'NONE', *, *, #30930, .F. ) ;
#74153=CARTESIAN_POINT ( 'NONE',  ( -16.60833333333333073, 99.74999999999998579, 8.000000000000000000 ) ) ;
#74159=FILL_AREA_STYLE_COLOUR ( '', #14050 ) ;
#74169=CARTESIAN_POINT ( 'NONE',  ( -15.00000000000000000, 83.99999999999998579, 3.750000000000000000 ) ) ;
#74176=( BOUNDED_CURVE ( )  B_SPLINE_CURVE ( 3, ( #44441, #98964, #52926, #74943 ),
 .UNSPECIFIED., .F., .T. ) 
 B_SPLINE_CURVE_WITH_KNOTS ( ( 4, 4 ),
 ( 0.000000000000000000, 1.570796326794896558 ),
 .UNSPECIFIED. ) 
 CURVE ( )  GEOMETRIC_REPRESENTATION_ITEM ( )  RATIONAL_B_SPLINE_CURVE ( ( 1.000000000000000000, 0.8047378541243649375, 0.8047378541243649375, 1.000000000000000000 ) ) 
 REPRESENTATION_ITEM ( '' )  );
#74179=TOROIDAL_SURFACE ( 'NONE', #5552, 0.5000000000000000000, 0.2500000000000000000 ) ;
#74190=( GEOMETRIC_REPRESENTATION_CONTEXT ( 3 ) GLOBAL_UNCERTAINTY_ASSIGNED_CONTEXT ( ( #13140 ) ) GLOBAL_UNIT_ASSIGNED_CONTEXT ( ( #47808, #2836, #34263 ) ) REPRESENTATION_CONTEXT ( 'NONE', 'WORKASPACE' ) );
#74193=CARTESIAN_POINT ( 'NONE',  ( -6.000000000000000000, 78.07179676972447169, 6.250000000000000000 ) ) ;
#74208=DIRECTION ( 'NONE',  ( 0.000000000000000000, -0.000000000000000000, -1.000000000000000000 ) ) ;
#74209=TOROIDAL_SURFACE ( 'NONE', #43886, 10.65000000000026326, 0.2500000000000000000 ) ;
#74221=LINE ( 'NONE', #53703, #53596 ) ;
#74224=DIRECTION ( 'NONE',  ( 1.000000000000000000, -0.000000000000000000, 0.000000000000000000 ) ) ;
#74226=CARTESIAN_POINT ( 'NONE',  ( -0.6999999999999957367, 99.99999999999998579, 8.000000000000000000 ) ) ;
#74240=DIRECTION ( 'NONE',  ( -1.000000000000000000, 0.000000000000000000, 0.000000000000000000 ) ) ;
#74242=AXIS2_PLACEMENT_3D ( 'NONE', #63267, #55283, #70801 ) ;
#74243=ADVANCED_FACE ( 'NONE', ( #661 ), #2630, .F. ) ;
#74249=DIRECTION ( 'NONE',  ( 1.000000000000000000, 2.107602052970794797E-16, -0.000000000000000000 ) ) ;
#74255=SURFACE_STYLE_USAGE ( .BOTH. , #20787 ) ;
#74257=DIRECTION ( 'NONE',  ( -1.000000000000000000, 0.000000000000000000, 0.000000000000000000 ) ) ;
#74263=EDGE_CURVE ( 'NONE', #69763, #86107, #91271, .T. ) ;
#74264=UNCERTAINTY_MEASURE_WITH_UNIT (LENGTH_MEASURE( 1.000000000000000082E-05 ), #4608, 'distance_accuracy_value', 'NONE');
#74271=EDGE_CURVE ( 'NONE', #29532, #37612, #88054, .T. ) ;
#74276=FILL_AREA_STYLE_COLOUR ( '', #15569 ) ;
#74279=CARTESIAN_POINT ( 'NONE',  ( 4.219999999999999751, 10.00000000000000000, -3.750000000000000000 ) ) ;
#74282=ORIENTED_EDGE ( 'NONE', *, *, #43035, .T. ) ;
#74288=CARTESIAN_POINT ( 'NONE',  ( -43.26219512195119421, 34.60975609756091842, -8.000000000000000000 ) ) ;
#74292=EDGE_CURVE ( 'NONE', #14873, #717, #59510, .T. ) ;
#74294=ORIENTED_EDGE ( 'NONE', *, *, #63879, .T. ) ;
#74298=ADVANCED_FACE ( 'NONE', ( #50062 ), #72272, .F. ) ;
#74306=PRESENTATION_STYLE_ASSIGNMENT (( #68804 ) ) ;
#74309=TOROIDAL_SURFACE ( 'NONE', #21664, 2.899999999999999467, 0.1000000000000000056 ) ;
#74326=FILL_AREA_STYLE ('',( #59328 ) ) ;
#74333=VECTOR ( 'NONE', #90222, 1000.000000000000000 ) ;
#74350=FACE_OUTER_BOUND ( 'NONE', #57626, .T. ) ;
#74355=CARTESIAN_POINT ( 'NONE',  ( 6.880000000000009663, 40.99999999999999289, 6.500000000000000888 ) ) ;
#74367=ORIENTED_EDGE ( 'NONE', *, *, #34774, .F. ) ;
#74368=DIRECTION ( 'NONE',  ( 0.000000000000000000, 0.000000000000000000, 1.000000000000000000 ) ) ;
#74369=CARTESIAN_POINT ( 'NONE',  ( -10.32525428031774339, -40.46312579907074536, -4.000000000000000000 ) ) ;
#74384=VECTOR ( 'NONE', #63398, 1000.000000000000000 ) ;
#74386=ADVANCED_FACE ( 'NONE', ( #95060 ), #72552, .T. ) ;
#74398=FACE_OUTER_BOUND ( 'NONE', #10960, .T. ) ;
#74405=EDGE_CURVE ( 'NONE', #85917, #55638, #71103, .T. ) ;
#74412=SURFACE_STYLE_USAGE ( .BOTH. , #57452 ) ;
#74421=ORIENTED_EDGE ( 'NONE', *, *, #75342, .F. ) ;
#74422=EDGE_CURVE ( 'NONE', #14972, #96670, #44934, .T. ) ;
#74433=AXIS2_PLACEMENT_3D ( 'NONE', #27123, #49620, #81117 ) ;
#74447=CARTESIAN_POINT ( 'NONE',  ( -6.732636091893170693, -88.11213685669366669, 2.500000000000000888 ) ) ;
#74451=CARTESIAN_POINT ( 'NONE',  ( 11.01504402775471014, -96.09667835293565474, 3.750000000000000000 ) ) ;
#74462=DIRECTION ( 'NONE',  ( 0.6246950475544237324, 0.7808688094430306093, 0.000000000000000000 ) ) ;
#74466=EDGE_CURVE ( 'NONE', #31523, #59916, #15242, .T. ) ;
#74487=MECHANICAL_DESIGN_GEOMETRIC_PRESENTATION_REPRESENTATION('',(#53621),#71295);
#74513=VECTOR ( 'NONE', #77159, 1000.000000000000000 ) ;
#74543=EDGE_CURVE ( 'NONE', #91314, #68676, #56164, .T. ) ;
#74577=CARTESIAN_POINT ( 'NONE',  ( 9.479672251262046601, -19.63639846206612560, 4.000000000000000888 ) ) ;
#74578=ORIENTED_EDGE ( 'NONE', *, *, #90990, .F. ) ;
#74586=EDGE_LOOP ( 'NONE', ( #26513, #32137, #1967 ) ) ;
#74588=CARTESIAN_POINT ( 'NONE',  ( -7.037762026445613550, -86.26090966542943761, 3.750000000000001332 ) ) ;
#74589=CARTESIAN_POINT ( 'NONE',  ( 9.779999999999990479, 18.00000000000000000, 0.000000000000000000 ) ) ;
#74593=VERTEX_POINT ( 'NONE', #81104 ) ;
#74599=ADVANCED_FACE ( 'NONE', ( #95114 ), #25666, .F. ) ;
#74603=FILL_AREA_STYLE_COLOUR ( '', #89022 ) ;
#74604=COLOUR_RGB ( '', 0.08235294, 0.09019608, 0.10196078) ;
#74641=MANIFOLD_SOLID_BREP ( 'Fillet9', #31460 ) ;
#74648=CARTESIAN_POINT ( 'NONE',  ( -4.250000000000000000, 37.00000000000000000, 4.000000000000000000 ) ) ;
#74659=CARTESIAN_POINT ( 'NONE',  ( -11.42361443008651634, -90.30744058743700009, 3.750000000000000000 ) ) ;
#74666=LINE ( 'NONE', #6176, #81116 ) ;
#74673=VERTEX_POINT ( 'NONE', #98105 ) ;
#74685=VERTEX_POINT ( 'NONE', #74589 ) ;
#74689=VERTEX_POINT ( 'NONE', #81590 ) ;
#74700=LINE ( 'NONE', #53672, #39304 ) ;
#74701=ORIENTED_EDGE ( 'NONE', *, *, #48492, .F. ) ;
#74703=LINE ( 'NONE', #59196, #1993 ) ;
#74704=LINE ( 'NONE', #6214, #18012 ) ;
#74705=FACE_OUTER_BOUND ( 'NONE', #61247, .T. ) ;
#74728=FACE_OUTER_BOUND ( 'NONE', #97943, .T. ) ;
#74730=CARTESIAN_POINT ( 'NONE',  ( 12.30000000000000249, 99.99999999999998579, 8.000000000000000000 ) ) ;
#74739=DIRECTION ( 'NONE',  ( 0.000000000000000000, 0.000000000000000000, 1.000000000000000000 ) ) ;
#74750=CARTESIAN_POINT ( 'NONE',  ( 6.432108699068923130, -88.20011490510430008, 2.750000000000000000 ) ) ;
#74751=LINE ( 'NONE', #51262, #39112 ) ;
#74759=CARTESIAN_POINT ( 'NONE',  ( 9.479665769801981057, -19.63627307883762185, -4.000000000000000000 ) ) ;
#74765=DIRECTION ( 'NONE',  ( 0.000000000000000000, 0.000000000000000000, -1.000000000000000000 ) ) ;
#74769=FACE_OUTER_BOUND ( 'NONE', #46875, .T. ) ;
#74773=MECHANICAL_DESIGN_GEOMETRIC_PRESENTATION_REPRESENTATION('',(#34794),#15697);
#74786=CARTESIAN_POINT ( 'NONE',  ( 4.864290147396342689, -17.52197929138388588, -2.500000000000000000 ) ) ;
#74789=CARTESIAN_POINT ( 'NONE',  ( -3.628626192037550435, -3.642031182890759666, 3.999999999999193090 ) ) ;
#74797=EDGE_CURVE ( 'NONE', #76544, #46091, #43364, .T. ) ;
#74800=EDGE_LOOP ( 'NONE', ( #38450, #37704, #94608, #7203 ) ) ;
#74803=ORIENTED_EDGE ( 'NONE', *, *, #92438, .T. ) ;
#74804=EDGE_CURVE ( 'NONE', #28677, #35851, #30066, .T. ) ;
#74806=VERTEX_POINT ( 'NONE', #97129 ) ;
#74813=AXIS2_PLACEMENT_3D ( 'NONE', #39880, #1905, #75904 ) ;
#74822=VECTOR ( 'NONE', #87428, 1000.000000000000000 ) ;
#74829=DIRECTION ( 'NONE',  ( 1.000000000000000000, 0.000000000000000000, 0.000000000000000000 ) ) ;
#74835=ORIENTED_EDGE ( 'NONE', *, *, #4128, .T. ) ;
#74838=FACE_OUTER_BOUND ( 'NONE', #89021, .T. ) ;
#74842=CARTESIAN_POINT ( 'NONE',  ( 5.113979357139876392, -17.50950876244384702, -2.500000000001608491 ) ) ;
#74847=CARTESIAN_POINT ( 'NONE',  ( 3.969999999999999751, 36.75000000000000000, 2.500000000000000000 ) ) ;
#74849=CARTESIAN_POINT ( 'NONE',  ( -12.16982443903231292, 90.48687232357865184, -7.214476785723133112 ) ) ;
#74853=CARTESIAN_POINT ( 'NONE',  ( 3.969999999999999751, 36.75000000000000000, 2.750000000000000000 ) ) ;
#74858=SURFACE_STYLE_FILL_AREA ( #11899 ) ;
#74860=LINE ( 'NONE', #82856, #33142 ) ;
#74867=DIRECTION ( 'NONE',  ( 0.02970531260815257105, -0.9995586998285053149, 0.000000000000000000 ) ) ;
#74874=ORIENTED_EDGE ( 'NONE', *, *, #43686, .T. ) ;
#74875=FACE_OUTER_BOUND ( 'NONE', #19598, .T. ) ;
#74880=LINE ( 'NONE', #42910, #76559 ) ;
#74881=AXIS2_PLACEMENT_3D ( 'NONE', #95165, #42668, #18698 ) ;
#74902=COLOUR_RGB ( '', 0.72549020, 0.75294118, 0.79215686) ;
#74907=MECHANICAL_DESIGN_GEOMETRIC_PRESENTATION_REPRESENTATION('',(#46164),#89252);
#74918=( NAMED_UNIT ( * ) SI_UNIT ( $, .STERADIAN. ) SOLID_ANGLE_UNIT ( ) );
#74919=DIRECTION ( 'NONE',  ( 0.000000000000000000, 0.000000000000000000, -1.000000000000000000 ) ) ;
#74933=DIRECTION ( 'NONE',  ( -0.08715574274765139351, -0.9961946980917461003, 0.000000000000000000 ) ) ;
#74943=CARTESIAN_POINT ( 'NONE',  ( 9.779999999999988702, 27.00436609429084811, 3.000000000000000000 ) ) ;
#74950=CARTESIAN_POINT ( 'NONE',  ( -7.079903288618116797, -69.52484394646381816, 2.750000000000000000 ) ) ;
#74954=CARTESIAN_POINT ( 'NONE',  ( 10.89309004150372751, -97.65096242295280149, 3.749999999996625810 ) ) ;
#74963=EDGE_CURVE ( 'NONE', #67464, #44301, #84075, .T. ) ;
#74969=CARTESIAN_POINT ( 'NONE',  ( -13.68546037613094057, 90.96609652458319317, -7.941826699654800592 ) ) ;
#74971=CARTESIAN_POINT ( 'NONE',  ( 8.629999999999995453, 41.24999999999999289, -6.250000000000000000 ) ) ;
#74979=DIRECTION ( 'NONE',  ( 1.257402221000611116E-16, -1.000000000000000000, 0.000000000000000000 ) ) ;
#74983=( BOUNDED_SURFACE ( )  B_SPLINE_SURFACE ( 3, 2, ( 
 ( #7842, #16321, #98863 ),
 ( #38339, #22352, #31302 ),
 ( #53320, #44825, #84336 ),
 ( #75331, #6844, #68834 ),
 ( #69322, #67849, #52827 ),
 ( #76810, #98367, #45839 ),
 ( #82835, #83334, #92310 ),
 ( #45331, #75830, #46323 ),
 ( #365, #74842, #30317 ),
 ( #30813, #7351, #61803 ),
 ( #15354, #29823, #15838 ),
 ( #23342, #61312, #37852 ),
 ( #84815, #53824, #6343 ),
 ( #68342, #91318, #8325 ),
 ( #60819, #22846, #38829 ),
 ( #843, #60333, #36854 ),
 ( #67345, #97871, #29331 ),
 ( #90322, #21860, #52340 ) ),
 .UNSPECIFIED., .F., .F., .F. ) 
 B_SPLINE_SURFACE_WITH_KNOTS ( ( 4, 2, 2, 2, 2, 2, 2, 2, 4 ),
 ( 3, 3 ),
 ( 0.000000000000000000, 0.002783459421176835875, 0.005566918842353671751, 0.01113383768470734350, 0.02226767536941468700, 0.04453535073882937401, 0.06680302610824406795, 0.07793686379295140798, 0.08907070147765874801 ),
 ( 0.000000000000000000, 1.000000000000000000 ),
 .UNSPECIFIED. ) 
 GEOMETRIC_REPRESENTATION_ITEM ( )  RATIONAL_B_SPLINE_SURFACE ( (
 ( 1.000000000000000000, 0.7071067811865482389, 1.000000000000000000),
 ( 1.000000000000000000, 0.7071067811865482389, 1.000000000000000000),
 ( 1.000000000000000000, 0.7071067811865482389, 1.000000000000000000),
 ( 1.000000000000000000, 0.7071067811865482389, 1.000000000000000000),
 ( 1.000000000000000000, 0.7071067811865482389, 1.000000000000000000),
 ( 1.000000000000000000, 0.7071067811865482389, 1.000000000000000000),
 ( 1.000000000000000000, 0.7071067811865469066, 1.000000000000000000),
 ( 1.000000000000000000, 0.7071067811865469066, 1.000000000000000000),
 ( 1.000000000000000000, 0.7071067811865471286, 1.000000000000000000),
 ( 1.000000000000000000, 0.7071067811865471286, 1.000000000000000000),
 ( 1.000000000000000000, 0.7071067811865456854, 1.000000000000000000),
 ( 1.000000000000000000, 0.7071067811865456854, 1.000000000000000000),
 ( 1.000000000000000000, 0.7071067811865482389, 1.000000000000000000),
 ( 1.000000000000000000, 0.7071067811865482389, 1.000000000000000000),
 ( 1.000000000000000000, 0.7071067811865493491, 1.000000000000000000),
 ( 1.000000000000000000, 0.7071067811865493491, 1.000000000000000000),
 ( 1.000000000000000000, 0.7071067811865482389, 1.000000000000000000),
 ( 1.000000000000000000, 0.7071067811865482389, 1.000000000000000000) ) ) 
 REPRESENTATION_ITEM ( '' )  SURFACE ( )  );
#74997=AXIS2_PLACEMENT_3D ( 'NONE', #96921, #20907, #73891 ) ;
#75021=DIRECTION ( 'NONE',  ( 0.000000000000000000, 0.000000000000000000, 1.000000000000000000 ) ) ;
#75025=CARTESIAN_POINT ( 'NONE',  ( -3.750000000000000000, 10.25000000000000000, -2.500000000000000000 ) ) ;
#75027=DIRECTION ( 'NONE',  ( -0.000000000000000000, -0.000000000000000000, -1.000000000000000000 ) ) ;
#75028=CARTESIAN_POINT ( 'NONE',  ( -4.537879770859267303, -17.56524742835268782, -3.749999999998386180 ) ) ;
#75030=ORIENTED_EDGE ( 'NONE', *, *, #15576, .F. ) ;
#75035=( LENGTH_UNIT ( ) NAMED_UNIT ( * ) SI_UNIT ( .MILLI., .METRE. ) );
#75046=DIRECTION ( 'NONE',  ( 0.06975647374412452528, 0.9975640502598243087, 0.000000000000000000 ) ) ;
#75064=ORIENTED_EDGE ( 'NONE', *, *, #35785, .T. ) ;
#75075=ORIENTED_EDGE ( 'NONE', *, *, #84249, .T. ) ;
#75082=SURFACE_STYLE_FILL_AREA ( #13598 ) ;
#75104=SURFACE_STYLE_USAGE ( .BOTH. , #28121 ) ;
#75123=UNCERTAINTY_MEASURE_WITH_UNIT (LENGTH_MEASURE( 1.000000000000000082E-05 ), #2327, 'distance_accuracy_value', 'NONE');
#75126=VECTOR ( 'NONE', #1488, 1000.000000000000114 ) ;
#75130=CIRCLE ( 'NONE', #63981, 0.2500000000000002220 ) ;
#75139=LINE ( 'NONE', #97675, #83285 ) ;
#75143=DIRECTION ( 'NONE',  ( -0.000000000000000000, 0.000000000000000000, 1.000000000000000000 ) ) ;
#75150=CARTESIAN_POINT ( 'NONE',  ( -8.107943641816854452, -3.126452786863499256, 3.750000000000000000 ) ) ;
#75169=DIRECTION ( 'NONE',  ( 0.000000000000000000, -1.000000000000000000, 0.000000000000000000 ) ) ;
#75172=CIRCLE ( 'NONE', #11283, 0.2500000000000002220 ) ;
#75197=CARTESIAN_POINT ( 'NONE',  ( -7.750000000000000000, 41.24999999999999289, -6.250000000000000000 ) ) ;
#75198=AXIS2_PLACEMENT_3D ( 'NONE', #34422, #3465, #94934 ) ;
#75215=ORIENTED_EDGE ( 'NONE', *, *, #51184, .T. ) ;
#75220=SURFACE_STYLE_USAGE ( .BOTH. , #84224 ) ;
#75224=CARTESIAN_POINT ( 'NONE',  ( 0.000000000000000000, 80.32179676972448590, 4.000000000000000000 ) ) ;
#75227=DIRECTION ( 'NONE',  ( 1.049065152435176504E-16, -1.000000000000000000, 0.000000000000000000 ) ) ;
#75231=DIRECTION ( 'NONE',  ( -1.000000000000000000, 0.000000000000000000, 0.000000000000000000 ) ) ;
#75234=COLOUR_RGB ( '', 0.31764706, 0.68627451, 0.89019608) ;
#75238=AXIS2_PLACEMENT_3D ( 'NONE', #84476, #55451, #1482 ) ;
#75239=ORIENTED_EDGE ( 'NONE', *, *, #18543, .F. ) ;
#75243=CARTESIAN_POINT ( 'NONE',  ( 6.880000000000009663, 40.74999999999999289, 4.000000000000000000 ) ) ;
#75245=CARTESIAN_POINT ( 'NONE',  ( 8.629999999999995453, 41.24999999999999289, -6.250000000000000000 ) ) ;
#75249=ORIENTED_EDGE ( 'NONE', *, *, #6952, .T. ) ;
#75251=CARTESIAN_POINT ( 'NONE',  ( 10.76563361875039782, -96.07941716639480489, -4.000000000000000000 ) ) ;
#75256=( LENGTH_UNIT ( ) NAMED_UNIT ( * ) SI_UNIT ( .MILLI., .METRE. ) );
#75261=DIRECTION ( 'NONE',  ( -1.257402221000611116E-16, 1.000000000000000000, 0.000000000000000000 ) ) ;
#75263=AXIS2_PLACEMENT_3D ( 'NONE', #28719, #89713, #29208 ) ;
#75267=EDGE_LOOP ( 'NONE', ( #94632, #87447, #82551, #80304 ) ) ;
#75269=FACE_OUTER_BOUND ( 'NONE', #36184, .T. ) ;
#75278=COLOUR_RGB ( '', 0.31764706, 0.68627451, 0.89019608) ;
#75279=CARTESIAN_POINT ( 'NONE',  ( 6.507517414235627129, -58.30789062356495833, -2.499999999999999112 ) ) ;
#75284=AXIS2_PLACEMENT_3D ( 'NONE', #25608, #95569, #12061 ) ;
#75292=ORIENTED_EDGE ( 'NONE', *, *, #90022, .F. ) ;
#75297=ORIENTED_EDGE ( 'NONE', *, *, #96550, .T. ) ;
#75300=DIRECTION ( 'NONE',  ( -0.000000000000000000, 0.000000000000000000, 1.000000000000000000 ) ) ;
#75307=EDGE_CURVE ( 'NONE', #66682, #14813, #64123, .T. ) ;
#75319=CARTESIAN_POINT ( 'NONE',  ( 6.349999999999995204, -97.00000000000000000, 3.750000000000000000 ) ) ;
#75328=CIRCLE ( 'NONE', #38589, 2.750000000000002665 ) ;
#75331=CARTESIAN_POINT ( 'NONE',  ( 4.191189844333915282, -2.692444605285015946, -2.500000000000000888 ) ) ;
#75334=LINE ( 'NONE', #37856, #13660 ) ;
#75336=CARTESIAN_POINT ( 'NONE',  ( 6.579634127946608402, -87.99828267815712479, 2.500000000000000000 ) ) ;
#75342=EDGE_CURVE ( 'NONE', #24454, #38399, #14707, .T. ) ;
#75346=EDGE_LOOP ( 'NONE', ( #31324, #66797, #71026, #94578 ) ) ;
#75356=B_SPLINE_SURFACE_WITH_KNOTS ( 'NONE', 3, 1, ( 
 ( #41660, #3655 ),
 ( #34612, #87623 ),
 ( #95630, #42625 ),
 ( #59094, #30073 ),
 ( #28104, #82095 ) ),
 .UNSPECIFIED., .F., .F., .F.,
 ( 4, 1, 4 ),
 ( 2, 2 ),
 ( 0.000000000000000000, 0.4657625508283478322, 1.000000000000000000 ),
 ( 0.000000000000000000, 1.000000000000000000 ),
 .UNSPECIFIED. ) ;
#75359=CARTESIAN_POINT ( 'NONE',  ( 6.829574850505126804, -88.00372650098204019, 2.750000000000002665 ) ) ;
#75365=FACE_OUTER_BOUND ( 'NONE', #38707, .T. ) ;
#75371=CARTESIAN_POINT ( 'NONE',  ( -13.69999999999999751, 99.99999999999998579, 8.000000000000000000 ) ) ;
#75404=CARTESIAN_POINT ( 'NONE',  ( 4.920853330076631060, -13.83152733636334020, 4.000000000001609379 ) ) ;
#75405=DIRECTION ( 'NONE',  ( -0.000000000000000000, 0.000000000000000000, 1.000000000000000000 ) ) ;
#75411=( GEOMETRIC_REPRESENTATION_CONTEXT ( 3 ) GLOBAL_UNCERTAINTY_ASSIGNED_CONTEXT ( ( #63188 ) ) GLOBAL_UNIT_ASSIGNED_CONTEXT ( ( #49725, #34724, #94749 ) ) REPRESENTATION_CONTEXT ( 'NONE', 'WORKASPACE' ) );
#75418=AXIS2_PLACEMENT_3D ( 'NONE', #25138, #3119, #87087 ) ;
#75430=AXIS2_PLACEMENT_3D ( 'NONE', #42679, #41227, #65660 ) ;
#75448=CARTESIAN_POINT ( 'NONE',  ( 6.284496703633148051, -36.06254290988034228, -4.000000000000000888 ) ) ;
#75456=UNCERTAINTY_MEASURE_WITH_UNIT (LENGTH_MEASURE( 1.000000000000000082E-05 ), #47065, 'distance_accuracy_value', 'NONE');
#75473=EDGE_CURVE ( 'NONE', #32093, #51986, #62632, .T. ) ;
#75495=CIRCLE ( 'NONE', #97853, 0.2499999999999995559 ) ;
#75510=ORIENTED_EDGE ( 'NONE', *, *, #11287, .T. ) ;
#75521=TOROIDAL_SURFACE ( 'NONE', #78745, 7.250000000000002665, 0.2500000000000000000 ) ;
#75522=EDGE_CURVE ( 'NONE', #31285, #44437, #96207, .T. ) ;
#75524=CARTESIAN_POINT ( 'NONE',  ( -7.366168427725257040, -80.69295184796105502, -4.000000000000000000 ) ) ;
#75525=ORIENTED_EDGE ( 'NONE', *, *, #45198, .T. ) ;
#75541=DIRECTION ( 'NONE',  ( 1.000000000000000000, -1.303078667400386302E-15, 0.000000000000000000 ) ) ;
#75544=ORIENTED_EDGE ( 'NONE', *, *, #97379, .T. ) ;
#75546=ORIENTED_EDGE ( 'NONE', *, *, #25889, .F. ) ;
#75558=ORIENTED_EDGE ( 'NONE', *, *, #37407, .T. ) ;
#75561=VERTEX_POINT ( 'NONE', #77941 ) ;
#75562=EDGE_CURVE ( 'NONE', #75561, #87452, #40315, .T. ) ;
#75564=VERTEX_POINT ( 'NONE', #15499 ) ;
#75570=CARTESIAN_POINT ( 'NONE',  ( -4.000000000000000000, 10.25000000000000000, 2.500000000000000000 ) ) ;
#75571=CARTESIAN_POINT ( 'NONE',  ( 3.969999999999999751, 36.75000000000000000, 2.750000000000000000 ) ) ;
#75572=CARTESIAN_POINT ( 'NONE',  ( 11.10646695662389760, -65.08356741891232389, 4.000000000000000000 ) ) ;
#75573=VERTEX_POINT ( 'NONE', #53464 ) ;
#75575=ORIENTED_EDGE ( 'NONE', *, *, #63202, .F. ) ;
#75577=CARTESIAN_POINT ( 'NONE',  ( -3.750000000000000000, 10.25000000000000000, -3.750000000000000000 ) ) ;
#75579=ORIENTED_EDGE ( 'NONE', *, *, #11408, .T. ) ;
#75588=CARTESIAN_POINT ( 'NONE',  ( -7.750000000000000000, 80.07179676972448590, -4.250000000000000000 ) ) ;
#75610=DIRECTION ( 'NONE',  ( 0.08715574274765129636, 0.9961946980917462113, 0.000000000000000000 ) ) ;
#75619=AXIS2_PLACEMENT_3D ( 'NONE', #22387, #82876, #37884 ) ;
#75620=CIRCLE ( 'NONE', #37317, 0.2500000000000002220 ) ;
#75627=SURFACE_STYLE_FILL_AREA ( #53612 ) ;
#75637=DIRECTION ( 'NONE',  ( -0.000000000000000000, -0.000000000000000000, -1.000000000000000000 ) ) ;
#75647=CARTESIAN_POINT ( 'NONE',  ( -9.823916613453683055, -32.16564667760975027, 4.000000000000000000 ) ) ;
#75652=ADVANCED_FACE ( 'NONE', ( #30958 ), #38973, .T. ) ;
#75658=ORIENTED_EDGE ( 'NONE', *, *, #12112, .T. ) ;
#75661=SURFACE_STYLE_USAGE ( .BOTH. , #45157 ) ;
#75672=ORIENTED_EDGE ( 'NONE', *, *, #84873, .T. ) ;
#75680=CARTESIAN_POINT ( 'NONE',  ( 4.879999999999991900, 76.07179676972444327, -6.500000000000000888 ) ) ;
#75685=DIRECTION ( 'NONE',  ( -1.000000000000000000, -0.000000000000000000, -0.000000000000000000 ) ) ;
#75690=( LENGTH_UNIT ( ) NAMED_UNIT ( * ) SI_UNIT ( .MILLI., .METRE. ) );
#75697=DIRECTION ( 'NONE',  ( -0.000000000000000000, 0.000000000000000000, 1.000000000000000000 ) ) ;
#75711=DIRECTION ( 'NONE',  ( 1.000000000000000000, 0.000000000000000000, 0.000000000000000000 ) ) ;
#75718=CYLINDRICAL_SURFACE ( 'NONE', #13704, 1.249999999999987121 ) ;
#75719=DIRECTION ( 'NONE',  ( 1.000000000000000000, 0.000000000000000000, 0.000000000000000000 ) ) ;
#75723=ADVANCED_FACE ( 'NONE', ( #25932 ), #41211, .F. ) ;
#75729=FACE_OUTER_BOUND ( 'NONE', #38172, .T. ) ;
#75742=EDGE_LOOP ( 'NONE', ( #77890, #17617, #74367, #55879 ) ) ;
#75744=CARTESIAN_POINT ( 'NONE',  ( 10.89310702003767162, -97.65080520972955469, -4.000000000001574740 ) ) ;
#75754=DIRECTION ( 'NONE',  ( -1.000000000000000000, -1.257402221000612102E-16, 0.000000000000000000 ) ) ;
#75758=ORIENTED_EDGE ( 'NONE', *, *, #59560, .F. ) ;
#75771=FACE_OUTER_BOUND ( 'NONE', #83926, .T. ) ;
#75773=VECTOR ( 'NONE', #77078, 1000.000000000000114 ) ;
#75775=( NAMED_UNIT ( * ) PLANE_ANGLE_UNIT ( ) SI_UNIT ( $, .RADIAN. ) );
#75787=EDGE_CURVE ( 'NONE', #53779, #22610, #94546, .T. ) ;
#75788=ORIENTED_EDGE ( 'NONE', *, *, #24777, .T. ) ;
#75790=CARTESIAN_POINT ( 'NONE',  ( -6.000000000000009770, 40.99999999999999289, -6.250000000000000000 ) ) ;
#75792=EDGE_CURVE ( 'NONE', #22141, #93500, #27521, .T. ) ;
#75795=CARTESIAN_POINT ( 'NONE',  ( 14.35000000000000142, 98.49999999999998579, 8.000000000000000000 ) ) ;
#75797=SURFACE_STYLE_USAGE ( .BOTH. , #98334 ) ;
#75798=SURFACE_STYLE_FILL_AREA ( #38308 ) ;
#75803=VERTEX_POINT ( 'NONE', #35878 ) ;
#75813=CARTESIAN_POINT ( 'NONE',  ( -7.750000000000000000, 1.019547802438458550, 4.000000000000000000 ) ) ;
#75825=ORIENTED_EDGE ( 'NONE', *, *, #38119, .F. ) ;
#75830=CARTESIAN_POINT ( 'NONE',  ( 4.919406150734204175, -13.80316667495554661, -2.499999999999999112 ) ) ;
#75850=CARTESIAN_POINT ( 'NONE',  ( -9.206646936887572963, -19.70874149522336793, -3.750000000000000000 ) ) ;
#75854=ORIENTED_EDGE ( 'NONE', *, *, #93597, .T. ) ;
#75867=CARTESIAN_POINT ( 'NONE',  ( -3.750000000000000000, 37.00000000000000000, 2.750000000000000000 ) ) ;
#75873=FILL_AREA_STYLE_COLOUR ( '', #35213 ) ;
#75877=DIRECTION ( 'NONE',  ( 0.000000000000000000, 0.000000000000000000, 1.000000000000000000 ) ) ;
#75884=DIRECTION ( 'NONE',  ( -0.000000000000000000, 0.000000000000000000, 1.000000000000000000 ) ) ;
#75903=CARTESIAN_POINT ( 'NONE',  ( 5.680373671027947324, -28.65980262291034819, 3.749999999996780353 ) ) ;
#75904=DIRECTION ( 'NONE',  ( -0.08715574274765112983, -0.9961946980917461003, 0.000000000000000000 ) ) ;
#75926=VERTEX_POINT ( 'NONE', #391 ) ;
#75931=B_SPLINE_CURVE_WITH_KNOTS ( 'NONE', 3,
 ( #70680, #62167, #9185, #69688, #23721, #18167, #70187, #730, #31184, #39201, #17196, #1704, #40673, #92196, #1222, #33150, #62662, #9678 ),
 .UNSPECIFIED., .F., .F.,
 ( 4, 2, 2, 2, 2, 2, 2, 2, 4 ),
 ( 0.000000000000000000, 0.01113508862748988255, 0.02227017725497976511, 0.04454035450995957185, 0.06681053176493938206, 0.07794562039242927676, 0.08351316470617423104, 0.08629693686304670819, 0.08908070901991918533 ),
 .UNSPECIFIED. ) ;
#75932=ORIENTED_EDGE ( 'NONE', *, *, #77125, .T. ) ;
#75939=DIRECTION ( 'NONE',  ( 0.000000000000000000, 0.000000000000000000, 1.000000000000000000 ) ) ;
#75951=CARTESIAN_POINT ( 'NONE',  ( -12.23643000159001382, 90.44368800334291336, 7.046674173435446775 ) ) ;
#75964=EDGE_CURVE ( 'NONE', #5021, #39466, #5206, .T. ) ;
#75975=CIRCLE ( 'NONE', #85546, 0.2500000000000002220 ) ;
#76000=DIRECTION ( 'NONE',  ( -1.000000000000000000, 0.000000000000000000, 0.000000000000000000 ) ) ;
#76018=CARTESIAN_POINT ( 'NONE',  ( -6.982525766850296911, -88.11956318484570261, -3.750000000000000000 ) ) ;
#76049=ORIENTED_EDGE ( 'NONE', *, *, #76248, .T. ) ;
#76052=ORIENTED_EDGE ( 'NONE', *, *, #27469, .F. ) ;
#76054=EDGE_CURVE ( 'NONE', #70343, #67870, #30340, .T. ) ;
#76061=CARTESIAN_POINT ( 'NONE',  ( 8.959592931132405624, -9.312622102011351544, 4.000000000000000888 ) ) ;
#76064=ORIENTED_EDGE ( 'NONE', *, *, #87825, .T. ) ;
#76071=CARTESIAN_POINT ( 'NONE',  ( 14.99999999999997868, 80.07179676972448590, 6.250000000000000000 ) ) ;
#76073=ORIENTED_EDGE ( 'NONE', *, *, #61400, .T. ) ;
#76084=FACE_OUTER_BOUND ( 'NONE', #63459, .T. ) ;
#76094=CARTESIAN_POINT ( 'NONE',  ( -7.045329894599615450, -66.66420243593404393, -3.750000000000000000 ) ) ;
#76102=SURFACE_SIDE_STYLE ('',( #46108 ) ) ;
#76112=CARTESIAN_POINT ( 'NONE',  ( -9.000000000000001776, 80.99999999999994316, 1.249999999999987121 ) ) ;
#76114=UNCERTAINTY_MEASURE_WITH_UNIT (LENGTH_MEASURE( 1.000000000000000082E-05 ), #94242, 'distance_accuracy_value', 'NONE');
#76131=VECTOR ( 'NONE', #23960, 1000.000000000000000 ) ;
#76134=ORIENTED_EDGE ( 'NONE', *, *, #75473, .T. ) ;
#76135=EDGE_LOOP ( 'NONE', ( #68093, #53798, #39888 ) ) ;
#76142=CARTESIAN_POINT ( 'NONE',  ( -8.897278993253172175, -15.56326597357423758, 3.750000000000000000 ) ) ;
#76156=( LENGTH_UNIT ( ) NAMED_UNIT ( * ) SI_UNIT ( .MILLI., .METRE. ) );
#76157=ORIENTED_EDGE ( 'NONE', *, *, #13905, .F. ) ;
#76158=CARTESIAN_POINT ( 'NONE',  ( 0.4400000000000020006, 1.019547802438468986, 4.000000000000000000 ) ) ;
#76163=DIRECTION ( 'NONE',  ( -0.9961946980917453232, 0.08715574274766037244, 0.000000000000000000 ) ) ;
#76164=EDGE_CURVE ( 'NONE', #80552, #81788, #75495, .T. ) ;
#76168=VECTOR ( 'NONE', #55983, 1000.000000000000000 ) ;
#76169=ORIENTED_EDGE ( 'NONE', *, *, #31605, .F. ) ;
#76185=FILL_AREA_STYLE ('',( #77161 ) ) ;
#76193=DIRECTION ( 'NONE',  ( 0.000000000000000000, -0.000000000000000000, -1.000000000000000000 ) ) ;
#76203=EDGE_CURVE ( 'NONE', #19964, #19346, #85324, .T. ) ;
#76208=CIRCLE ( 'NONE', #96995, 0.2500000000000002220 ) ;
#76215=ADVANCED_FACE ( 'NONE', ( #7866 ), #868, .F. ) ;
#76223=SURFACE_SIDE_STYLE ('',( #45721 ) ) ;
#76228=CARTESIAN_POINT ( 'NONE',  ( -6.349999999999995204, -97.00000000000000000, -3.750000000000000000 ) ) ;
#76240=DIRECTION ( 'NONE',  ( 0.000000000000000000, 0.000000000000000000, -1.000000000000000000 ) ) ;
#76248=EDGE_CURVE ( 'NONE', #2391, #23479, #59502, .T. ) ;
#76249=CARTESIAN_POINT ( 'NONE',  ( 11.19532855852642328, -77.48518070173305716, -4.000000000000000000 ) ) ;
#76250=LINE ( 'NONE', #5782, #33127 ) ;
#76252=DIRECTION ( 'NONE',  ( -0.000000000000000000, -1.000000000000000000, -0.000000000000000000 ) ) ;
#76259=ORIENTED_EDGE ( 'NONE', *, *, #427, .F. ) ;
#76271=CARTESIAN_POINT ( 'NONE',  ( 11.24699797944280100, 54.09857164847241506, 0.000000000000000000 ) ) ;
#76275=CARTESIAN_POINT ( 'NONE',  ( -3.500000001642929792, 0.08393865083513252223, 4.000000000000000000 ) ) ;
#76288=ORIENTED_EDGE ( 'NONE', *, *, #18061, .T. ) ;
#76299=EDGE_CURVE ( 'NONE', #15068, #72111, #71799, .T. ) ;
#76307=DIRECTION ( 'NONE',  ( -0.000000000000000000, -0.000000000000000000, 1.000000000000000000 ) ) ;
#76321=CIRCLE ( 'NONE', #98770, 10.00000000000000178 ) ;
#76328=CARTESIAN_POINT ( 'NONE',  ( -8.124115902427741176, 75.04369783535875627, -2.900000000000000355 ) ) ;
#76334=DIRECTION ( 'NONE',  ( 1.000000000000000000, 0.000000000000000000, 0.000000000000000000 ) ) ;
#76339=AXIS2_PLACEMENT_3D ( 'NONE', #68767, #298, #46260 ) ;
#76341=VECTOR ( 'NONE', #87692, 1000.000000000000000 ) ;
#76342=CARTESIAN_POINT ( 'NONE',  ( -8.000000002515021080, -0.01655697268385602355, -4.000000000000000000 ) ) ;
#76359=ORIENTED_EDGE ( 'NONE', *, *, #39383, .T. ) ;
#76360=( NAMED_UNIT ( * ) PLANE_ANGLE_UNIT ( ) SI_UNIT ( $, .RADIAN. ) );
#76361=EDGE_CURVE ( 'NONE', #35180, #59059, #17818, .T. ) ;
#76367=FACE_OUTER_BOUND ( 'NONE', #40897, .T. ) ;
#76388=VECTOR ( 'NONE', #27772, 1000.000000000000000 ) ;
#76396=ORIENTED_EDGE ( 'NONE', *, *, #47195, .F. ) ;
#76398=CARTESIAN_POINT ( 'NONE',  ( 4.657035931814768048, -8.268334176803392666, 3.749999999999597211 ) ) ;
#76403=CARTESIAN_POINT ( 'NONE',  ( -7.371420888394235149, -73.25401859617248590, -4.000000000000000888 ) ) ;
#76406=EDGE_LOOP ( 'NONE', ( #58681, #19212, #20396, #94502, #62032 ) ) ;
#76409=AXIS2_PLACEMENT_3D ( 'NONE', #43104, #14100, #97619 ) ;
#76419=STYLED_ITEM ( 'NONE', ( #92019 ), #70810 ) ;
#76426=ORIENTED_EDGE ( 'NONE', *, *, #72570, .T. ) ;
#76437=DIRECTION ( 'NONE',  ( 0.000000000000000000, 0.000000000000000000, -1.000000000000000000 ) ) ;
#76451=DIRECTION ( 'NONE',  ( 0.9995586998285053149, 0.02970531260815256758, 0.000000000000000000 ) ) ;
#76455=CARTESIAN_POINT ( 'NONE',  ( 4.864310448992819502, -17.52237222647785941, 2.500000000000000000 ) ) ;
#76476=CARTESIAN_POINT ( 'NONE',  ( 9.879999999999988347, 26.99999999999999645, -2.900000000000000799 ) ) ;
#76485=DIRECTION ( 'NONE',  ( 0.000000000000000000, 0.000000000000000000, 1.000000000000000000 ) ) ;
#76496=CARTESIAN_POINT ( 'NONE',  ( 8.630000000000000782, 1.019547802438458550, -3.750000000000000000 ) ) ;
#76500=DIRECTION ( 'NONE',  ( -0.06975647374412544122, -0.9975640502598241977, -0.000000000000000000 ) ) ;
#76508=DIRECTION ( 'NONE',  ( -0.000000000000000000, -0.000000000000000000, -1.000000000000000000 ) ) ;
#76512=ORIENTED_EDGE ( 'NONE', *, *, #21963, .T. ) ;
#76530=VERTEX_POINT ( 'NONE', #10808 ) ;
#76544=VERTEX_POINT ( 'NONE', #70832 ) ;
#76552=EDGE_LOOP ( 'NONE', ( #17378, #33423, #95078, #44644 ) ) ;
#76555=ORIENTED_EDGE ( 'NONE', *, *, #15758, .T. ) ;
#76559=VECTOR ( 'NONE', #73392, 1000.000000000000000 ) ;
#76562=CARTESIAN_POINT ( 'NONE',  ( 4.879999999999994564, 43.00000000000000711, -4.250000000000000000 ) ) ;
#76567=EDGE_LOOP ( 'NONE', ( #61761, #66873, #83175, #31919 ) ) ;
#76582=CARTESIAN_POINT ( 'NONE',  ( -7.118731320094870973, -71.92838106472885329, -2.750000000000000444 ) ) ;
#76584=DIRECTION ( 'NONE',  ( 1.000000000000000000, 0.000000000000000000, 0.000000000000000000 ) ) ;
#76585=STYLED_ITEM ( 'NONE', ( #71784 ), #5038 ) ;
#76595=COLOUR_RGB ( '', 0.40784314, 0.44705882, 0.49803922) ;
#76601=DIRECTION ( 'NONE',  ( 0.000000000000000000, -1.000000000000000000, 0.000000000000000000 ) ) ;
#76602=AXIS2_PLACEMENT_3D ( 'NONE', #15602, #84580, #47557 ) ;
#76621=VERTEX_POINT ( 'NONE', #75243 ) ;
#76628=CARTESIAN_POINT ( 'NONE',  ( -11.05191079938102128, -57.06817940849487059, 4.000000000000000000 ) ) ;
#76640=AXIS2_PLACEMENT_3D ( 'NONE', #33242, #54759, #9774 ) ;
#76642=FACE_OUTER_BOUND ( 'NONE', #18876, .T. ) ;
#76656=ORIENTED_EDGE ( 'NONE', *, *, #21238, .T. ) ;
#76658=CIRCLE ( 'NONE', #46333, 0.2500000000000002220 ) ;
#76678=ORIENTED_EDGE ( 'NONE', *, *, #72341, .T. ) ;
#76691=STYLED_ITEM ( 'NONE', ( #82763 ), #66347 ) ;
#76692=B_SPLINE_CURVE_WITH_KNOTS ( 'NONE', 3,
 ( #89970, #12006, #21486, #13992, #44467, #74969, #6474, #60457, #45962, #7967, #965, #22477 ),
 .UNSPECIFIED., .F., .F.,
 ( 4, 2, 2, 2, 2, 4 ),
 ( 3.878959614448864246E-18, 4.389529495108911855E-05, 8.779058990217436108E-05, 0.0001755811798043448461, 0.0003511623596086858434, 0.0007023247192173684341 ),
 .UNSPECIFIED. ) ;
#76695=DIRECTION ( 'NONE',  ( 0.000000000000000000, -1.000000000000000000, 0.000000000000000000 ) ) ;
#76700=( NAMED_UNIT ( * ) PLANE_ANGLE_UNIT ( ) SI_UNIT ( $, .RADIAN. ) );
#76713=EDGE_CURVE ( 'NONE', #105, #60118, #4787, .T. ) ;
#76723=DIRECTION ( 'NONE',  ( 0.000000000000000000, 0.000000000000000000, -1.000000000000000000 ) ) ;
#76729=CARTESIAN_POINT ( 'NONE',  ( 11.01507687203709018, -96.09620168234333448, -4.000000000000224709 ) ) ;
#76738=AXIS2_PLACEMENT_3D ( 'NONE', #91090, #22618, #91597 ) ;
#76741=ORIENTED_EDGE ( 'NONE', *, *, #93607, .F. ) ;
#76742=VERTEX_POINT ( 'NONE', #74750 ) ;
#76743=AXIS2_PLACEMENT_3D ( 'NONE', #62159, #33623, #1698 ) ;
#76753=EDGE_CURVE ( 'NONE', #43677, #87849, #10053, .T. ) ;
#76754=CARTESIAN_POINT ( 'NONE',  ( 18.00000000000000000, 78.80384757729336798, 3.750000000000000444 ) ) ;
#76757=CARTESIAN_POINT ( 'NONE',  ( -3.522141228383032452, -0.8488377519105255731, 3.750000000000201172 ) ) ;
#76760=VERTEX_POINT ( 'NONE', #57766 ) ;
#76768=MECHANICAL_DESIGN_GEOMETRIC_PRESENTATION_REPRESENTATION('',(#8116),#1845);
#76771=EDGE_CURVE ( 'NONE', #90212, #21688, #91487, .T. ) ;
#76779=FILL_AREA_STYLE ('',( #30778 ) ) ;
#76784=ORIENTED_EDGE ( 'NONE', *, *, #96522, .T. ) ;
#76799=CARTESIAN_POINT ( 'NONE',  ( -5.069387707482587935, -24.96207253826403871, -2.750000000000001776 ) ) ;
#76810=CARTESIAN_POINT ( 'NONE',  ( 4.323026924234770085, -6.401461444633167019, -2.500000000000000000 ) ) ;
#76821=STYLED_ITEM ( 'NONE', ( #2806 ), #33244 ) ;
#76825=SURFACE_STYLE_FILL_AREA ( #861 ) ;
#76829=VERTEX_POINT ( 'NONE', #83552 ) ;
#76837=AXIS2_PLACEMENT_3D ( 'NONE', #53492, #44514, #29008 ) ;
#76841=VERTEX_POINT ( 'NONE', #82560 ) ;
#76842=CARTESIAN_POINT ( 'NONE',  ( -18.89999999999999147, 91.00000000000000000, 8.000000000000000000 ) ) ;
#76881=CARTESIAN_POINT ( 'NONE',  ( 6.935087012919454175, -80.58470470491536730, 4.000000000001609379 ) ) ;
#76883=DIRECTION ( 'NONE',  ( 1.000000000000000000, 0.000000000000000000, 0.000000000000000000 ) ) ;
#76887=EDGE_CURVE ( 'NONE', #40011, #86711, #2157, .T. ) ;
#76891=ORIENTED_EDGE ( 'NONE', *, *, #73921, .F. ) ;
#76909=AXIS2_PLACEMENT_3D ( 'NONE', #7315, #15322, #14826 ) ;
#76914=AXIS2_PLACEMENT_3D ( 'NONE', #23092, #25063, #15099 ) ;
#76923=DIRECTION ( 'NONE',  ( -0.000000000000000000, -0.000000000000000000, 1.000000000000000000 ) ) ;
#76927=CARTESIAN_POINT ( 'NONE',  ( -4.000000000000000000, 36.75000000000000000, 2.750000000000000000 ) ) ;
#76956=DIRECTION ( 'NONE',  ( -0.5905099943842175847, -0.8070303256584298035, 0.000000000000000000 ) ) ;
#76959=CARTESIAN_POINT ( 'NONE',  ( 8.879999999999995453, 41.24999999999999289, -6.250000000000000000 ) ) ;
#76961=DIRECTION ( 'NONE',  ( 0.000000000000000000, 1.000000000000000000, 0.000000000000000000 ) ) ;
#76965=DIRECTION ( 'NONE',  ( 0.000000000000000000, 0.000000000000000000, -1.000000000000000000 ) ) ;
#76976=CARTESIAN_POINT ( 'NONE',  ( -8.000000000000000000, 41.24999999999999289, -4.250000000000000000 ) ) ;
#76977=AXIS2_PLACEMENT_3D ( 'NONE', #36934, #917, #67425 ) ;
#76986=ORIENTED_EDGE ( 'NONE', *, *, #56748, .F. ) ;
#76993=AXIS2_PLACEMENT_3D ( 'NONE', #31009, #61505, #90037 ) ;
#76996=FACE_OUTER_BOUND ( 'NONE', #83337, .T. ) ;
#77000=CARTESIAN_POINT ( 'NONE',  ( -7.374934931933696092, -78.83424294380051833, -4.000000000000000888 ) ) ;
#77008=DIRECTION ( 'NONE',  ( -0.000000000000000000, -0.000000000000000000, -1.000000000000000000 ) ) ;
#77044=DIRECTION ( 'NONE',  ( 8.673617379884028570E-16, 1.000000000000000000, -9.540979117872446908E-15 ) ) ;
#77051=AXIS2_PLACEMENT_3D ( 'NONE', #42737, #35214, #19734 ) ;
#77053=AXIS2_PLACEMENT_3D ( 'NONE', #48367, #41394, #63846 ) ;
#77067=DIRECTION ( 'NONE',  ( 0.000000000000000000, 1.000000000000000000, 0.000000000000000000 ) ) ;
#77076=DIRECTION ( 'NONE',  ( 0.000000000000000000, -0.000000000000000000, 1.000000000000000000 ) ) ;
#77078=DIRECTION ( 'NONE',  ( 0.08715574274765112983, 0.9961946980917461003, 0.000000000000000000 ) ) ;
#77086=LINE ( 'NONE', #92580, #16067 ) ;
#77107=FACE_OUTER_BOUND ( 'NONE', #79767, .T. ) ;
#77118=CARTESIAN_POINT ( 'NONE',  ( -10.79671963681641600, -44.59934526486136974, 3.999999999996397992 ) ) ;
#77123=AXIS2_PLACEMENT_3D ( 'NONE', #44599, #29579, #68596 ) ;
#77125=EDGE_CURVE ( 'NONE', #38057, #10110, #77192, .T. ) ;
#77128=VECTOR ( 'NONE', #70579, 1000.000000000000000 ) ;
#77132=STYLED_ITEM ( 'NONE', ( #37346 ), #77457 ) ;
#77134=ORIENTED_EDGE ( 'NONE', *, *, #50492, .F. ) ;
#77151=CARTESIAN_POINT ( 'NONE',  ( -3.377746357650261988, -3.629174488344649951, 2.499999999999999556 ) ) ;
#77159=DIRECTION ( 'NONE',  ( -0.000000000000000000, -1.000000000000000000, -0.000000000000000000 ) ) ;
#77161=FILL_AREA_STYLE_COLOUR ( '', #43541 ) ;
#77169=ORIENTED_EDGE ( 'NONE', *, *, #87612, .F. ) ;
#77182=CIRCLE ( 'NONE', #45215, 0.2500000000000002220 ) ;
#77183=ORIENTED_EDGE ( 'NONE', *, *, #63876, .F. ) ;
#77192=B_SPLINE_CURVE_WITH_KNOTS ( 'NONE', 3,
 ( #19851, #73837, #13342, #96369, #27842, #13842, #89827, #96867, #50344, #89340 ),
 .UNSPECIFIED., .F., .F.,
 ( 4, 3, 3, 4 ),
 ( -5.954425897502142659E-06, 0.000000000000000000, 6.576041642147462129E-05, 0.0001360868310503591421 ),
 .UNSPECIFIED. ) ;
#77201=CARTESIAN_POINT ( 'NONE',  ( 8.879999999999991900, 27.04366094290857347, 3.000000000000000000 ) ) ;
#77203=EDGE_CURVE ( 'NONE', #38304, #49656, #50851, .T. ) ;
#77214=UNCERTAINTY_MEASURE_WITH_UNIT (LENGTH_MEASURE( 1.000000000000000082E-05 ), #52287, 'distance_accuracy_value', 'NONE');
#77218=EDGE_LOOP ( 'NONE', ( #75932, #17041, #34304, #34388 ) ) ;
#77227=( NAMED_UNIT ( * ) PLANE_ANGLE_UNIT ( ) SI_UNIT ( $, .RADIAN. ) );
#77234=FILL_AREA_STYLE_COLOUR ( '', #58779 ) ;
#77257=ORIENTED_EDGE ( 'NONE', *, *, #21078, .T. ) ;
#77263=ORIENTED_EDGE ( 'NONE', *, *, #88187, .F. ) ;
#77267=LINE ( 'NONE', #24784, #43164 ) ;
#77283=CARTESIAN_POINT ( 'NONE',  ( 4.395798237819382059, -0.8372147401281977430, -3.750000000000000444 ) ) ;
#77296=CARTESIAN_POINT ( 'NONE',  ( -10.34223742324294548, 89.23976162705943693, 5.715022854599767221 ) ) ;
#77319=FILL_AREA_STYLE ('',( #83852 ) ) ;
#77320=LINE ( 'NONE', #75359, #21557 ) ;
#77337=DIRECTION ( 'NONE',  ( -1.000000000000000000, 0.000000000000000000, 0.000000000000000000 ) ) ;
#77341=FACE_OUTER_BOUND ( 'NONE', #81410, .T. ) ;
#77342=FACE_OUTER_BOUND ( 'NONE', #80414, .T. ) ;
#77361=ORIENTED_EDGE ( 'NONE', *, *, #34774, .T. ) ;
#77362=AXIS2_PLACEMENT_3D ( 'NONE', #4329, #64792, #19803 ) ;
#77367=CARTESIAN_POINT ( 'NONE',  ( 5.170525679121678486, -13.81869365337359845, 4.000000000000000000 ) ) ;
#77373=CARTESIAN_POINT ( 'NONE',  ( -3.836041483939801378, -2.701055130266050153, -4.000000000000000888 ) ) ;
#77376=ORIENTED_EDGE ( 'NONE', *, *, #38207, .T. ) ;
#77387=ORIENTED_EDGE ( 'NONE', *, *, #78101, .F. ) ;
#77398=LINE ( 'NONE', #8427, #61806 ) ;
#77401=CARTESIAN_POINT ( 'NONE',  ( -18.00000000000000355, 75.73428692542562146, -2.900000000000000799 ) ) ;
#77403=DIRECTION ( 'NONE',  ( 1.000000000000000000, 1.387778780781444413E-14, 0.000000000000000000 ) ) ;
#77404=CARTESIAN_POINT ( 'NONE',  ( 7.007880867418010418, -58.32092081208355694, -4.000000000000000888 ) ) ;
#77419=CARTESIAN_POINT ( 'NONE',  ( 4.474002695404426966, -3.767820133606233579, -3.750000000000000888 ) ) ;
#77421=CARTESIAN_POINT ( 'NONE',  ( 4.380000000000000782, 1.019547802438464768, 2.500000000000000000 ) ) ;
#77425=CARTESIAN_POINT ( 'NONE',  ( -4.250000000000000000, 36.75000000000000000, 3.750000000000000000 ) ) ;
#77434=EDGE_CURVE ( 'NONE', #33828, #34829, #60806, .T. ) ;
#77456=VERTEX_POINT ( 'NONE', #75319 ) ;
#77457=ADVANCED_FACE ( 'NONE', ( #22834 ), #7831, .T. ) ;
#77464=CIRCLE ( 'NONE', #47127, 10.90000000000026326 ) ;
#77481=ORIENTED_EDGE ( 'NONE', *, *, #97118, .F. ) ;
#77500=ORIENTED_EDGE ( 'NONE', *, *, #19708, .F. ) ;
#77508=CIRCLE ( 'NONE', #24862, 2.999999999999999556 ) ;
#77510=ORIENTED_EDGE ( 'NONE', *, *, #56253, .F. ) ;
#77518=ADVANCED_FACE ( 'NONE', ( #52327 ), #19677, .T. ) ;
#77526=ORIENTED_EDGE ( 'NONE', *, *, #72291, .F. ) ;
#77537=FILL_AREA_STYLE_COLOUR ( '', #74604 ) ;
#77550=EDGE_CURVE ( 'NONE', #25872, #15638, #91559, .T. ) ;
#77554=ORIENTED_EDGE ( 'NONE', *, *, #27201, .F. ) ;
#77563=FILL_AREA_STYLE_COLOUR ( '', #58186 ) ;
#77574=DIRECTION ( 'NONE',  ( 0.000000000000000000, -0.000000000000000000, -1.000000000000000000 ) ) ;
#77587=DIRECTION ( 'NONE',  ( 3.469446951953615372E-15, 1.000000000000000000, 0.000000000000000000 ) ) ;
#77600=ORIENTED_EDGE ( 'NONE', *, *, #23549, .T. ) ;
#77601=EDGE_LOOP ( 'NONE', ( #24586, #1028, #68901, #47668 ) ) ;
#77614=CARTESIAN_POINT ( 'NONE',  ( 6.880000000000009663, 40.99999999999999289, -4.250000000000000000 ) ) ;
#77619=ORIENTED_EDGE ( 'NONE', *, *, #43911, .F. ) ;
#77624=CARTESIAN_POINT ( 'NONE',  ( 9.879999999999990123, 20.99999999999999645, 0.000000000000000000 ) ) ;
#77631=ORIENTED_EDGE ( 'NONE', *, *, #50019, .F. ) ;
#77633=DIRECTION ( 'NONE',  ( 0.000000000000000000, 0.000000000000000000, 1.000000000000000000 ) ) ;
#77648=ORIENTED_EDGE ( 'NONE', *, *, #42020, .T. ) ;
#77653=( LENGTH_UNIT ( ) NAMED_UNIT ( * ) SI_UNIT ( .MILLI., .METRE. ) );
#77655=ORIENTED_EDGE ( 'NONE', *, *, #49221, .T. ) ;
#77661=ORIENTED_EDGE ( 'NONE', *, *, #39973, .F. ) ;
#77662=CARTESIAN_POINT ( 'NONE',  ( 8.880000000000000782, 1.019547802438458550, 4.000000000000000000 ) ) ;
#77668=AXIS2_PLACEMENT_3D ( 'NONE', #91718, #75227, #8226 ) ;
#77672=VERTEX_POINT ( 'NONE', #70796 ) ;
#77673=ADVANCED_FACE ( 'NONE', ( #2313 ), #55279, .F. ) ;
#77675=CARTESIAN_POINT ( 'NONE',  ( 11.60808467749492934, 57.07844016847288060, 0.000000000000000000 ) ) ;
#77680=( LENGTH_UNIT ( ) NAMED_UNIT ( * ) SI_UNIT ( .MILLI., .METRE. ) );
#77683=CARTESIAN_POINT ( 'NONE',  ( 8.630000000000000782, 1.019547802438458550, -4.000000000000000000 ) ) ;
#77717=SURFACE_STYLE_FILL_AREA ( #69740 ) ;
#77725=DIRECTION ( 'NONE',  ( -0.06975647374412534407, -0.9975640502598241977, 0.000000000000000000 ) ) ;
#77735=DIRECTION ( 'NONE',  ( 0.000000000000000000, 1.000000000000000000, 0.000000000000000000 ) ) ;
#77739=CYLINDRICAL_SURFACE ( 'NONE', #27001, 0.1000000000000001166 ) ;
#77757=SURFACE_STYLE_FILL_AREA ( #69783 ) ;
#77764=VECTOR ( 'NONE', #63998, 1000.000000000000000 ) ;
#77770=SURFACE_STYLE_FILL_AREA ( #94245 ) ;
#77779=ADVANCED_FACE ( 'NONE', ( #12234 ), #72242, .T. ) ;
#77781=CLOSED_SHELL ( 'NONE', ( #98824, #5806, #53984, #3619, #68830, #50856, #16760, #50009, #30764, #68443, #26127, #47403, #94843, #85675, #59803, #95150, #12876, #77838, #86498, #21933, #59355, #16265, #14578, #2442 ) ) ;
#77790=FACE_OUTER_BOUND ( 'NONE', #7060, .T. ) ;
#77804=CARTESIAN_POINT ( 'NONE',  ( -7.778994393791476725, -1.060811710739452796, -4.000000000000000000 ) ) ;
#77812=CARTESIAN_POINT ( 'NONE',  ( -7.750355510519348456, 84.07179676972448590, -4.000000000000000000 ) ) ;
#77826=VECTOR ( 'NONE', #16056, 999.9999999999998863 ) ;
#77833=CARTESIAN_POINT ( 'NONE',  ( -19.89999999999999858, 0.000000000000000000, 8.000000000000000000 ) ) ;
#77834=CYLINDRICAL_SURFACE ( 'NONE', #21233, 0.2500000000000002220 ) ;
#77837=CIRCLE ( 'NONE', #37958, 0.2500000000000002220 ) ;
#77838=ADVANCED_FACE ( 'NONE', ( #64726 ), #11253, .T. ) ;
#77841=( GEOMETRIC_REPRESENTATION_CONTEXT ( 3 ) GLOBAL_UNCERTAINTY_ASSIGNED_CONTEXT ( ( #31230 ) ) GLOBAL_UNIT_ASSIGNED_CONTEXT ( ( #91765, #38283, #309 ) ) REPRESENTATION_CONTEXT ( 'NONE', 'WORKASPACE' ) );
#77846=CARTESIAN_POINT ( 'NONE',  ( -7.750000000000000000, 41.24999999999999289, -4.250000000000000000 ) ) ;
#77865=DIRECTION ( 'NONE',  ( 0.6246950475544237324, 0.7808688094430306093, 0.000000000000000000 ) ) ;
#77866=PLANE ( 'NONE',  #74813 ) ;
#77870=CARTESIAN_POINT ( 'NONE',  ( -7.232415441807423129, -88.12698951299773853, -4.000000000000000000 ) ) ;
#77875=AXIS2_PLACEMENT_3D ( 'NONE', #14737, #45213, #75711 ) ;
#77890=ORIENTED_EDGE ( 'NONE', *, *, #56253, .T. ) ;
#77897=CARTESIAN_POINT ( 'NONE',  ( -10.77730536144846596, -98.63085534186639336, 3.750000000000000000 ) ) ;
#77901=DIRECTION ( 'NONE',  ( 1.000000000000000000, 1.483861936729427615E-16, 0.000000000000000000 ) ) ;
#77904=DIRECTION ( 'NONE',  ( 0.000000000000000000, 0.000000000000000000, 1.000000000000000000 ) ) ;
#77905=DIRECTION ( 'NONE',  ( 1.000000000000000000, 0.000000000000000000, 0.000000000000000000 ) ) ;
#77909=LINE ( 'NONE', #9419, #23043 ) ;
#77911=ADVANCED_FACE ( 'NONE', ( #65722 ), #96248, .T. ) ;
#77912=CARTESIAN_POINT ( 'NONE',  ( -3.750000000000000888, 1.019547802438465212, -4.000000000000000000 ) ) ;
#77918=EDGE_CURVE ( 'NONE', #54753, #13947, #35728, .T. ) ;
#77925=CARTESIAN_POINT ( 'NONE',  ( 4.669733657693289963, -13.81599790096684899, 2.500000000000000000 ) ) ;
#77929=DIRECTION ( 'NONE',  ( 0.000000000000000000, 0.000000000000000000, 1.000000000000000000 ) ) ;
#77935=CARTESIAN_POINT ( 'NONE',  ( -3.750000000000000000, 36.75000000000000000, 3.750000000000000000 ) ) ;
#77941=CARTESIAN_POINT ( 'NONE',  ( -3.750000000000000000, 37.25000000000000000, -4.000000000000000000 ) ) ;
#77947=SURFACE_SIDE_STYLE ('',( #991 ) ) ;
#77968=DIRECTION ( 'NONE',  ( -0.8073289077886854903, 0.5901017155107486367, 0.000000000000000000 ) ) ;
#77972=SURFACE_SIDE_STYLE ('',( #93469 ) ) ;
#77973=FACE_OUTER_BOUND ( 'NONE', #8625, .T. ) ;
#77993=DIRECTION ( 'NONE',  ( 0.000000000000000000, 0.000000000000000000, -1.000000000000000000 ) ) ;
#78041=EDGE_CURVE ( 'NONE', #16571, #15515, #95884, .T. ) ;
#78043=SURFACE_STYLE_USAGE ( .BOTH. , #24572 ) ;
#78047=ORIENTED_EDGE ( 'NONE', *, *, #87137, .F. ) ;
#78052=( GEOMETRIC_REPRESENTATION_CONTEXT ( 3 ) GLOBAL_UNCERTAINTY_ASSIGNED_CONTEXT ( ( #88295 ) ) GLOBAL_UNIT_ASSIGNED_CONTEXT ( ( #32216, #23772, #24741 ) ) REPRESENTATION_CONTEXT ( 'NONE', 'WORKASPACE' ) );
#78056=CARTESIAN_POINT ( 'NONE',  ( -8.900000000000002132, 75.76920769491746910, -2.900000000000000355 ) ) ;
#78066=CARTESIAN_POINT ( 'NONE',  ( -6.445967608602039434, -48.01283281809150338, -2.750000000000000444 ) ) ;
#78068=FACE_OUTER_BOUND ( 'NONE', #81510, .T. ) ;
#78076=COLOUR_RGB ( '', 0.66274510, 0.83137255, 0.94901961) ;
#78077=CARTESIAN_POINT ( 'NONE',  ( -10.77984007285762047, -96.52126437879435628, 3.999999999999999112 ) ) ;
#78086=CARTESIAN_POINT ( 'NONE',  ( 5.129999999999994564, 43.00000000000000711, -6.500000000000000888 ) ) ;
#78087=FILL_AREA_STYLE_COLOUR ( '', #43296 ) ;
#78101=EDGE_CURVE ( 'NONE', #83910, #11101, #67187, .T. ) ;
#78103=LINE ( 'NONE', #34057, #15326 ) ;
#78119=ORIENTED_EDGE ( 'NONE', *, *, #16476, .T. ) ;
#78121=CARTESIAN_POINT ( 'NONE',  ( 46.27857419604806211, 63.24738473459895260, -8.000000000000000000 ) ) ;
#78131=EDGE_CURVE ( 'NONE', #70674, #88822, #91192, .T. ) ;
#78136=ORIENTED_EDGE ( 'NONE', *, *, #29682, .T. ) ;
#78149=CARTESIAN_POINT ( 'NONE',  ( -3.500000000000000444, 0.09224605989676173956, 2.750000000000000000 ) ) ;
#78150=ORIENTED_EDGE ( 'NONE', *, *, #57339, .F. ) ;
#78151=FILL_AREA_STYLE ('',( #23702 ) ) ;
#78155=EDGE_CURVE ( 'NONE', #55638, #1168, #37717, .T. ) ;
#78158=DIRECTION ( 'NONE',  ( 1.000000000000000000, 0.000000000000000000, 0.000000000000000000 ) ) ;
#78162=ORIENTED_EDGE ( 'NONE', *, *, #64, .F. ) ;
#78166=VECTOR ( 'NONE', #94796, 1000.000000000000000 ) ;
#78169=CARTESIAN_POINT ( 'NONE',  ( 4.469999999999999751, 36.75000000000000000, -4.000000000000000000 ) ) ;
#78177=FILL_AREA_STYLE ('',( #47175 ) ) ;
#78178=CARTESIAN_POINT ( 'NONE',  ( 11.34661744925197624, 54.08985607419764818, 0.000000000000000000 ) ) ;
#78204=CARTESIAN_POINT ( 'NONE',  ( 4.879999999999991900, 76.07179676972444327, -6.250000000000000000 ) ) ;
#78211=DIRECTION ( 'NONE',  ( 0.000000000000000000, 0.000000000000000000, 1.000000000000000000 ) ) ;
#78215=UNCERTAINTY_MEASURE_WITH_UNIT (LENGTH_MEASURE( 1.000000000000000082E-05 ), #91181, 'distance_accuracy_value', 'NONE');
#78217=ORIENTED_EDGE ( 'NONE', *, *, #46303, .F. ) ;
#78218=EDGE_LOOP ( 'NONE', ( #44693, #32744, #61609, #36162 ) ) ;
#78220=LINE ( 'NONE', #67903, #63851 ) ;
#78229=CARTESIAN_POINT ( 'NONE',  ( -8.000000000000000000, 0.000000000000000000, 3.750000000000000000 ) ) ;
#78233=CARTESIAN_POINT ( 'NONE',  ( -7.080143328648152767, -69.54337233422636189, 3.750000000000000444 ) ) ;
#78234=EDGE_LOOP ( 'NONE', ( #67280, #64927, #93993, #13089 ) ) ;
#78242=DIRECTION ( 'NONE',  ( 0.000000000000000000, 0.000000000000000000, 1.000000000000000000 ) ) ;
#78252=VERTEX_POINT ( 'NONE', #62656 ) ;
#78266=ADVANCED_FACE ( 'NONE', ( #31669 ), #70403, .F. ) ;
#78269=VECTOR ( 'NONE', #22888, 1000.000000000000114 ) ;
#78276=CARTESIAN_POINT ( 'NONE',  ( -7.037762029935627162, -86.26090954799332167, -2.749999999999999556 ) ) ;
#78286=CARTESIAN_POINT ( 'NONE',  ( 0.000000000000000000, 40.74999999999999289, 4.000000000000000000 ) ) ;
#78292=CARTESIAN_POINT ( 'NONE',  ( 6.829574850505127692, -88.00372650098204019, -2.750000000000000444 ) ) ;
#78304=( GEOMETRIC_REPRESENTATION_CONTEXT ( 3 ) GLOBAL_UNCERTAINTY_ASSIGNED_CONTEXT ( ( #88274 ) ) GLOBAL_UNIT_ASSIGNED_CONTEXT ( ( #41169, #78663, #84685 ) ) REPRESENTATION_CONTEXT ( 'NONE', 'WORKASPACE' ) );
#78323=CYLINDRICAL_SURFACE ( 'NONE', #87829, 0.2500000000000002220 ) ;
#78328=FILL_AREA_STYLE ('',( #69367 ) ) ;
#78353=VECTOR ( 'NONE', #68669, 1000.000000000000000 ) ;
#78355=ORIENTED_EDGE ( 'NONE', *, *, #90876, .T. ) ;
#78361=ADVANCED_FACE ( 'NONE', ( #32154 ), #17676, .T. ) ;
#78363=DIRECTION ( 'NONE',  ( -0.000000000000000000, 0.000000000000000000, 1.000000000000000000 ) ) ;
#78382=EDGE_LOOP ( 'NONE', ( #692, #94506, #41144, #85872 ) ) ;
#78398=CARTESIAN_POINT ( 'NONE',  ( 8.880000000000000782, 1.116573172248542834E-15, 4.000000000000000000 ) ) ;
#78401=MECHANICAL_DESIGN_GEOMETRIC_PRESENTATION_REPRESENTATION('',(#40153),#91175);
#78407=CIRCLE ( 'NONE', #14563, 9.900000000000002132 ) ;
#78417=CARTESIAN_POINT ( 'NONE',  ( 4.441081520556267925, -2.684960557654440638, 2.500000000000000000 ) ) ;
#78432=CARTESIAN_POINT ( 'NONE',  ( -6.030006457149878152, -39.79017371238850842, -2.750000000000000000 ) ) ;
#78436=CARTESIAN_POINT ( 'NONE',  ( -6.732636091893175134, -88.11213685669365248, -2.750000000000000000 ) ) ;
#78452=EDGE_CURVE ( 'NONE', #80099, #76621, #46412, .T. ) ;
#78455=UNCERTAINTY_MEASURE_WITH_UNIT (LENGTH_MEASURE( 1.000000000000000082E-05 ), #74105, 'distance_accuracy_value', 'NONE');
#78456=STYLED_ITEM ( 'NONE', ( #42305 ), #80504 ) ;
#78480=EDGE_LOOP ( 'NONE', ( #72768, #64962, #21305, #88995 ) ) ;
#78485=EDGE_CURVE ( 'NONE', #72511, #59916, #47158, .T. ) ;
#78493=CARTESIAN_POINT ( 'NONE',  ( -8.108527105141890345, -3.139510826252087661, -3.750000000000000888 ) ) ;
#78500=( GEOMETRIC_REPRESENTATION_CONTEXT ( 3 ) GLOBAL_UNCERTAINTY_ASSIGNED_CONTEXT ( ( #31111 ) ) GLOBAL_UNIT_ASSIGNED_CONTEXT ( ( #85113, #55091, #41603 ) ) REPRESENTATION_CONTEXT ( 'NONE', 'WORKASPACE' ) );
#78518=SURFACE_STYLE_FILL_AREA ( #47029 ) ;
#78540=FILL_AREA_STYLE ('',( #79526 ) ) ;
#78558=AXIS2_PLACEMENT_3D ( 'NONE', #5939, #12931, #67419 ) ;
#78560=CARTESIAN_POINT ( 'NONE',  ( 18.00000000000001776, 4.625929269271493211E-15, 8.000000000000000000 ) ) ;
#78571=CARTESIAN_POINT ( 'NONE',  ( -11.37646734096567336, -81.99481244925677004, 4.000000000000000000 ) ) ;
#78572=EDGE_CURVE ( 'NONE', #54617, #2021, #81594, .T. ) ;
#78582=DIRECTION ( 'NONE',  ( 0.6246950475544238435, 0.7808688094430307203, 0.000000000000000000 ) ) ;
#78588=FACE_OUTER_BOUND ( 'NONE', #98817, .T. ) ;
#78596=DIRECTION ( 'NONE',  ( 0.000000000000000000, 0.000000000000000000, 1.000000000000000000 ) ) ;
#78627=FILL_AREA_STYLE_COLOUR ( '', #88575 ) ;
#78628=DIRECTION ( 'NONE',  ( -0.000000000000000000, -0.000000000000000000, 1.000000000000000000 ) ) ;
#78633=ORIENTED_EDGE ( 'NONE', *, *, #17873, .F. ) ;
#78650=CARTESIAN_POINT ( 'NONE',  ( -5.068142462294323636, -24.94450071860671514, 2.499999999999194422 ) ) ;
#78652=CARTESIAN_POINT ( 'NONE',  ( 0.000000000000000000, -97.00000000000000000, 3.750000000000000000 ) ) ;
#78656=CARTESIAN_POINT ( 'NONE',  ( -3.530007528296587704, -1.230351260576522110, 3.750000000000000444 ) ) ;
#78663=( NAMED_UNIT ( * ) PLANE_ANGLE_UNIT ( ) SI_UNIT ( $, .RADIAN. ) );
#78692=ADVANCED_FACE ( 'NONE', ( #27611 ), #26626, .F. ) ;
#78699=DIRECTION ( 'NONE',  ( 1.483861936729427615E-16, -1.000000000000000000, 0.000000000000000000 ) ) ;
#78701=CIRCLE ( 'NONE', #35581, 0.2500000000000002220 ) ;
#78707=CARTESIAN_POINT ( 'NONE',  ( 8.991946320824435901, -4.139779132958989472, -4.000000000000000000 ) ) ;
#78716=( NAMED_UNIT ( * ) SI_UNIT ( $, .STERADIAN. ) SOLID_ANGLE_UNIT ( ) );
#78717=EDGE_LOOP ( 'NONE', ( #8028, #66097, #10228, #49213 ) ) ;
#78720=CYLINDRICAL_SURFACE ( 'NONE', #83006, 0.2500000000000002220 ) ;
#78733=ADVANCED_FACE ( 'NONE', ( #87128 ), #18649, .T. ) ;
#78735=AXIS2_PLACEMENT_3D ( 'NONE', #33338, #33819, #17868 ) ;
#78736=DIRECTION ( 'NONE',  ( -0.08715574274765114371, -0.9961946980917462113, 0.000000000000000000 ) ) ;
#78737=ORIENTED_EDGE ( 'NONE', *, *, #93027, .T. ) ;
#78739=ORIENTED_EDGE ( 'NONE', *, *, #64, .T. ) ;
#78741=EDGE_LOOP ( 'NONE', ( #5663, #78998, #38632, #86877 ) ) ;
#78745=AXIS2_PLACEMENT_3D ( 'NONE', #93940, #3931, #33413 ) ;
#78750=CIRCLE ( 'NONE', #8436, 7.000000000000002665 ) ;
#78755=ORIENTED_EDGE ( 'NONE', *, *, #43268, .F. ) ;
#78760=DIRECTION ( 'NONE',  ( 1.000000000000000000, 0.000000000000000000, 0.000000000000000000 ) ) ;
#78763=LINE ( 'NONE', #10272, #94529 ) ;
#78764=DIRECTION ( 'NONE',  ( 1.483861936729427615E-16, -1.000000000000000000, -0.000000000000000000 ) ) ;
#78769=AXIS2_PLACEMENT_3D ( 'NONE', #11540, #88522, #73509 ) ;
#78788=CARTESIAN_POINT ( 'NONE',  ( -8.669785729375572458, 87.01784090252159842, 4.324025984537457568 ) ) ;
#78799=CARTESIAN_POINT ( 'NONE',  ( 17.99999999999999645, 78.20646178170991902, -3.828774214053709990 ) ) ;
#78808=FILL_AREA_STYLE_COLOUR ( '', #58197 ) ;
#78816=ORIENTED_EDGE ( 'NONE', *, *, #11409, .T. ) ;
#78824=CARTESIAN_POINT ( 'NONE',  ( 8.630000000000002558, -0.01510857754941254301, -4.000000000000000000 ) ) ;
#78828=FILL_AREA_STYLE_COLOUR ( '', #98613 ) ;
#78845=VECTOR ( 'NONE', #27423, 1000.000000000000000 ) ;
#78854=ORIENTED_EDGE ( 'NONE', *, *, #94864, .F. ) ;
#78886=CARTESIAN_POINT ( 'NONE',  ( -8.899009838862365740, -15.58694756607049570, 3.749999999999999112 ) ) ;
#78891=EDGE_CURVE ( 'NONE', #53272, #21472, #75172, .T. ) ;
#78897=CYLINDRICAL_SURFACE ( 'NONE', #50197, 0.2500000000000002220 ) ;
#78900=AXIS2_PLACEMENT_3D ( 'NONE', #6163, #75143, #67662 ) ;
#78904=EDGE_LOOP ( 'NONE', ( #30527, #8651, #37202, #45950 ) ) ;
#78917=CARTESIAN_POINT ( 'NONE',  ( 10.35044781186116936, -32.03405546004147908, 3.750000000000000000 ) ) ;
#78924=EDGE_LOOP ( 'NONE', ( #21371, #84763, #43074, #30421 ) ) ;
#78927=CARTESIAN_POINT ( 'NONE',  ( -3.500000000000000444, 1.019547802438453887, -2.750000000000000000 ) ) ;
#78928=DIRECTION ( 'NONE',  ( -1.000000000000000000, 0.000000000000000000, 0.000000000000000000 ) ) ;
#78933=CARTESIAN_POINT ( 'NONE',  ( 4.645844135293939914, -0.8374644621422210333, -4.000000000000000000 ) ) ;
#78944=CIRCLE ( 'NONE', #26260, 0.2500000000000002220 ) ;
#78969=ORIENTED_EDGE ( 'NONE', *, *, #3989, .F. ) ;
#78980=DIRECTION ( 'NONE',  ( 1.000000000000000000, -0.000000000000000000, -0.000000000000000000 ) ) ;
#78996=AXIS2_PLACEMENT_3D ( 'NONE', #9828, #71800, #64275 ) ;
#78998=ORIENTED_EDGE ( 'NONE', *, *, #43116, .F. ) ;
#79007=CARTESIAN_POINT ( 'NONE',  ( -5.999999999999994671, 43.00000000000000000, -6.500000000000000888 ) ) ;
#79015=ORIENTED_EDGE ( 'NONE', *, *, #9608, .T. ) ;
#79024=ORIENTED_EDGE ( 'NONE', *, *, #1773, .T. ) ;
#79050=FACE_OUTER_BOUND ( 'NONE', #72001, .T. ) ;
#79052=CARTESIAN_POINT ( 'NONE',  ( -10.95083791870221823, -94.44918831364067557, -4.000000000000000888 ) ) ;
#79053=CARTESIAN_POINT ( 'NONE',  ( -11.33435148536054271, -69.53340079814059038, 4.000000000000000000 ) ) ;
#79058=AXIS2_PLACEMENT_3D ( 'NONE', #67758, #274, #90239 ) ;
#79064=CARTESIAN_POINT ( 'NONE',  ( 11.10000000000000142, 98.49999999999998579, 8.000000000000000000 ) ) ;
#79079=CIRCLE ( 'NONE', #32751, 1.750000000000000666 ) ;
#79081=CARTESIAN_POINT ( 'NONE',  ( 10.83696084481538691, -98.17058944465519232, -3.750000000000000000 ) ) ;
#79084=VERTEX_POINT ( 'NONE', #46079 ) ;
#79103=FILL_AREA_STYLE ('',( #24642 ) ) ;
#79128=CARTESIAN_POINT ( 'NONE',  ( -4.259797194937135600, -13.81744876718661885, 2.500000000000001776 ) ) ;
#79130=CARTESIAN_POINT ( 'NONE',  ( 11.18123354744523468, -92.99280210685034831, 3.750000000000000000 ) ) ;
#79133=DIRECTION ( 'NONE',  ( -1.049065152435176504E-16, 1.000000000000000000, 0.000000000000000000 ) ) ;
#79135=CARTESIAN_POINT ( 'NONE',  ( -6.757332319902496387, -55.97232334539076959, 3.750000000000000444 ) ) ;
#79138=CARTESIAN_POINT ( 'NONE',  ( 15.00000000000000178, 73.00000000000000000, 6.250000000000000000 ) ) ;
#79150=VECTOR ( 'NONE', #61858, 1000.000000000000000 ) ;
#79166=CARTESIAN_POINT ( 'NONE',  ( -8.000000000000000000, 80.99999999999994316, 1.249999999999987121 ) ) ;
#79167=CARTESIAN_POINT ( 'NONE',  ( 9.879999999999990123, 20.99999999999999645, 0.000000000000000000 ) ) ;
#79196=DIRECTION ( 'NONE',  ( 0.000000000000000000, 1.000000000000000000, 0.000000000000000000 ) ) ;
#79198=ADVANCED_FACE ( 'NONE', ( #36006 ), #41567, .F. ) ;
#79233=EDGE_LOOP ( 'NONE', ( #49929, #15309, #47032, #11839 ) ) ;
#79274=CARTESIAN_POINT ( 'NONE',  ( -10.06059601896260247, 88.97539449291203084, 5.490105317800513696 ) ) ;
#79275=AXIS2_PLACEMENT_3D ( 'NONE', #87627, #94644, #33147 ) ;
#79281=SURFACE_SIDE_STYLE ('',( #48775 ) ) ;
#79285=SURFACE_STYLE_USAGE ( .BOTH. , #85810 ) ;
#79286=CARTESIAN_POINT ( 'NONE',  ( -1.899999999999997247, 98.49999999999998579, 8.000000000000000000 ) ) ;
#79290=CIRCLE ( 'NONE', #96872, 2.000000000000000888 ) ;
#79294=COLOUR_RGB ( '', 0.31764706, 0.68627451, 0.89019608) ;
#79295=CARTESIAN_POINT ( 'NONE',  ( -5.810051007611032325, -36.09132727650185757, 2.750000000000000000 ) ) ;
#79300=CARTESIAN_POINT ( 'NONE',  ( -8.224651678658434051, 85.81254401277075772, -3.937446577531860559 ) ) ;
#79308=EDGE_LOOP ( 'NONE', ( #52758, #39513, #58446, #92161 ) ) ;
#79369=AXIS2_PLACEMENT_3D ( 'NONE', #9954, #19416, #71922 ) ;
#79377=MECHANICAL_DESIGN_GEOMETRIC_PRESENTATION_REPRESENTATION('',(#65001),#57023);
#79382=CARTESIAN_POINT ( 'NONE',  ( -8.000000000000000000, 1.019547802438458550, 3.750000000000000000 ) ) ;
#79392=DIRECTION ( 'NONE',  ( 0.000000000000000000, 0.000000000000000000, -1.000000000000000000 ) ) ;
#79397=STYLED_ITEM ( 'NONE', ( #62042 ), #89831 ) ;
#79400=ORIENTED_EDGE ( 'NONE', *, *, #13576, .F. ) ;
#79404=EDGE_CURVE ( 'NONE', #23594, #91180, #54468, .T. ) ;
#79408=AXIS2_PLACEMENT_3D ( 'NONE', #61540, #77044, #17543 ) ;
#79412=CARTESIAN_POINT ( 'NONE',  ( 6.685134130355901760, -80.57704203043711289, 2.500000000000000888 ) ) ;
#79415=ORIENTED_EDGE ( 'NONE', *, *, #44484, .T. ) ;
#79418=CARTESIAN_POINT ( 'NONE',  ( 11.20713776170701870, -56.83174664233160911, 3.750000000000000444 ) ) ;
#79419=CIRCLE ( 'NONE', #55519, 0.2499999999999997224 ) ;
#79422=VECTOR ( 'NONE', #16007, 1000.000000000000000 ) ;
#79428=( NAMED_UNIT ( * ) SI_UNIT ( $, .STERADIAN. ) SOLID_ANGLE_UNIT ( ) );
#79433=CARTESIAN_POINT ( 'NONE',  ( 4.920853330076631060, -13.83152733636334020, -4.000000000001609379 ) ) ;
#79436=CARTESIAN_POINT ( 'NONE',  ( 14.99999999999998046, 70.25000000000000000, 6.500000000000000888 ) ) ;
#79451=EDGE_LOOP ( 'NONE', ( #90336, #22673, #12280, #52673 ) ) ;
#79453=FILL_AREA_STYLE ('',( #9480 ) ) ;
#79459=CIRCLE ( 'NONE', #48874, 0.2500000000000002220 ) ;
#79481=CARTESIAN_POINT ( 'NONE',  ( 6.880000000000011440, 40.74999999999999289, -4.000000000000000000 ) ) ;
#79484=CIRCLE ( 'NONE', #73094, 0.2500000000000002220 ) ;
#79494=MECHANICAL_DESIGN_GEOMETRIC_PRESENTATION_REPRESENTATION('',(#85918),#42804);
#79504=CARTESIAN_POINT ( 'NONE',  ( -3.638307330400850415, -8.269691488429797843, 2.499999999999999556 ) ) ;
#79512=DIRECTION ( 'NONE',  ( 0.000000000000000000, 0.000000000000000000, 1.000000000000000000 ) ) ;
#79519=UNCERTAINTY_MEASURE_WITH_UNIT (LENGTH_MEASURE( 1.000000000000000082E-05 ), #29817, 'distance_accuracy_value', 'NONE');
#79520=LINE ( 'NONE', #33992, #53547 ) ;
#79523=( NAMED_UNIT ( * ) SI_UNIT ( $, .STERADIAN. ) SOLID_ANGLE_UNIT ( ) );
#79526=FILL_AREA_STYLE_COLOUR ( '', #97849 ) ;
#79527=VERTEX_POINT ( 'NONE', #37505 ) ;
#79540=EDGE_LOOP ( 'NONE', ( #91425, #38055, #90839, #72207 ) ) ;
#79547=DIRECTION ( 'NONE',  ( 0.000000000000000000, 1.000000000000000000, 0.000000000000000000 ) ) ;
#79550=VECTOR ( 'NONE', #17183, 1000.000000000000000 ) ;
#79557=( GEOMETRIC_REPRESENTATION_CONTEXT ( 3 ) GLOBAL_UNCERTAINTY_ASSIGNED_CONTEXT ( ( #9350 ) ) GLOBAL_UNIT_ASSIGNED_CONTEXT ( ( #41081, #55073, #7461 ) ) REPRESENTATION_CONTEXT ( 'NONE', 'WORKASPACE' ) );
#79570=CARTESIAN_POINT ( 'NONE',  ( -7.079957117332396521, -69.52918679324339735, -3.750000000000000000 ) ) ;
#79572=ORIENTED_EDGE ( 'NONE', *, *, #96999, .F. ) ;
#79587=VERTEX_POINT ( 'NONE', #59495 ) ;
#79592=CYLINDRICAL_SURFACE ( 'NONE', #41151, 0.09999999999999939493 ) ;
#79609=( GEOMETRIC_REPRESENTATION_CONTEXT ( 3 ) GLOBAL_UNCERTAINTY_ASSIGNED_CONTEXT ( ( #9215 ) ) GLOBAL_UNIT_ASSIGNED_CONTEXT ( ( #31377, #23419, #31864 ) ) REPRESENTATION_CONTEXT ( 'NONE', 'WORKASPACE' ) );
#79614=ORIENTED_EDGE ( 'NONE', *, *, #93247, .F. ) ;
#79621=CARTESIAN_POINT ( 'NONE',  ( 17.75000000000000355, 78.80384757729335377, -4.000000000000000000 ) ) ;
#79625=LINE ( 'NONE', #11126, #15408 ) ;
#79628=CARTESIAN_POINT ( 'NONE',  ( 11.15633734011313294, -69.21829398629044761, 4.000000000000000000 ) ) ;
#79642=( NAMED_UNIT ( * ) SI_UNIT ( $, .STERADIAN. ) SOLID_ANGLE_UNIT ( ) );
#79646=SURFACE_STYLE_FILL_AREA ( #27616 ) ;
#79665=DIRECTION ( 'NONE',  ( 0.000000000000000000, 0.000000000000000000, -1.000000000000000000 ) ) ;
#79683=CARTESIAN_POINT ( 'NONE',  ( 17.82151337995249207, 90.99999999999998579, -8.000000000000000000 ) ) ;
#79684=CARTESIAN_POINT ( 'NONE',  ( 4.400664535130860422, -1.180071741297640253, 2.750000000000000000 ) ) ;
#79693=MECHANICAL_DESIGN_GEOMETRIC_PRESENTATION_REPRESENTATION('',(#14254),#41398);
#79694=ADVANCED_FACE ( 'NONE', ( #24473 ), #69963, .T. ) ;
#79697=FILL_AREA_STYLE_COLOUR ( '', #70658 ) ;
#79708=EDGE_CURVE ( 'NONE', #64082, #91314, #21407, .T. ) ;
#79716=FACE_OUTER_BOUND ( 'NONE', #59071, .T. ) ;
#79717=VERTEX_POINT ( 'NONE', #76959 ) ;
#79727=EDGE_CURVE ( 'NONE', #74593, #8279, #8956, .T. ) ;
#79729=ORIENTED_EDGE ( 'NONE', *, *, #69638, .T. ) ;
#79731=VERTEX_POINT ( 'NONE', #23977 ) ;
#79741=VECTOR ( 'NONE', #25582, 1000.000000000000000 ) ;
#79743=CARTESIAN_POINT ( 'NONE',  ( -8.000000000000000000, 83.99999999999994316, -3.750000000000000000 ) ) ;
#79749=DIRECTION ( 'NONE',  ( 0.000000000000000000, 0.000000000000000000, -1.000000000000000000 ) ) ;
#79765=CARTESIAN_POINT ( 'NONE',  ( -12.98310705059785164, 90.76710648773764945, 7.614994760437721055 ) ) ;
#79767=EDGE_LOOP ( 'NONE', ( #71523, #71384, #56291 ) ) ;
#79778=CARTESIAN_POINT ( 'NONE',  ( 4.380000000000001670, 0.09073877121621831687, 3.750000000000000888 ) ) ;
#79779=DIRECTION ( 'NONE',  ( 1.000000000000000000, 0.000000000000000000, 0.000000000000000000 ) ) ;
#79783=EDGE_LOOP ( 'NONE', ( #30270, #29063, #87986, #36848 ) ) ;
#79787=CARTESIAN_POINT ( 'NONE',  ( -8.048010592883702685, 84.92462609336300261, -4.034077756265262771 ) ) ;
#79791=EDGE_CURVE ( 'NONE', #88687, #54112, #41716, .T. ) ;
#79795=ORIENTED_EDGE ( 'NONE', *, *, #28919, .F. ) ;
#79802=AXIS2_PLACEMENT_3D ( 'NONE', #61322, #59842, #7850 ) ;
#79818=EDGE_CURVE ( 'NONE', #14873, #45794, #65664, .T. ) ;
#79829=VERTEX_POINT ( 'NONE', #93937 ) ;
#79852=CYLINDRICAL_SURFACE ( 'NONE', #28743, 0.09999999999999939493 ) ;
#79863=ORIENTED_EDGE ( 'NONE', *, *, #15312, .F. ) ;
#79871=CARTESIAN_POINT ( 'NONE',  ( 14.99999999999997868, 79.82179676972448590, 6.250000000000000000 ) ) ;
#79894=ADVANCED_FACE ( 'NONE', ( #64403 ), #33410, .F. ) ;
#79895=CARTESIAN_POINT ( 'NONE',  ( 11.40653762822727835, -69.23734991727425836, 3.750000000000000444 ) ) ;
#79910=CARTESIAN_POINT ( 'NONE',  ( 4.657035931814768048, -8.268334176803392666, -3.749999999999597211 ) ) ;
#79913=CARTESIAN_POINT ( 'NONE',  ( -3.878335320991981305, -3.629921146508676255, 4.000000000000000000 ) ) ;
#79923=VECTOR ( 'NONE', #83184, 1000.000000000000000 ) ;
#79935=CARTESIAN_POINT ( 'NONE',  ( 4.600000000000003197, 98.49999999999998579, -8.000000000000000000 ) ) ;
#79936=DIRECTION ( 'NONE',  ( 1.000000000000000000, 1.257402221000611116E-16, -0.000000000000000000 ) ) ;
#79954=MECHANICAL_DESIGN_GEOMETRIC_PRESENTATION_REPRESENTATION('',(#124),#78304);
#79962=CARTESIAN_POINT ( 'NONE',  ( -11.19838940738413235, -94.49360967301636549, -3.750000000000000000 ) ) ;
#79983=( GEOMETRIC_REPRESENTATION_CONTEXT ( 3 ) GLOBAL_UNCERTAINTY_ASSIGNED_CONTEXT ( ( #66398 ) ) GLOBAL_UNIT_ASSIGNED_CONTEXT ( ( #75256, #22278, #29746 ) ) REPRESENTATION_CONTEXT ( 'NONE', 'WORKASPACE' ) );
#80004=DIRECTION ( 'NONE',  ( 0.000000000000000000, -1.000000000000000000, 0.000000000000000000 ) ) ;
#80006=CARTESIAN_POINT ( 'NONE',  ( 8.776446609406717059, 70.10355339059326241, 6.500000000000001776 ) ) ;
#80012=MECHANICAL_DESIGN_GEOMETRIC_PRESENTATION_REPRESENTATION('',(#1820),#30547);
#80015=ADVANCED_FACE ( 'NONE', ( #87893 ), #19410, .F. ) ;
#80038=( NAMED_UNIT ( * ) PLANE_ANGLE_UNIT ( ) SI_UNIT ( $, .RADIAN. ) );
#80049=CARTESIAN_POINT ( 'NONE',  ( -5.329506769333839600, -28.66963596002775816, -3.750000000000001332 ) ) ;
#80051=AXIS2_PLACEMENT_3D ( 'NONE', #13028, #42547, #88536 ) ;
#80053=ORIENTED_EDGE ( 'NONE', *, *, #51059, .T. ) ;
#80067=DIRECTION ( 'NONE',  ( -1.000000000000000000, -0.000000000000000000, -0.000000000000000000 ) ) ;
#80091=( GEOMETRIC_REPRESENTATION_CONTEXT ( 3 ) GLOBAL_UNCERTAINTY_ASSIGNED_CONTEXT ( ( #19430 ) ) GLOBAL_UNIT_ASSIGNED_CONTEXT ( ( #27753, #81255, #19277 ) ) REPRESENTATION_CONTEXT ( 'NONE', 'WORKASPACE' ) );
#80099=VERTEX_POINT ( 'NONE', #93927 ) ;
#80105=( NAMED_UNIT ( * ) SI_UNIT ( $, .STERADIAN. ) SOLID_ANGLE_UNIT ( ) );
#80106=CIRCLE ( 'NONE', #24255, 0.09999999999999982514 ) ;
#80108=ORIENTED_EDGE ( 'NONE', *, *, #53064, .T. ) ;
#80109=CARTESIAN_POINT ( 'NONE',  ( 9.209315896096745391, -9.300848983894347555, 4.000000000000000000 ) ) ;
#80116=CARTESIAN_POINT ( 'NONE',  ( -5.999999999999994671, 43.00000000000000000, 6.250000000000000000 ) ) ;
#80120=DIRECTION ( 'NONE',  ( 0.08715574274765129636, 0.9961946980917462113, 0.000000000000000000 ) ) ;
#80123=( GEOMETRIC_REPRESENTATION_CONTEXT ( 3 ) GLOBAL_UNCERTAINTY_ASSIGNED_CONTEXT ( ( #24130 ) ) GLOBAL_UNIT_ASSIGNED_CONTEXT ( ( #91066, #90082, #43597 ) ) REPRESENTATION_CONTEXT ( 'NONE', 'WORKASPACE' ) );
#80127=EDGE_CURVE ( 'NONE', #60118, #24768, #12997, .T. ) ;
#80133=VERTEX_POINT ( 'NONE', #39944 ) ;
#80140=CARTESIAN_POINT ( 'NONE',  ( 6.564124673094354101, -0.5742864948665229452, 2.900000000000000355 ) ) ;
#80146=CARTESIAN_POINT ( 'NONE',  ( -10.85639882392407074, -98.10817599973766789, -3.750000000004759304 ) ) ;
#80148=FACE_OUTER_BOUND ( 'NONE', #76567, .T. ) ;
#80160=FACE_BOUND ( 'NONE', #24564, .T. ) ;
#80166=ORIENTED_EDGE ( 'NONE', *, *, #59734, .F. ) ;
#80168=CARTESIAN_POINT ( 'NONE',  ( 6.903457398626330566, -84.61157762779829739, 2.749999999999999556 ) ) ;
#80179=ORIENTED_EDGE ( 'NONE', *, *, #1458, .T. ) ;
#80180=LINE ( 'NONE', #64667, #51714 ) ;
#80200=FILL_AREA_STYLE ('',( #64687 ) ) ;
#80208=EDGE_CURVE ( 'NONE', #83598, #47034, #94439, .T. ) ;
#80230=FACE_OUTER_BOUND ( 'NONE', #8344, .T. ) ;
#80241=CARTESIAN_POINT ( 'NONE',  ( 0.000000000000000000, 99.99999999999998579, 8.000000000000000000 ) ) ;
#80242=FILL_AREA_STYLE_COLOUR ( '', #62474 ) ;
#80250=COLOUR_RGB ( '', 0.72549020, 0.75294118, 0.79215686) ;
#80256=CIRCLE ( 'NONE', #49928, 0.7500000000000006661 ) ;
#80265=CARTESIAN_POINT ( 'NONE',  ( 8.879999999999991900, 76.07179676972447169, -4.250000000000000000 ) ) ;
#80281=CARTESIAN_POINT ( 'NONE',  ( -12.98310705059825310, 90.76710648773774892, -7.614994760437855170 ) ) ;
#80292=CIRCLE ( 'NONE', #78735, 6.349999999999995204 ) ;
#80299=CYLINDRICAL_SURFACE ( 'NONE', #14669, 1.249999999999987121 ) ;
#80300=FILL_AREA_STYLE_COLOUR ( '', #72319 ) ;
#80303=CIRCLE ( 'NONE', #14879, 3.250000000000002665 ) ;
#80304=ORIENTED_EDGE ( 'NONE', *, *, #47968, .F. ) ;
#80306=LINE ( 'NONE', #42314, #70001 ) ;
#80311=FACE_OUTER_BOUND ( 'NONE', #41748, .T. ) ;
#80320=ORIENTED_EDGE ( 'NONE', *, *, #17873, .T. ) ;
#80328=( GEOMETRIC_REPRESENTATION_CONTEXT ( 3 ) GLOBAL_UNCERTAINTY_ASSIGNED_CONTEXT ( ( #98298 ) ) GLOBAL_UNIT_ASSIGNED_CONTEXT ( ( #1384, #48321, #92355 ) ) REPRESENTATION_CONTEXT ( 'NONE', 'WORKASPACE' ) );
#80345=COLOUR_RGB ( '', 0.72549020, 0.75294118, 0.79215686) ;
#80350=CARTESIAN_POINT ( 'NONE',  ( -6.982525766850298687, -88.11956318484570261, -2.750000000000000444 ) ) ;
#80356=ORIENTED_EDGE ( 'NONE', *, *, #13420, .F. ) ;
#80367=CARTESIAN_POINT ( 'NONE',  ( 8.879999999999991900, 76.07179676972447169, -6.250000000000000000 ) ) ;
#80377=AXIS2_PLACEMENT_3D ( 'NONE', #15462, #54898, #37961 ) ;
#80384=CARTESIAN_POINT ( 'NONE',  ( 8.879999999999991900, 18.00000000000000355, 2.900000000000000355 ) ) ;
#80386=DIRECTION ( 'NONE',  ( 1.049065152435176504E-16, -1.000000000000000000, 0.000000000000000000 ) ) ;
#80392=EDGE_CURVE ( 'NONE', #26706, #49230, #36996, .T. ) ;
#80393=CARTESIAN_POINT ( 'NONE',  ( 6.579634127946653699, -87.99828267815715321, 2.500000000000001332 ) ) ;
#80403=COLOUR_RGB ( '', 0.40784314, 0.44705882, 0.49803922) ;
#80406=CARTESIAN_POINT ( 'NONE',  ( -3.887834249412644994, -8.254296980873727207, -2.749999999999596767 ) ) ;
#80414=EDGE_LOOP ( 'NONE', ( #69545, #22071, #1784, #57180 ) ) ;
#80417=CARTESIAN_POINT ( 'NONE',  ( 5.115475850227041654, -17.53855045868316154, -4.000000000006439294 ) ) ;
#80420=CARTESIAN_POINT ( 'NONE',  ( -7.232415441807423129, -88.12698951299773853, 4.000000000000000000 ) ) ;
#80448=EDGE_CURVE ( 'NONE', #92377, #45159, #60895, .T. ) ;
#80455=DIRECTION ( 'NONE',  ( 1.000000000000000000, 0.000000000000000000, 0.000000000000000000 ) ) ;
#80462=CARTESIAN_POINT ( 'NONE',  ( -8.000000608138725156, -0.01989113958122736350, -3.750000000000000888 ) ) ;
#80484=ORIENTED_EDGE ( 'NONE', *, *, #77918, .T. ) ;
#80489=ADVANCED_FACE ( 'NONE', ( #48809 ), #1381, .T. ) ;
#80493=CARTESIAN_POINT ( 'NONE',  ( -18.89999999999999503, 98.99999999999998579, 7.750000000000000000 ) ) ;
#80500=ORIENTED_EDGE ( 'NONE', *, *, #40282, .F. ) ;
#80502=EDGE_CURVE ( 'NONE', #28519, #36015, #17799, .T. ) ;
#80504=ADVANCED_FACE ( 'NONE', ( #11798 ), #80299, .F. ) ;
#80509=FILL_AREA_STYLE ('',( #85551 ) ) ;
#80515=ADVANCED_FACE ( 'NONE', ( #59262 ), #89763, .F. ) ;
#80525=DIRECTION ( 'NONE',  ( -1.000000000000000000, -0.000000000000000000, -0.000000000000000000 ) ) ;
#80530=CARTESIAN_POINT ( 'NONE',  ( -0.6999999999999957367, 99.99999999999998579, -8.525133428036873795 ) ) ;
#80533=CARTESIAN_POINT ( 'NONE',  ( -4.010384638568479154, -13.83464189901983232, -2.500000000000000444 ) ) ;
#80539=CARTESIAN_POINT ( 'NONE',  ( 4.469999999999999751, 10.25000000000000000, 3.750000000000000000 ) ) ;
#80540=EDGE_CURVE ( 'NONE', #6847, #26894, #35333, .T. ) ;
#80543=CARTESIAN_POINT ( 'NONE',  ( 18.00000000000000000, 78.06026162106621769, -3.869897288747938369 ) ) ;
#80544=( GEOMETRIC_REPRESENTATION_CONTEXT ( 3 ) GLOBAL_UNCERTAINTY_ASSIGNED_CONTEXT ( ( #89476 ) ) GLOBAL_UNIT_ASSIGNED_CONTEXT ( ( #86410, #94879, #33863 ) ) REPRESENTATION_CONTEXT ( 'NONE', 'WORKASPACE' ) );
#80550=FACE_OUTER_BOUND ( 'NONE', #60770, .T. ) ;
#80552=VERTEX_POINT ( 'NONE', #12290 ) ;
#80566=DIRECTION ( 'NONE',  ( 1.000000000000000000, 0.000000000000000000, -0.000000000000000000 ) ) ;
#80567=CARTESIAN_POINT ( 'NONE',  ( -3.750000000000000888, 1.019547802438453887, -4.000000000000000000 ) ) ;
#80574=CARTESIAN_POINT ( 'NONE',  ( -13.72572134032981062, 90.95701465610191860, 7.926449989681190189 ) ) ;
#80581=EDGE_CURVE ( 'NONE', #62017, #28374, #8300, .T. ) ;
#80582=VERTEX_POINT ( 'NONE', #58774 ) ;
#80584=ORIENTED_EDGE ( 'NONE', *, *, #93514, .F. ) ;
#80606=CARTESIAN_POINT ( 'NONE',  ( 18.00000000000000355, 77.07179676972445748, -4.250000000000000000 ) ) ;
#80609=DIRECTION ( 'NONE',  ( 1.000000000000000000, 2.107602052970794797E-16, -0.000000000000000000 ) ) ;
#80614=ORIENTED_EDGE ( 'NONE', *, *, #15169, .F. ) ;
#80616=STYLED_ITEM ( 'NONE', ( #70744 ), #90669 ) ;
#80619=CARTESIAN_POINT ( 'NONE',  ( -7.081429851441987999, -84.79152421822195151, 2.750000000000000000 ) ) ;
#80622=DIRECTION ( 'NONE',  ( 0.000000000000000000, 0.000000000000000000, 1.000000000000000000 ) ) ;
#80625=CARTESIAN_POINT ( 'NONE',  ( -8.000000000000000000, 79.82179676972448590, 6.250000000000000000 ) ) ;
#80627=DIRECTION ( 'NONE',  ( 0.6246950475544237324, 0.7808688094430306093, 0.000000000000000000 ) ) ;
#80631=DIRECTION ( 'NONE',  ( -1.000000000000000000, 0.000000000000000000, 0.000000000000000000 ) ) ;
#80669=CARTESIAN_POINT ( 'NONE',  ( 8.879999999999995453, 41.24999999999999289, -4.250000000000000000 ) ) ;
#80675=CARTESIAN_POINT ( 'NONE',  ( -10.44999999999999751, 99.99999999999998579, 8.000000000000000000 ) ) ;
#80689=CARTESIAN_POINT ( 'NONE',  ( 47.41185586981792000, 64.79620302208442695, -8.000000000000000000 ) ) ;
#80697=DIRECTION ( 'NONE',  ( 1.000000000000000000, -0.000000000000000000, 0.000000000000000000 ) ) ;
#80701=EDGE_CURVE ( 'NONE', #51712, #14094, #54600, .T. ) ;
#80702=EDGE_LOOP ( 'NONE', ( #59130, #31113 ) ) ;
#80721=DIRECTION ( 'NONE',  ( 1.000000000000000000, -0.000000000000000000, 0.000000000000000000 ) ) ;
#80726=VECTOR ( 'NONE', #69238, 1000.000000000000114 ) ;
#80735=DIRECTION ( 'NONE',  ( -0.1496197561345325722, 0.9887436111420609963, 0.000000000000000000 ) ) ;
#80747=MECHANICAL_DESIGN_GEOMETRIC_PRESENTATION_REPRESENTATION('',(#58394),#64734);
#80761=CARTESIAN_POINT ( 'NONE',  ( 8.879999999999995453, 41.24999999999999289, 6.500000000000000888 ) ) ;
#80767=CARTESIAN_POINT ( 'NONE',  ( -3.749999999999993783, 43.00000000000000711, -4.000000000000000000 ) ) ;
#80768=EDGE_CURVE ( 'NONE', #51986, #43714, #55742, .T. ) ;
#80772=CARTESIAN_POINT ( 'NONE',  ( -7.750000000000000000, 80.32179676972448590, 4.000000000000000000 ) ) ;
#80779=CARTESIAN_POINT ( 'NONE',  ( 18.00000000000001776, 4.625929269271493211E-15, 4.000000000000000000 ) ) ;
#80784=SURFACE_STYLE_FILL_AREA ( #35271 ) ;
#80785=FACE_OUTER_BOUND ( 'NONE', #64587, .T. ) ;
#80794=( LENGTH_UNIT ( ) NAMED_UNIT ( * ) SI_UNIT ( .MILLI., .METRE. ) );
#80796=SURFACE_SIDE_STYLE ('',( #50280 ) ) ;
#80802=DIRECTION ( 'NONE',  ( 1.000000000000000000, 0.000000000000000000, 0.000000000000000000 ) ) ;
#80820=FILL_AREA_STYLE_COLOUR ( '', #20146 ) ;
#80821=( GEOMETRIC_REPRESENTATION_CONTEXT ( 3 ) GLOBAL_UNCERTAINTY_ASSIGNED_CONTEXT ( ( #95430 ) ) GLOBAL_UNIT_ASSIGNED_CONTEXT ( ( #37427, #90893, #22421 ) ) REPRESENTATION_CONTEXT ( 'NONE', 'WORKASPACE' ) );
#80822=EDGE_LOOP ( 'NONE', ( #16462, #72809, #20828, #16353, #29394, #75672, #11087, #80484 ) ) ;
#80823=CIRCLE ( 'NONE', #92032, 0.1000000000000001166 ) ;
#80843=( GEOMETRIC_REPRESENTATION_CONTEXT ( 3 ) GLOBAL_UNCERTAINTY_ASSIGNED_CONTEXT ( ( #48448 ) ) GLOBAL_UNIT_ASSIGNED_CONTEXT ( ( #23599, #8577, #70068 ) ) REPRESENTATION_CONTEXT ( 'NONE', 'WORKASPACE' ) );
#80851=EDGE_CURVE ( 'NONE', #35385, #82533, #41728, .T. ) ;
#80880=EDGE_CURVE ( 'NONE', #98319, #55638, #51405, .T. ) ;
#80897=CARTESIAN_POINT ( 'NONE',  ( -6.871342362925322078, -73.24551516664604378, -2.500000000000000000 ) ) ;
#80903=ORIENTED_EDGE ( 'NONE', *, *, #52473, .T. ) ;
#80908=CARTESIAN_POINT ( 'NONE',  ( -7.117803565204841476, -58.38168516195395341, 3.999999999999999112 ) ) ;
#80918=( LENGTH_UNIT ( ) NAMED_UNIT ( * ) SI_UNIT ( .MILLI., .METRE. ) );
#80921=STYLED_ITEM ( 'NONE', ( #69928 ), #72720 ) ;
#80927=ORIENTED_EDGE ( 'NONE', *, *, #48537, .F. ) ;
#80944=CYLINDRICAL_SURFACE ( 'NONE', #66821, 9.999999999999998224 ) ;
#80968=CARTESIAN_POINT ( 'NONE',  ( -8.000000000000000000, 40.74999999999999289, 4.250000000000000000 ) ) ;
#80979=AXIS2_PLACEMENT_3D ( 'NONE', #17058, #33499, #11018 ) ;
#80983=ORIENTED_EDGE ( 'NONE', *, *, #80701, .F. ) ;
#80995=DIRECTION ( 'NONE',  ( 1.000000000000000000, 0.000000000000000000, 0.000000000000000000 ) ) ;
#80996=VERTEX_POINT ( 'NONE', #42699 ) ;
#81010=ORIENTED_EDGE ( 'NONE', *, *, #11287, .F. ) ;
#81018=CARTESIAN_POINT ( 'NONE',  ( -4.818654718866499209, -24.96058166501293485, -2.500000000000001776 ) ) ;
#81022=CARTESIAN_POINT ( 'NONE',  ( 3.969999999999999751, 36.75000000000000000, 2.500000000000000000 ) ) ;
#81028=CARTESIAN_POINT ( 'NONE',  ( 18.00000000000525091, 77.36262727519759608, -4.161036774751641687 ) ) ;
#81047=DIRECTION ( 'NONE',  ( 0.000000000000000000, -1.000000000000000000, 0.000000000000000000 ) ) ;
#81051=CARTESIAN_POINT ( 'NONE',  ( -10.09048698379360687, 46.92328126389585208, 0.000000000000000000 ) ) ;
#81052=TOROIDAL_SURFACE ( 'NONE', #37968, 0.5000000000000000000, 0.2500000000000000000 ) ;
#81067=DIRECTION ( 'NONE',  ( -0.000000000000000000, -0.000000000000000000, -1.000000000000000000 ) ) ;
#81070=ORIENTED_EDGE ( 'NONE', *, *, #81939, .T. ) ;
#81083=ORIENTED_EDGE ( 'NONE', *, *, #91110, .T. ) ;
#81094=ORIENTED_EDGE ( 'NONE', *, *, #39298, .T. ) ;
#81098=FACE_OUTER_BOUND ( 'NONE', #47741, .T. ) ;
#81100=CIRCLE ( 'NONE', #15689, 0.2500000000000002220 ) ;
#81101=ORIENTED_EDGE ( 'NONE', *, *, #94961, .T. ) ;
#81103=CARTESIAN_POINT ( 'NONE',  ( -8.000000000000000000, 41.24999999999999289, -6.250000000000000000 ) ) ;
#81104=CARTESIAN_POINT ( 'NONE',  ( -10.09048698379360687, 46.92328126389585208, 3.000000000000000000 ) ) ;
#81107=ORIENTED_EDGE ( 'NONE', *, *, #52473, .F. ) ;
#81116=VECTOR ( 'NONE', #97693, 1000.000000000000000 ) ;
#81117=DIRECTION ( 'NONE',  ( 0.000000000000000000, 0.000000000000000000, -1.000000000000000000 ) ) ;
#81124=DIRECTION ( 'NONE',  ( 1.000000000000000000, 0.000000000000000000, 0.000000000000000000 ) ) ;
#81125=CARTESIAN_POINT ( 'NONE',  ( -4.000000000000000000, 37.00000000000000000, -2.500000000000000000 ) ) ;
#81126=DIRECTION ( 'NONE',  ( -0.000000000000000000, -0.000000000000000000, 1.000000000000000000 ) ) ;
#81134=LINE ( 'NONE', #10679, #8077 ) ;
#81148=ORIENTED_EDGE ( 'NONE', *, *, #55529, .F. ) ;
#81160=EDGE_CURVE ( 'NONE', #19902, #54884, #35565, .T. ) ;
#81165=CARTESIAN_POINT ( 'NONE',  ( 4.221203097590866982, -3.619724449986670756, 2.500000000000000000 ) ) ;
#81169=ORIENTED_EDGE ( 'NONE', *, *, #96522, .F. ) ;
#81170=PRESENTATION_STYLE_ASSIGNMENT (( #35672 ) ) ;
#81177=CARTESIAN_POINT ( 'NONE',  ( -11.20041124669619670, -94.46430075987372277, 3.999999999999099387 ) ) ;
#81186=AXIS2_PLACEMENT_3D ( 'NONE', #3941, #64901, #95427 ) ;
#81188=EDGE_LOOP ( 'NONE', ( #74874, #42346, #84168, #93744 ) ) ;
#81189=CARTESIAN_POINT ( 'NONE',  ( 8.879999999999991900, 76.07179676972447169, 6.250000000000000000 ) ) ;
#81190=ORIENTED_EDGE ( 'NONE', *, *, #620, .T. ) ;
#81243=DIRECTION ( 'NONE',  ( -0.000000000000000000, -0.000000000000000000, 1.000000000000000000 ) ) ;
#81245=AXIS2_PLACEMENT_3D ( 'NONE', #36943, #67440, #329 ) ;
#81254=CARTESIAN_POINT ( 'NONE',  ( 4.920153426831056720, -13.81781469843442345, 3.749999999999998668 ) ) ;
#81255=( NAMED_UNIT ( * ) PLANE_ANGLE_UNIT ( ) SI_UNIT ( $, .RADIAN. ) );
#81256=EDGE_CURVE ( 'NONE', #95526, #8937, #52056, .T. ) ;
#81261=ORIENTED_EDGE ( 'NONE', *, *, #95766, .F. ) ;
#81265=DIRECTION ( 'NONE',  ( 0.000000000000000000, 0.000000000000000000, 1.000000000000000000 ) ) ;
#81266=CARTESIAN_POINT ( 'NONE',  ( 18.00000000000000000, 84.07179676972448590, -3.750000000000000000 ) ) ;
#81281=DIRECTION ( 'NONE',  ( -1.000000000000000000, -0.000000000000000000, -0.000000000000000000 ) ) ;
#81287=UNCERTAINTY_MEASURE_WITH_UNIT (LENGTH_MEASURE( 1.000000000000000082E-05 ), #85310, 'distance_accuracy_value', 'NONE');
#81295=CYLINDRICAL_SURFACE ( 'NONE', #77362, 10.90000000000026326 ) ;
#81301=DIRECTION ( 'NONE',  ( 0.000000000000000000, 0.000000000000000000, 1.000000000000000000 ) ) ;
#81314=ORIENTED_EDGE ( 'NONE', *, *, #58243, .T. ) ;
#81315=CARTESIAN_POINT ( 'NONE',  ( -4.000000000000000000, 36.75000000000000000, -2.500000000000000000 ) ) ;
#81323=ORIENTED_EDGE ( 'NONE', *, *, #70402, .T. ) ;
#81341=CIRCLE ( 'NONE', #38259, 0.2500000000000002220 ) ;
#81351=CARTESIAN_POINT ( 'NONE',  ( 17.75000000000000355, 78.80384757729335377, -4.000000000000000000 ) ) ;
#81353=ORIENTED_EDGE ( 'NONE', *, *, #22063, .T. ) ;
#81362=CARTESIAN_POINT ( 'NONE',  ( -8.448386164854104763, 87.04264023965325237, -4.560422061235506419 ) ) ;
#81366=SPHERICAL_SURFACE ( 'NONE', #19070, 0.2500000000000000000 ) ;
#81371=EDGE_LOOP ( 'NONE', ( #29769, #33599, #41031, #26022 ) ) ;
#81373=AXIS2_PLACEMENT_3D ( 'NONE', #46836, #17348, #71808 ) ;
#81376=CARTESIAN_POINT ( 'NONE',  ( 3.969999999999999751, 10.25000000000000000, 2.500000000000000000 ) ) ;
#81378=CARTESIAN_POINT ( 'NONE',  ( -8.448386164854106539, 87.04264023965323815, 4.560422061235506419 ) ) ;
#81388=LINE ( 'NONE', #18931, #73970 ) ;
#81392=CARTESIAN_POINT ( 'NONE',  ( -3.750000000000000888, 0.08806741915676698229, 4.000000000000000000 ) ) ;
#81402=( NAMED_UNIT ( * ) SI_UNIT ( $, .STERADIAN. ) SOLID_ANGLE_UNIT ( ) );
#81410=EDGE_LOOP ( 'NONE', ( #52271, #32259, #46476, #63826 ) ) ;
#81411=CARTESIAN_POINT ( 'NONE',  ( -6.982525766850296911, -88.11956318484570261, -3.750000000000000000 ) ) ;
#81420=EDGE_LOOP ( 'NONE', ( #30908, #75510, #31001, #70467, #62497 ) ) ;
#81428=( NAMED_UNIT ( * ) SI_UNIT ( $, .STERADIAN. ) SOLID_ANGLE_UNIT ( ) );
#81450=EDGE_CURVE ( 'NONE', #2391, #80552, #91292, .T. ) ;
#81462=CARTESIAN_POINT ( 'NONE',  ( -6.829922651553562929, -69.52824172495176924, 2.500000000000000000 ) ) ;
#81464=DIRECTION ( 'NONE',  ( 0.6246950475544238435, 0.7808688094430307203, 0.000000000000000000 ) ) ;
#81469=CARTESIAN_POINT ( 'NONE',  ( 5.365133693937635506, -17.52547282955412200, 4.000000000000000000 ) ) ;
#81481=DIRECTION ( 'NONE',  ( 1.000000000000000000, 0.000000000000000000, 0.000000000000000000 ) ) ;
#81509=FILL_AREA_STYLE ('',( #5534 ) ) ;
#81510=EDGE_LOOP ( 'NONE', ( #1256, #57199, #72651, #51766 ) ) ;
#81542=FACE_OUTER_BOUND ( 'NONE', #86996, .T. ) ;
#81555=DIRECTION ( 'NONE',  ( 1.000000000000000000, 0.000000000000000000, 0.000000000000000000 ) ) ;
#81557=VERTEX_POINT ( 'NONE', #30523 ) ;
#81577=CARTESIAN_POINT ( 'NONE',  ( 0.000000000000000000, -97.00000000000000000, 2.500000000000000000 ) ) ;
#81585=CARTESIAN_POINT ( 'NONE',  ( -8.000000000000000000, 0.000000000000000000, 3.750000000000000000 ) ) ;
#81589=DIRECTION ( 'NONE',  ( -1.000000000000000000, 0.000000000000000000, 0.000000000000000000 ) ) ;
#81590=CARTESIAN_POINT ( 'NONE',  ( -10.77730536144846596, -98.63085534186639336, 3.750000000000000000 ) ) ;
#81594=LINE ( 'NONE', #20113, #25654 ) ;
#81605=EDGE_CURVE ( 'NONE', #58305, #86598, #65875, .T. ) ;
#81614=DIRECTION ( 'NONE',  ( -0.000000000000000000, 0.000000000000000000, 1.000000000000000000 ) ) ;
#81621=CARTESIAN_POINT ( 'NONE',  ( -10.77974636317328994, -96.52223143591398014, -4.000000000000000000 ) ) ;
#81622=AXIS2_PLACEMENT_3D ( 'NONE', #87078, #64551, #80566 ) ;
#81625=CARTESIAN_POINT ( 'NONE',  ( -7.199999999999997513, 99.99999999999998579, -8.000000000000000000 ) ) ;
#81626=PRESENTATION_STYLE_ASSIGNMENT (( #88636 ) ) ;
#81638=EDGE_CURVE ( 'NONE', #93468, #27652, #57957, .T. ) ;
#81653=SURFACE_STYLE_FILL_AREA ( #43660 ) ;
#81665=DIRECTION ( 'NONE',  ( -0.000000000000000000, 0.000000000000000000, 1.000000000000000000 ) ) ;
#81684=ORIENTED_EDGE ( 'NONE', *, *, #13324, .F. ) ;
#81686=ORIENTED_EDGE ( 'NONE', *, *, #76753, .F. ) ;
#81693=DIRECTION ( 'NONE',  ( 0.6246950475544237324, 0.7808688094430306093, 0.000000000000000000 ) ) ;
#81713=ADVANCED_FACE ( 'NONE', ( #35950 ), #59436, .T. ) ;
#81718=CARTESIAN_POINT ( 'NONE',  ( -13.86076281203281546, 90.90669854496245250, 7.842019570309374465 ) ) ;
#81722=ORIENTED_EDGE ( 'NONE', *, *, #88300, .T. ) ;
#81733=DIRECTION ( 'NONE',  ( 0.000000000000000000, 0.000000000000000000, 1.000000000000000000 ) ) ;
#81742=ORIENTED_EDGE ( 'NONE', *, *, #59560, .T. ) ;
#81747=( LENGTH_UNIT ( ) NAMED_UNIT ( * ) SI_UNIT ( .MILLI., .METRE. ) );
#81748=TOROIDAL_SURFACE ( 'NONE', #64194, 2.750000000000001776, 0.2500000000000000000 ) ;
#81755=( GEOMETRIC_REPRESENTATION_CONTEXT ( 3 ) GLOBAL_UNCERTAINTY_ASSIGNED_CONTEXT ( ( #65481 ) ) GLOBAL_UNIT_ASSIGNED_CONTEXT ( ( #35171, #21676, #35679 ) ) REPRESENTATION_CONTEXT ( 'NONE', 'WORKASPACE' ) );
#81782=CARTESIAN_POINT ( 'NONE',  ( 4.191187596054804843, -2.692365941978121846, -2.500000000000000444 ) ) ;
#81785=ORIENTED_EDGE ( 'NONE', *, *, #41137, .T. ) ;
#81788=VERTEX_POINT ( 'NONE', #51952 ) ;
#81808=FACE_OUTER_BOUND ( 'NONE', #22194, .T. ) ;
#81819=CIRCLE ( 'NONE', #16323, 0.2500000000000002220 ) ;
#81822=DIRECTION ( 'NONE',  ( -0.000000000000000000, 1.000000000000000000, 0.000000000000000000 ) ) ;
#81836=( NAMED_UNIT ( * ) PLANE_ANGLE_UNIT ( ) SI_UNIT ( $, .RADIAN. ) );
#81840=FILL_AREA_STYLE_COLOUR ( '', #29701 ) ;
#81844=ORIENTED_EDGE ( 'NONE', *, *, #26485, .F. ) ;
#81847=CARTESIAN_POINT ( 'NONE',  ( -7.984789763142468466, 85.83064272735663280, -4.183481735294423132 ) ) ;
#81849=VECTOR ( 'NONE', #29671, 1000.000000000000000 ) ;
#81862=AXIS2_PLACEMENT_3D ( 'NONE', #12719, #95737, #89211 ) ;
#81864=CARTESIAN_POINT ( 'NONE',  ( 4.130000000000002558, 1.019547802438464545, -2.750000000000000000 ) ) ;
#81876=CYLINDRICAL_SURFACE ( 'NONE', #26100, 0.2500000000000002220 ) ;
#81883=CYLINDRICAL_SURFACE ( 'NONE', #46245, 0.09999999999999982514 ) ;
#81908=ORIENTED_EDGE ( 'NONE', *, *, #61660, .F. ) ;
#81913=LINE ( 'NONE', #72934, #34478 ) ;
#81918=SURFACE_STYLE_USAGE ( .BOTH. , #96456 ) ;
#81919=SURFACE_STYLE_USAGE ( .BOTH. , #6923 ) ;
#81929=VERTEX_POINT ( 'NONE', #69410 ) ;
#81938=AXIS2_PLACEMENT_3D ( 'NONE', #95416, #33901, #10444 ) ;
#81939=EDGE_CURVE ( 'NONE', #80099, #38899, #85398, .T. ) ;
#81957=CARTESIAN_POINT ( 'NONE',  ( 10.09974179609097611, -32.02510747890637077, 4.000000000000000000 ) ) ;
#81978=ORIENTED_EDGE ( 'NONE', *, *, #3169, .T. ) ;
#81980=AXIS2_PLACEMENT_3D ( 'NONE', #55785, #11748, #57728 ) ;
#81994=CARTESIAN_POINT ( 'NONE',  ( 9.780380530190813104, 27.00871557427475977, -3.000000000000000000 ) ) ;
#82021=VERTEX_POINT ( 'NONE', #83432 ) ;
#82034=CARTESIAN_POINT ( 'NONE',  ( 10.95627140743379613, -96.88013104273433385, -3.750000000000000888 ) ) ;
#82041=AXIS2_PLACEMENT_3D ( 'NONE', #92732, #54720, #48209 ) ;
#82052=ORIENTED_EDGE ( 'NONE', *, *, #72291, .T. ) ;
#82078=ORIENTED_EDGE ( 'NONE', *, *, #63780, .F. ) ;
#82081=ORIENTED_EDGE ( 'NONE', *, *, #21122, .T. ) ;
#82083=CARTESIAN_POINT ( 'NONE',  ( 6.880000000000009663, 41.24999999999999289, 6.500000000000000888 ) ) ;
#82088=CARTESIAN_POINT ( 'NONE',  ( -7.124967611315338623, -78.82395889337750816, 3.750000000000000888 ) ) ;
#82092=EDGE_LOOP ( 'NONE', ( #57492, #45280, #67302, #70770, #80179, #54320, #83064, #75075, #39324, #2845 ) ) ;
#82095=CARTESIAN_POINT ( 'NONE',  ( 8.880000000000000782, 1.019547802438459216, -3.750000000000001776 ) ) ;
#82098=CYLINDRICAL_SURFACE ( 'NONE', #60138, 0.2500000000000002220 ) ;
#82100=FACE_OUTER_BOUND ( 'NONE', #71587, .T. ) ;
#82102=VERTEX_POINT ( 'NONE', #92401 ) ;
#82108=( NAMED_UNIT ( * ) SI_UNIT ( $, .STERADIAN. ) SOLID_ANGLE_UNIT ( ) );
#82112=DIRECTION ( 'NONE',  ( -1.000000000000000000, 0.000000000000000000, 0.000000000000000000 ) ) ;
#82127=UNCERTAINTY_MEASURE_WITH_UNIT (LENGTH_MEASURE( 1.000000000000000082E-05 ), #2504, 'distance_accuracy_value', 'NONE');
#82141=CARTESIAN_POINT ( 'NONE',  ( 18.00000000000000355, 77.07179676972445748, 6.250000000000000000 ) ) ;
#82148=( NAMED_UNIT ( * ) SI_UNIT ( $, .STERADIAN. ) SOLID_ANGLE_UNIT ( ) );
#82155=CARTESIAN_POINT ( 'NONE',  ( -11.07542066904767175, -96.02453755659226431, 4.000000000000452971 ) ) ;
#82185=EDGE_LOOP ( 'NONE', ( #39013, #97243, #58917, #25857, #48071, #90801, #80108, #8581 ) ) ;
#82196=ORIENTED_EDGE ( 'NONE', *, *, #41262, .T. ) ;
#82199=CARTESIAN_POINT ( 'NONE',  ( -3.750000000000000000, 10.25000000000000000, 3.750000000000000000 ) ) ;
#82206=ORIENTED_EDGE ( 'NONE', *, *, #4098, .T. ) ;
#82214=DIRECTION ( 'NONE',  ( -0.8073289077885722476, 0.5901017155109032908, -1.999617224239539632E-13 ) ) ;
#82215=CIRCLE ( 'NONE', #72578, 1.750000000000000666 ) ;
#82237=FACE_OUTER_BOUND ( 'NONE', #78234, .T. ) ;
#82242=ORIENTED_EDGE ( 'NONE', *, *, #40332, .T. ) ;
#82250=ORIENTED_EDGE ( 'NONE', *, *, #93444, .F. ) ;
#82252=CARTESIAN_POINT ( 'NONE',  ( 11.04808542137200966, -95.57857389789997171, -4.000000000000000000 ) ) ;
#82268=CIRCLE ( 'NONE', #85500, 0.2500000000000002220 ) ;
#82279=CARTESIAN_POINT ( 'NONE',  ( 5.783708210295563923, -36.05554043934295549, -2.500000000000000444 ) ) ;
#82284=ORIENTED_EDGE ( 'NONE', *, *, #54646, .F. ) ;
#82286=VERTEX_POINT ( 'NONE', #32875 ) ;
#82289=ORIENTED_EDGE ( 'NONE', *, *, #21078, .F. ) ;
#82298=ORIENTED_EDGE ( 'NONE', *, *, #37815, .T. ) ;
#82326=SURFACE_STYLE_USAGE ( .BOTH. , #44817 ) ;
#82330=ORIENTED_EDGE ( 'NONE', *, *, #50053, .F. ) ;
#82335=AXIS2_PLACEMENT_3D ( 'NONE', #93673, #2708, #24213 ) ;
#82343=CARTESIAN_POINT ( 'NONE',  ( -7.804338076140435732, 84.96756567522902515, -4.038273117401846690 ) ) ;
#82369=CARTESIAN_POINT ( 'NONE',  ( 3.969999999999999751, 36.75000000000000000, -2.500000000000000000 ) ) ;
#82376=CARTESIAN_POINT ( 'NONE',  ( 8.979999999999991545, 27.04366094290857347, -3.000000000000000000 ) ) ;
#82386=AXIS2_PLACEMENT_3D ( 'NONE', #76158, #91655, #19824 ) ;
#82428=( NAMED_UNIT ( * ) PLANE_ANGLE_UNIT ( ) SI_UNIT ( $, .RADIAN. ) );
#82450=CARTESIAN_POINT ( 'NONE',  ( -7.116252256160142231, -80.68108970088715637, 2.749999999999193978 ) ) ;
#82454=CARTESIAN_POINT ( 'NONE',  ( 11.44533298127016074, -77.48611261198149691, 4.000000000000000000 ) ) ;
#82458=MECHANICAL_DESIGN_GEOMETRIC_PRESENTATION_REPRESENTATION('',(#28140),#61677);
#82463=AXIS2_PLACEMENT_3D ( 'NONE', #19115, #50601, #73581 ) ;
#82478=VECTOR ( 'NONE', #19817, 1000.000000000000000 ) ;
#82482=FILL_AREA_STYLE ('',( #96019 ) ) ;
#82486=AXIS2_PLACEMENT_3D ( 'NONE', #78398, #26870, #64852 ) ;
#82504=CARTESIAN_POINT ( 'NONE',  ( -0.5000000000000073275, 80.99999999999994316, -1.249999999999987121 ) ) ;
#82506=AXIS2_PLACEMENT_3D ( 'NONE', #95681, #42676, #27167 ) ;
#82517=DIRECTION ( 'NONE',  ( 1.000000000000000000, -0.000000000000000000, 0.000000000000000000 ) ) ;
#82531=CARTESIAN_POINT ( 'NONE',  ( -6.868018881919620178, -58.39307134327821558, -3.999999999999999556 ) ) ;
#82532=ORIENTED_EDGE ( 'NONE', *, *, #26313, .T. ) ;
#82533=VERTEX_POINT ( 'NONE', #27344 ) ;
#82546=EDGE_CURVE ( 'NONE', #22102, #45519, #35836, .T. ) ;
#82551=ORIENTED_EDGE ( 'NONE', *, *, #91077, .T. ) ;
#82553=CYLINDRICAL_SURFACE ( 'NONE', #9466, 2.999999999999997780 ) ;
#82560=CARTESIAN_POINT ( 'NONE',  ( -15.00000000000004974, 91.25000000000000000, -8.000000000000000000 ) ) ;
#82578=CARTESIAN_POINT ( 'NONE',  ( 10.95672398092087718, -56.81605919574143826, 4.000000000000000888 ) ) ;
#82585=ORIENTED_EDGE ( 'NONE', *, *, #79818, .F. ) ;
#82596=CARTESIAN_POINT ( 'NONE',  ( -4.000000000000000000, 10.00000000000000000, 2.500000000000000000 ) ) ;
#82599=CARTESIAN_POINT ( 'NONE',  ( -0.5000000000000073275, 80.99999999999994316, 1.249999999999987121 ) ) ;
#82607=CARTESIAN_POINT ( 'NONE',  ( -3.635384400432159158, -3.854802480546752896, -2.750000000000000444 ) ) ;
#82611=VECTOR ( 'NONE', #16765, 1000.000000000000000 ) ;
#82619=CARTESIAN_POINT ( 'NONE',  ( -3.750000000000000000, 10.25000000000000000, 2.500000000000000000 ) ) ;
#82620=EDGE_CURVE ( 'NONE', #49181, #60398, #10022, .T. ) ;
#82624=AXIS2_PLACEMENT_3D ( 'NONE', #64311, #81301, #35300 ) ;
#82634=( NAMED_UNIT ( * ) PLANE_ANGLE_UNIT ( ) SI_UNIT ( $, .RADIAN. ) );
#82647=ORIENTED_EDGE ( 'NONE', *, *, #5766, .T. ) ;
#82655=FILL_AREA_STYLE_COLOUR ( '', #62624 ) ;
#82676=AXIS2_PLACEMENT_3D ( 'NONE', #9222, #93202, #61716 ) ;
#82681=ORIENTED_EDGE ( 'NONE', *, *, #76164, .F. ) ;
#82685=COLOUR_RGB ( '', 0.08235294, 0.09019608, 0.10196078) ;
#82686=EDGE_CURVE ( 'NONE', #37189, #28474, #78750, .T. ) ;
#82692=EDGE_CURVE ( 'NONE', #92445, #12912, #38785, .T. ) ;
#82697=CARTESIAN_POINT ( 'NONE',  ( -9.000000000000000000, 75.76920769491746910, -2.900000000000000799 ) ) ;
#82702=ORIENTED_EDGE ( 'NONE', *, *, #8576, .T. ) ;
#82719=DIRECTION ( 'NONE',  ( 0.000000000000000000, 0.000000000000000000, -1.000000000000000000 ) ) ;
#82723=SURFACE_STYLE_FILL_AREA ( #36744 ) ;
#82735=( LENGTH_UNIT ( ) NAMED_UNIT ( * ) SI_UNIT ( .MILLI., .METRE. ) );
#82757=CIRCLE ( 'NONE', #6100, 7.000000000000002665 ) ;
#82763=PRESENTATION_STYLE_ASSIGNMENT (( #52267 ) ) ;
#82767=CIRCLE ( 'NONE', #84352, 0.2500000000000002220 ) ;
#82772=EDGE_CURVE ( 'NONE', #87018, #28474, #43332, .T. ) ;
#82782=DIRECTION ( 'NONE',  ( 1.000000000000000000, 1.850371707708593182E-14, 0.000000000000000000 ) ) ;
#82789=VERTEX_POINT ( 'NONE', #823 ) ;
#82799=ORIENTED_EDGE ( 'NONE', *, *, #21393, .T. ) ;
#82800=ORIENTED_EDGE ( 'NONE', *, *, #29295, .T. ) ;
#82808=COLOUR_RGB ( '', 0.08235294, 0.09019608, 0.10196078) ;
#82816=COLOUR_RGB ( '', 0.66274510, 0.83137255, 0.94901961) ;
#82820=SURFACE_STYLE_USAGE ( .BOTH. , #22341 ) ;
#82824=FACE_OUTER_BOUND ( 'NONE', #3882, .T. ) ;
#82835=CARTESIAN_POINT ( 'NONE',  ( 4.406185888753203272, -8.255243720366360449, -2.499999999999999112 ) ) ;
#82856=CARTESIAN_POINT ( 'NONE',  ( 9.879999999999990123, 20.99999999999999645, -1.249999999999987121 ) ) ;
#82859=DIRECTION ( 'NONE',  ( -0.9995586998285019842, -0.02970531260826359682, 0.000000000000000000 ) ) ;
#82868=CARTESIAN_POINT ( 'NONE',  ( -6.829922651553562929, -69.52824172495176924, -2.500000000000000000 ) ) ;
#82869=DIRECTION ( 'NONE',  ( 0.000000000000000000, 0.000000000000000000, 1.000000000000000000 ) ) ;
#82876=DIRECTION ( 'NONE',  ( -0.000000000000000000, -0.000000000000000000, 1.000000000000000000 ) ) ;
#82914=CARTESIAN_POINT ( 'NONE',  ( 4.920853330210497312, -13.83152733635706433, 3.750000000000804690 ) ) ;
#82915=DIRECTION ( 'NONE',  ( 0.6246950475544238435, 0.7808688094430307203, 0.000000000000000000 ) ) ;
#82934=CIRCLE ( 'NONE', #95714, 1.249999999999987121 ) ;
#82935=( BOUNDED_SURFACE ( )  B_SPLINE_SURFACE ( 3, 2, ( 
 ( #39475, #9953, #2962 ),
 ( #40459, #17945, #46951 ),
 ( #78933, #61461, #85454 ),
 ( #69471, #23497, #1484 ),
 ( #31937, #62438, #4431 ),
 ( #63912, #49409, #94913 ),
 ( #3441, #73885, #79910 ),
 ( #57891, #79433, #35394 ),
 ( #96415, #80417, #33899 ),
 ( #87414, #88406, #57407 ),
 ( #71920, #42905, #19414 ),
 ( #27399, #11418, #49905 ),
 ( #34897, #34399, #41940 ),
 ( #65886, #11915, #64406 ),
 ( #3929, #72402, #64887 ),
 ( #95415, #27890, #12890 ),
 ( #26910, #26412, #19904 ),
 ( #87898, #58378, #56913 ) ),
 .UNSPECIFIED., .F., .F., .F. ) 
 B_SPLINE_SURFACE_WITH_KNOTS ( ( 4, 2, 2, 2, 2, 2, 2, 2, 4 ),
 ( 3, 3 ),
 ( 0.000000000000000000, 0.002783952809522130881, 0.005567905619044261761, 0.01113581123808852352, 0.02227162247617704705, 0.04454324495235409409, 0.06681486742853114114, 0.07795067866661967160, 0.08908648990470818818 ),
 ( 0.000000000000000000, 1.000000000000000000 ),
 .UNSPECIFIED. ) 
 GEOMETRIC_REPRESENTATION_ITEM ( )  RATIONAL_B_SPLINE_SURFACE ( (
 ( 1.000000000000000000, 0.7071067811865475727, 1.000000000000000000),
 ( 1.000000000000000000, 0.7071067811865475727, 1.000000000000000000),
 ( 1.000000000000000000, 0.7071067811865475727, 1.000000000000000000),
 ( 1.000000000000000000, 0.7071067811865475727, 1.000000000000000000),
 ( 1.000000000000000000, 0.7071067811865475727, 1.000000000000000000),
 ( 1.000000000000000000, 0.7071067811865475727, 1.000000000000000000),
 ( 1.000000000000000000, 0.7071067811865475727, 1.000000000000000000),
 ( 1.000000000000000000, 0.7071067811865475727, 1.000000000000000000),
 ( 1.000000000000000000, 0.7071067811865475727, 1.000000000000000000),
 ( 1.000000000000000000, 0.7071067811865475727, 1.000000000000000000),
 ( 1.000000000000000000, 0.7071067811865487940, 1.000000000000000000),
 ( 1.000000000000000000, 0.7071067811865487940, 1.000000000000000000),
 ( 1.000000000000000000, 0.7071067811865487940, 1.000000000000000000),
 ( 1.000000000000000000, 0.7071067811865487940, 1.000000000000000000),
 ( 1.000000000000000000, 0.7071067811865475727, 1.000000000000000000),
 ( 1.000000000000000000, 0.7071067811865475727, 1.000000000000000000),
 ( 1.000000000000000000, 0.7071067811865479058, 1.000000000000000000),
 ( 1.000000000000000000, 0.7071067811865479058, 1.000000000000000000) ) ) 
 REPRESENTATION_ITEM ( '' )  SURFACE ( )  );
#82937=ORIENTED_EDGE ( 'NONE', *, *, #31500, .T. ) ;
#82942=ORIENTED_EDGE ( 'NONE', *, *, #27556, .T. ) ;
#82943=AXIS2_PLACEMENT_3D ( 'NONE', #44959, #62415, #83953 ) ;
#82950=VECTOR ( 'NONE', #32321, 1000.000000000000000 ) ;
#82972=ADVANCED_FACE ( 'NONE', ( #15332 ), #92290, .T. ) ;
#82988=EDGE_CURVE ( 'NONE', #92281, #16383, #53803, .T. ) ;
#82993=DIRECTION ( 'NONE',  ( 0.000000000000000000, 0.000000000000000000, -1.000000000000000000 ) ) ;
#83004=CIRCLE ( 'NONE', #15988, 2.750000000000000888 ) ;
#83006=AXIS2_PLACEMENT_3D ( 'NONE', #60878, #29388, #39748 ) ;
#83018=DIRECTION ( 'NONE',  ( -1.000000000000000000, 0.000000000000000000, 0.000000000000000000 ) ) ;
#83031=EDGE_CURVE ( 'NONE', #32731, #9920, #16792, .T. ) ;
#83032=CARTESIAN_POINT ( 'NONE',  ( -5.331138373814036768, -28.69357394139028017, -3.750000000000000000 ) ) ;
#83040=CARTESIAN_POINT ( 'NONE',  ( -11.22722615951306935, 89.90850287678604502, -6.380836486324904300 ) ) ;
#83049=ORIENTED_EDGE ( 'NONE', *, *, #21121, .F. ) ;
#83050=FACE_OUTER_BOUND ( 'NONE', #27722, .T. ) ;
#83051=EDGE_LOOP ( 'NONE', ( #30691, #73761, #76169, #75546 ) ) ;
#83064=ORIENTED_EDGE ( 'NONE', *, *, #5536, .T. ) ;
#83072=LINE ( 'NONE', #75570, #17181 ) ;
#83075=ORIENTED_EDGE ( 'NONE', *, *, #32433, .T. ) ;
#83085=ORIENTED_EDGE ( 'NONE', *, *, #58588, .F. ) ;
#83093=( NAMED_UNIT ( * ) PLANE_ANGLE_UNIT ( ) SI_UNIT ( $, .RADIAN. ) );
#83117=( GEOMETRIC_REPRESENTATION_CONTEXT ( 3 ) GLOBAL_UNCERTAINTY_ASSIGNED_CONTEXT ( ( #23273 ) ) GLOBAL_UNIT_ASSIGNED_CONTEXT ( ( #6774, #29750, #45257 ) ) REPRESENTATION_CONTEXT ( 'NONE', 'WORKASPACE' ) );
#83150=CARTESIAN_POINT ( 'NONE',  ( -7.750000000000000000, 1.019547802438466100, 4.000000000000000000 ) ) ;
#83156=( LENGTH_UNIT ( ) NAMED_UNIT ( * ) SI_UNIT ( .MILLI., .METRE. ) );
#83160=EDGE_LOOP ( 'NONE', ( #96169, #69694, #35146, #40214 ) ) ;
#83165=DIRECTION ( 'NONE',  ( 1.000000000000000000, 0.000000000000000000, 0.000000000000000000 ) ) ;
#83173=AXIS2_PLACEMENT_3D ( 'NONE', #48149, #3161, #47669 ) ;
#83175=ORIENTED_EDGE ( 'NONE', *, *, #21271, .F. ) ;
#83184=DIRECTION ( 'NONE',  ( -0.000000000000000000, 1.000000000000000000, -0.000000000000000000 ) ) ;
#83187=( GEOMETRIC_REPRESENTATION_CONTEXT ( 3 ) GLOBAL_UNCERTAINTY_ASSIGNED_CONTEXT ( ( #34415 ) ) GLOBAL_UNIT_ASSIGNED_CONTEXT ( ( #44707, #65723, #98235 ) ) REPRESENTATION_CONTEXT ( 'NONE', 'WORKASPACE' ) );
#83210=CARTESIAN_POINT ( 'NONE',  ( -19.00000000000000000, 75.76920769491739804, -2.900000000000000799 ) ) ;
#83235=AXIS2_PLACEMENT_3D ( 'NONE', #56424, #87881, #49393 ) ;
#83238=CARTESIAN_POINT ( 'NONE',  ( -10.77730536144846596, -98.63085534186639336, -3.750000000000000000 ) ) ;
#83253=CARTESIAN_POINT ( 'NONE',  ( 10.58840669699852199, -98.14374106289703548, -4.000000000000000000 ) ) ;
#83264=EDGE_CURVE ( 'NONE', #40405, #14972, #54765, .T. ) ;
#83266=UNCERTAINTY_MEASURE_WITH_UNIT (LENGTH_MEASURE( 1.000000000000000082E-05 ), #85236, 'distance_accuracy_value', 'NONE');
#83280=DIRECTION ( 'NONE',  ( 1.257402221000611116E-16, -1.000000000000000000, 0.000000000000000000 ) ) ;
#83285=VECTOR ( 'NONE', #75637, 1000.000000000000000 ) ;
#83298=ORIENTED_EDGE ( 'NONE', *, *, #21152, .F. ) ;
#83305=COLOUR_RGB ( '', 0.72549020, 0.75294118, 0.79215686) ;
#83308=COLOUR_RGB ( '', 0.31764706, 0.68627451, 0.89019608) ;
#83316=CARTESIAN_POINT ( 'NONE',  ( -7.199999999999996625, 99.99999999999998579, -8.525133428036873795 ) ) ;
#83322=( LENGTH_UNIT ( ) NAMED_UNIT ( * ) SI_UNIT ( .MILLI., .METRE. ) );
#83334=CARTESIAN_POINT ( 'NONE',  ( 4.655929185140254667, -8.243906417133416653, -2.499999999999999112 ) ) ;
#83337=EDGE_LOOP ( 'NONE', ( #5207, #15669, #14470, #7729 ) ) ;
#83346=CARTESIAN_POINT ( 'NONE',  ( -9.990730578767625047, 46.91630561652144138, 0.000000000000000000 ) ) ;
#83347=COLOUR_RGB ( '', 0.66274510, 0.83137255, 0.94901961) ;
#83353=CARTESIAN_POINT ( 'NONE',  ( -3.949999999999997069, 99.99999999999998579, 8.000000000000000000 ) ) ;
#83385=UNCERTAINTY_MEASURE_WITH_UNIT (LENGTH_MEASURE( 1.000000000000000082E-05 ), #5455, 'distance_accuracy_value', 'NONE');
#83394=DIRECTION ( 'NONE',  ( 0.8070303256584299145, -0.5905099943842175847, 0.000000000000000000 ) ) ;
#83398=ADVANCED_FACE ( 'NONE', ( #80230 ), #28211, .F. ) ;
#83405=CARTESIAN_POINT ( 'NONE',  ( -5.999999999999994671, 43.00000000000000000, -4.250000000000000000 ) ) ;
#83410=CARTESIAN_POINT ( 'NONE',  ( 6.575338752097509065, -50.90849809615561838, 3.999999999999999556 ) ) ;
#83419=EDGE_LOOP ( 'NONE', ( #41335, #27084, #52043, #59847 ) ) ;
#83432=CARTESIAN_POINT ( 'NONE',  ( -13.11254139118232231, 91.00000000000000000, 8.000000000000000000 ) ) ;
#83434=ORIENTED_EDGE ( 'NONE', *, *, #75522, .F. ) ;
#83438=LINE ( 'NONE', #51457, #31372 ) ;
#83448=CARTESIAN_POINT ( 'NONE',  ( 4.630000000000002558, 0.09071050906739661079, -4.000000000000000000 ) ) ;
#83457=CARTESIAN_POINT ( 'NONE',  ( -10.91371419741111204, 89.69638457836138912, 6.151049038645131084 ) ) ;
#83465=CARTESIAN_POINT ( 'NONE',  ( 6.004190426492125532, -34.81345361117713111, -2.750000000000000000 ) ) ;
#83483=DIRECTION ( 'NONE',  ( -0.000000000000000000, -1.000000000000000000, -0.000000000000000000 ) ) ;
#83501=ORIENTED_EDGE ( 'NONE', *, *, #90416, .F. ) ;
#83503=ADVANCED_FACE ( 'NONE', ( #88714 ), #5238, .T. ) ;
#83520=DIRECTION ( 'NONE',  ( 0.000000000000000000, 1.000000000000000000, -0.000000000000000000 ) ) ;
#83527=CARTESIAN_POINT ( 'NONE',  ( -7.330124059959834071, -69.53998168068577002, -3.999999999999999112 ) ) ;
#83528=ORIENTED_EDGE ( 'NONE', *, *, #56902, .T. ) ;
#83544=ORIENTED_EDGE ( 'NONE', *, *, #34284, .T. ) ;
#83552=CARTESIAN_POINT ( 'NONE',  ( 3.969999999999999751, 10.00000000000000000, -2.750000000000000000 ) ) ;
#83555=ADVANCED_FACE ( 'NONE', ( #58710 ), #88296, .T. ) ;
#83563=PLANE ( 'NONE',  #62284 ) ;
#83564=AXIS2_PLACEMENT_3D ( 'NONE', #85086, #39599, #94058 ) ;
#83573=CARTESIAN_POINT ( 'NONE',  ( 10.93144397355366770, -92.98246991212813839, 4.000000000000000000 ) ) ;
#83578=EDGE_CURVE ( 'NONE', #48651, #91690, #74704, .T. ) ;
#83581=DIRECTION ( 'NONE',  ( 0.6246950475544238435, 0.7808688094430307203, 0.000000000000000000 ) ) ;
#83586=EDGE_LOOP ( 'NONE', ( #39033, #77481, #22197, #50713 ) ) ;
#83593=DIRECTION ( 'NONE',  ( 0.000000000000000000, 0.000000000000000000, -1.000000000000000000 ) ) ;
#83597=VECTOR ( 'NONE', #95876, 1000.000000000000000 ) ;
#83598=VERTEX_POINT ( 'NONE', #4248 ) ;
#83606=CARTESIAN_POINT ( 'NONE',  ( -6.000000000000000000, 78.07179676972447169, 4.250000000000000000 ) ) ;
#83614=DIRECTION ( 'NONE',  ( 0.000000000000000000, 0.000000000000000000, -1.000000000000000000 ) ) ;
#83618=DIRECTION ( 'NONE',  ( 0.000000000000000000, 1.000000000000000000, 0.000000000000000000 ) ) ;
#83630=VECTOR ( 'NONE', #85934, 1000.000000000000000 ) ;
#83639=EDGE_CURVE ( 'NONE', #76841, #27600, #61177, .T. ) ;
#83649=CARTESIAN_POINT ( 'NONE',  ( -11.16005593731603618, -52.90553718811315775, 3.750000000000000000 ) ) ;
#83663=CYLINDRICAL_SURFACE ( 'NONE', #21742, 0.2500000000000002220 ) ;
#83668=FACE_OUTER_BOUND ( 'NONE', #78741, .T. ) ;
#83673=EDGE_CURVE ( 'NONE', #36015, #69849, #46186, .T. ) ;
#83683=DIRECTION ( 'NONE',  ( 0.000000000000000000, 1.000000000000000000, 0.000000000000000000 ) ) ;
#83688=CARTESIAN_POINT ( 'NONE',  ( 3.969999999999999751, 10.25000000000000000, -4.000000000000000000 ) ) ;
#83696=AXIS2_PLACEMENT_3D ( 'NONE', #44725, #53218, #8221 ) ;
#83697=DIRECTION ( 'NONE',  ( 0.000000000000000000, 0.000000000000000000, 1.000000000000000000 ) ) ;
#83720=LINE ( 'NONE', #6734, #29365 ) ;
#83730=DIRECTION ( 'NONE',  ( 0.8070303256584298035, -0.5905099943842175847, 0.000000000000000000 ) ) ;
#83748=CARTESIAN_POINT ( 'NONE',  ( 11.10657215103663553, -52.67603735984217650, -3.750000000001792788 ) ) ;
#83758=EDGE_CURVE ( 'NONE', #63180, #91314, #80303, .T. ) ;
#83764=COLOUR_RGB ( '', 0.08235294, 0.09019608, 0.10196078) ;
#83776=FILL_AREA_STYLE_COLOUR ( '', #57335 ) ;
#83786=ORIENTED_EDGE ( 'NONE', *, *, #66402, .T. ) ;
#83798=SURFACE_SIDE_STYLE ('',( #77757 ) ) ;
#83803=AXIS2_PLACEMENT_3D ( 'NONE', #30642, #75169, #6679 ) ;
#83825=VERTEX_POINT ( 'NONE', #6703 ) ;
#83837=FACE_OUTER_BOUND ( 'NONE', #12941, .T. ) ;
#83845=SURFACE_SIDE_STYLE ('',( #76825 ) ) ;
#83848=ORIENTED_EDGE ( 'NONE', *, *, #85350, .T. ) ;
#83852=FILL_AREA_STYLE_COLOUR ( '', #93044 ) ;
#83860=EDGE_LOOP ( 'NONE', ( #53061, #15558, #88101, #50799 ) ) ;
#83861=SURFACE_STYLE_USAGE ( .BOTH. , #43872 ) ;
#83876=EDGE_CURVE ( 'NONE', #26706, #82021, #53183, .T. ) ;
#83879=CIRCLE ( 'NONE', #8859, 0.2500000000000002220 ) ;
#83898=EDGE_LOOP ( 'NONE', ( #8062, #38774, #2879, #42567 ) ) ;
#83900=CARTESIAN_POINT ( 'NONE',  ( 6.034747819232443078, -36.07388523689489546, 3.750000000000000000 ) ) ;
#83902=FACE_OUTER_BOUND ( 'NONE', #22176, .T. ) ;
#83906=CARTESIAN_POINT ( 'NONE',  ( -4.139423687100487470, -8.271184049145455575, -4.000000000000000000 ) ) ;
#83910=VERTEX_POINT ( 'NONE', #82697 ) ;
#83919=CIRCLE ( 'NONE', #96717, 0.2500000000000002220 ) ;
#83926=EDGE_LOOP ( 'NONE', ( #328, #56695, #88684, #84517 ) ) ;
#83934=CYLINDRICAL_SURFACE ( 'NONE', #69183, 0.1000000000000001166 ) ;
#83936=ADVANCED_FACE ( 'NONE', ( #38685 ), #60190, .F. ) ;
#83953=DIRECTION ( 'NONE',  ( -1.000000000000000000, 0.000000000000000000, 0.000000000000000000 ) ) ;
#83955=CARTESIAN_POINT ( 'NONE',  ( 6.673414917871782315, -55.62670566514463388, -2.750000000000000000 ) ) ;
#83974=SURFACE_STYLE_FILL_AREA ( #47442 ) ;
#83995=AXIS2_PLACEMENT_3D ( 'NONE', #21132, #51632, #82112 ) ;
#84011=CARTESIAN_POINT ( 'NONE',  ( -6.349999999999995204, -97.00000000000000000, 3.750000000000000000 ) ) ;
#84025=EDGE_CURVE ( 'NONE', #61288, #14585, #62808, .T. ) ;
#84039=ORIENTED_EDGE ( 'NONE', *, *, #62192, .T. ) ;
#84049=COLOUR_RGB ( '', 0.31764706, 0.68627451, 0.89019608) ;
#84066=CARTESIAN_POINT ( 'NONE',  ( 10.47195283030799651, -40.28639508432959815, 4.000000000000001776 ) ) ;
#84074=LINE ( 'NONE', #46074, #10664 ) ;
#84075=LINE ( 'NONE', #53561, #84914 ) ;
#84085=FACE_OUTER_BOUND ( 'NONE', #64973, .T. ) ;
#84089=CIRCLE ( 'NONE', #98539, 2.999999999999997780 ) ;
#84096=ADVANCED_FACE ( 'NONE', ( #10640 ), #39437, .F. ) ;
#84111=AXIS2_PLACEMENT_3D ( 'NONE', #87758, #19273, #35249 ) ;
#84119=AXIS2_PLACEMENT_3D ( 'NONE', #79138, #48144, #78158 ) ;
#84127=AXIS2_PLACEMENT_3D ( 'NONE', #78056, #77067, #24083 ) ;
#84143=AXIS2_PLACEMENT_3D ( 'NONE', #11081, #64549, #42085 ) ;
#84153=CARTESIAN_POINT ( 'NONE',  ( -8.330954874177404434, -7.272562134471185047, 3.750000000000000000 ) ) ;
#84161=EDGE_CURVE ( 'NONE', #1168, #92445, #35963, .T. ) ;
#84167=CARTESIAN_POINT ( 'NONE',  ( 8.979999999999991545, 0.000000000000000000, 2.900000000000000355 ) ) ;
#84168=ORIENTED_EDGE ( 'NONE', *, *, #71634, .F. ) ;
#84177=ORIENTED_EDGE ( 'NONE', *, *, #39298, .F. ) ;
#84188=ORIENTED_EDGE ( 'NONE', *, *, #74422, .T. ) ;
#84191=DIRECTION ( 'NONE',  ( 0.000000000000000000, -0.000000000000000000, -1.000000000000000000 ) ) ;
#84193=COLOUR_RGB ( '', 0.08235294, 0.09019608, 0.10196078) ;
#84194=CARTESIAN_POINT ( 'NONE',  ( 8.880000000000000782, 1.019547802438459216, 4.000000000000000000 ) ) ;
#84198=CARTESIAN_POINT ( 'NONE',  ( -3.500000000000000444, 1.019547802438453887, 3.750000000000000444 ) ) ;
#84201=CARTESIAN_POINT ( 'NONE',  ( -9.000000000000001776, 83.99999999999994316, -2.900000000000000799 ) ) ;
#84215=AXIS2_PLACEMENT_3D ( 'NONE', #41414, #32889, #48872 ) ;
#84217=AXIS2_PLACEMENT_3D ( 'NONE', #69997, #61985, #15041 ) ;
#84219=ORIENTED_EDGE ( 'NONE', *, *, #85560, .T. ) ;
#84224=SURFACE_SIDE_STYLE ('',( #82723 ) ) ;
#84227=DIRECTION ( 'NONE',  ( 1.000000000000000000, -0.000000000000000000, 0.000000000000000000 ) ) ;
#84248=DIRECTION ( 'NONE',  ( 0.9961946980917461003, -0.08715574274765139351, 0.000000000000000000 ) ) ;
#84249=EDGE_CURVE ( 'NONE', #89076, #34917, #54807, .T. ) ;
#84250=COLOUR_RGB ( '', 0.72549020, 0.75294118, 0.79215686) ;
#84256=CARTESIAN_POINT ( 'NONE',  ( 10.79855660033419262, -95.56318652451196272, -4.000000000000000000 ) ) ;
#84260=CARTESIAN_POINT ( 'NONE',  ( -3.750000000000000000, 36.75000000000000000, -3.750000000000000000 ) ) ;
#84267=CIRCLE ( 'NONE', #36348, 1.249999999999987121 ) ;
#84272=EDGE_CURVE ( 'NONE', #55236, #47721, #40500, .T. ) ;
#84280=CARTESIAN_POINT ( 'NONE',  ( 18.00000000000000355, 77.66934307245642799, 4.068269658013480949 ) ) ;
#84284=CARTESIAN_POINT ( 'NONE',  ( 3.969999999999999751, 36.75000000000000000, -2.750000000000000000 ) ) ;
#84295=FACE_OUTER_BOUND ( 'NONE', #13317, .T. ) ;
#84296=ORIENTED_EDGE ( 'NONE', *, *, #89313, .T. ) ;
#84299=EDGE_LOOP ( 'NONE', ( #80500, #92534, #21167, #48583 ) ) ;
#84303=ORIENTED_EDGE ( 'NONE', *, *, #74271, .F. ) ;
#84306=( NAMED_UNIT ( * ) PLANE_ANGLE_UNIT ( ) SI_UNIT ( $, .RADIAN. ) );
#84314=CARTESIAN_POINT ( 'NONE',  ( -3.949999999999997069, 99.99999999999998579, 8.000000000000000000 ) ) ;
#84336=CARTESIAN_POINT ( 'NONE',  ( 4.395712687241005945, -0.8323168403886667122, -2.750000000000000444 ) ) ;
#84339=SURFACE_STYLE_FILL_AREA ( #23838 ) ;
#84352=AXIS2_PLACEMENT_3D ( 'NONE', #36056, #44545, #89554 ) ;
#84353=CARTESIAN_POINT ( 'NONE',  ( -10.54707717934878275, -44.61285707881522455, -3.999999999999998224 ) ) ;
#84364=EDGE_CURVE ( 'NONE', #25626, #98330, #46822, .T. ) ;
#84369=ORIENTED_EDGE ( 'NONE', *, *, #3440, .F. ) ;
#84397=EDGE_LOOP ( 'NONE', ( #71126, #75030, #66996, #92874 ) ) ;
#84405=CARTESIAN_POINT ( 'NONE',  ( 5.115475850186006923, -17.53855045867880591, 3.750000000001609823 ) ) ;
#84409=FACE_OUTER_BOUND ( 'NONE', #89468, .T. ) ;
#84411=CARTESIAN_POINT ( 'NONE',  ( -10.88853822400146676, 46.97908644289115898, 2.899999999999999467 ) ) ;
#84424=AXIS2_PLACEMENT_3D ( 'NONE', #86268, #56269, #86761 ) ;
#84426=DIRECTION ( 'NONE',  ( 1.000000000000000000, -0.000000000000000000, 0.000000000000000000 ) ) ;
#84437=CARTESIAN_POINT ( 'NONE',  ( 5.129999999999995453, 43.00000000000000711, 6.500000000000000888 ) ) ;
#84439=ADVANCED_FACE ( 'NONE', ( #15936 ), #37289, .T. ) ;
#84444=EDGE_LOOP ( 'NONE', ( #91083, #46913, #30247, #35307 ) ) ;
#84454=DIRECTION ( 'NONE',  ( -1.000000000000000000, 0.000000000000000000, -0.000000000000000000 ) ) ;
#84476=CARTESIAN_POINT ( 'NONE',  ( -7.750000000000000000, 41.24999999999999289, -6.250000000000000000 ) ) ;
#84481=LINE ( 'NONE', #70460, #4911 ) ;
#84507=ADVANCED_FACE ( 'NONE', ( #93399 ), #83934, .T. ) ;
#84512=EDGE_CURVE ( 'NONE', #7091, #87189, #29268, .T. ) ;
#84515=CARTESIAN_POINT ( 'NONE',  ( -7.121448108906508700, -73.25984652122873797, -3.750000000000000888 ) ) ;
#84517=ORIENTED_EDGE ( 'NONE', *, *, #72493, .F. ) ;
#84533=AXIS2_PLACEMENT_3D ( 'NONE', #28487, #36488, #96511 ) ;
#84549=ORIENTED_EDGE ( 'NONE', *, *, #83264, .F. ) ;
#84563=DIRECTION ( 'NONE',  ( 0.000000000000000000, -1.000000000000000000, -0.000000000000000000 ) ) ;
#84577=AXIS2_PLACEMENT_3D ( 'NONE', #7025, #62464, #83018 ) ;
#84580=DIRECTION ( 'NONE',  ( 1.000000000000000000, 6.938893903907221278E-15, 0.000000000000000000 ) ) ;
#84582=EDGE_CURVE ( 'NONE', #55236, #20156, #34034, .T. ) ;
#84584=ORIENTED_EDGE ( 'NONE', *, *, #78452, .F. ) ;
#84622=ADVANCED_FACE ( 'NONE', ( #91927 ), #85413, .T. ) ;
#84626=ORIENTED_EDGE ( 'NONE', *, *, #21144, .F. ) ;
#84632=CARTESIAN_POINT ( 'NONE',  ( -11.62541523589044168, -75.76371818141878123, 3.999999999998198330 ) ) ;
#84639=AXIS2_PLACEMENT_3D ( 'NONE', #32578, #25110, #15142 ) ;
#84643=ORIENTED_EDGE ( 'NONE', *, *, #54416, .F. ) ;
#84665=FACE_OUTER_BOUND ( 'NONE', #2678, .T. ) ;
#84671=CARTESIAN_POINT ( 'NONE',  ( 15.00000000000000000, 77.07179676972447169, 4.000000000000000000 ) ) ;
#84674=CARTESIAN_POINT ( 'NONE',  ( 8.650320195874050100, -1.048895414467672094, 4.000000000000000000 ) ) ;
#84677=CARTESIAN_POINT ( 'NONE',  ( 17.99999999999999645, 99.99999999999998579, 8.000000000000000000 ) ) ;
#84685=( NAMED_UNIT ( * ) SI_UNIT ( $, .STERADIAN. ) SOLID_ANGLE_UNIT ( ) );
#84704=EDGE_CURVE ( 'NONE', #71742, #55464, #34357, .T. ) ;
#84705=CARTESIAN_POINT ( 'NONE',  ( 8.630000000000000782, 1.019547802438458550, 4.000000000000000000 ) ) ;
#84711=FACE_OUTER_BOUND ( 'NONE', #79540, .T. ) ;
#84716=LINE ( 'NONE', #14253, #5371 ) ;
#84728=CARTESIAN_POINT ( 'NONE',  ( -18.89999999999999147, 91.00000000000000000, -7.750000000000000000 ) ) ;
#84742=FACE_OUTER_BOUND ( 'NONE', #61546, .T. ) ;
#84746=EDGE_CURVE ( 'NONE', #6373, #35739, #70826, .T. ) ;
#84748=VERTEX_POINT ( 'NONE', #48388 ) ;
#84749=LINE ( 'NONE', #16254, #35714 ) ;
#84759=CARTESIAN_POINT ( 'NONE',  ( 18.00000000000000000, 78.06026162106516608, 3.869897288748200825 ) ) ;
#84762=CARTESIAN_POINT ( 'NONE',  ( -7.072388532689616980, -84.40601219567531643, 4.000000000000805578 ) ) ;
#84763=ORIENTED_EDGE ( 'NONE', *, *, #83031, .F. ) ;
#84765=EDGE_LOOP ( 'NONE', ( #71545, #53626, #86437, #42336 ) ) ;
#84767=ORIENTED_EDGE ( 'NONE', *, *, #48860, .T. ) ;
#84771=SURFACE_STYLE_FILL_AREA ( #31258 ) ;
#84773=AXIS2_PLACEMENT_3D ( 'NONE', #48653, #10667, #64621 ) ;
#84775=EDGE_LOOP ( 'NONE', ( #8043, #19553, #43072, #52897 ) ) ;
#84778=ORIENTED_EDGE ( 'NONE', *, *, #46018, .T. ) ;
#84783=EDGE_CURVE ( 'NONE', #27291, #18983, #26866, .T. ) ;
#84788=ORIENTED_EDGE ( 'NONE', *, *, #89192, .T. ) ;
#84808=DIRECTION ( 'NONE',  ( 0.000000000000000000, 1.000000000000000000, 0.000000000000000000 ) ) ;
#84813=CARTESIAN_POINT ( 'NONE',  ( -10.28286150160520762, 89.18763609516977908, 5.839555419999288510 ) ) ;
#84815=CARTESIAN_POINT ( 'NONE',  ( 6.507545146409696279, -58.30914921458864342, -2.500000000000000000 ) ) ;
#84817=SURFACE_SIDE_STYLE ('',( #84339 ) ) ;
#84826=CARTESIAN_POINT ( 'NONE',  ( -16.60833333333331652, 99.75000000000000000, -8.000000000000000000 ) ) ;
#84829=CYLINDRICAL_SURFACE ( 'NONE', #93829, 0.1000000000000001166 ) ;
#84830=CARTESIAN_POINT ( 'NONE',  ( -10.79676793866758011, -44.60032227172015240, -4.000000000003602452 ) ) ;
#84854=DIRECTION ( 'NONE',  ( -1.000000000000000000, -2.569960705150834273E-16, 0.000000000000000000 ) ) ;
#84860=( NAMED_UNIT ( * ) PLANE_ANGLE_UNIT ( ) SI_UNIT ( $, .RADIAN. ) );
#84873=EDGE_CURVE ( 'NONE', #3878, #75561, #72357, .T. ) ;
#84875=ORIENTED_EDGE ( 'NONE', *, *, #94690, .F. ) ;
#84886=COLOUR_RGB ( '', 0.31764706, 0.68627451, 0.89019608) ;
#84912=ORIENTED_EDGE ( 'NONE', *, *, #34448, .T. ) ;
#84914=VECTOR ( 'NONE', #9056, 1000.000000000000000 ) ;
#84923=CARTESIAN_POINT ( 'NONE',  ( -6.000000000000009770, 40.74999999999999289, 4.250000000000000000 ) ) ;
#84928=EDGE_CURVE ( 'NONE', #1559, #13075, #63389, .T. ) ;
#84933=EDGE_CURVE ( 'NONE', #95526, #68087, #43919, .T. ) ;
#84938=CARTESIAN_POINT ( 'NONE',  ( 4.474002695404426966, -3.767820133606233579, -2.750000000000000000 ) ) ;
#84939=CARTESIAN_POINT ( 'NONE',  ( 4.395712687241356775, -0.8323168404091368933, 2.750000000000000000 ) ) ;
#84963=LINE ( 'NONE', #62944, #75126 ) ;
#84981=DIRECTION ( 'NONE',  ( 0.000000000000000000, 0.000000000000000000, -1.000000000000000000 ) ) ;
#84993=DIRECTION ( 'NONE',  ( 0.000000000000000000, 0.000000000000000000, -1.000000000000000000 ) ) ;
#84999=ADVANCED_FACE ( 'NONE', ( #82824 ), #6836, .T. ) ;
#85001=PLANE ( 'NONE',  #43980 ) ;
#85004=ORIENTED_EDGE ( 'NONE', *, *, #73061, .F. ) ;
#85020=PLANE ( 'NONE',  #15828 ) ;
#85030=ORIENTED_EDGE ( 'NONE', *, *, #70024, .F. ) ;
#85086=CARTESIAN_POINT ( 'NONE',  ( 9.779999999999990479, 20.99999999999999645, 0.000000000000000000 ) ) ;
#85088=PLANE ( 'NONE',  #43185 ) ;
#85094=LINE ( 'NONE', #8601, #85650 ) ;
#85112=STYLED_ITEM ( 'NONE', ( #87790 ), #66016 ) ;
#85113=( LENGTH_UNIT ( ) NAMED_UNIT ( * ) SI_UNIT ( .MILLI., .METRE. ) );
#85116=ORIENTED_EDGE ( 'NONE', *, *, #25227, .T. ) ;
#85121=CARTESIAN_POINT ( 'NONE',  ( -9.793382739345220855, -28.00152668697253233, 4.000000000000000000 ) ) ;
#85126=CIRCLE ( 'NONE', #53145, 0.2500000000000002220 ) ;
#85131=B_SPLINE_CURVE_WITH_KNOTS ( 'NONE', 3,
 ( #17834, #78824, #94307, #49789, #48316, #71814, #4312, #87787, #11796, #26304, #40832, #19787, #25830, #3320, #93823, #19303, #25353, #10334, #72292, #42303, #55836, #50276, #72775, #42797 ),
 .UNSPECIFIED., .F., .F.,
 ( 4, 2, 2, 2, 2, 2, 2, 2, 2, 2, 2, 4 ),
 ( 0.000000000000000000, 0.003100981433949152270, 0.006201962867898304539, 0.01240392573579660908, 0.02480785147159321816, 0.04961570294318642937, 0.06201962867898304366, 0.07442355441477965794, 0.08682748015057627222, 0.09302944301847457242, 0.09613042445242370171, 0.09923140588637283099 ),
 .UNSPECIFIED. ) ;
#85132=AXIS2_PLACEMENT_3D ( 'NONE', #66631, #18676, #79665 ) ;
#85138=EDGE_LOOP ( 'NONE', ( #39900, #53752, #77631, #75292 ) ) ;
#85144=CARTESIAN_POINT ( 'NONE',  ( 0.000000000000000000, 9.750000000000000000, -3.750000000000000000 ) ) ;
#85148=ORIENTED_EDGE ( 'NONE', *, *, #68798, .T. ) ;
#85161=CIRCLE ( 'NONE', #14874, 0.2500000000000002220 ) ;
#85165=CARTESIAN_POINT ( 'NONE',  ( -3.627483523066825644, -3.617667194781895024, 2.749999999999798828 ) ) ;
#85167=CYLINDRICAL_SURFACE ( 'NONE', #57346, 0.2500000000000002220 ) ;
#85182=EDGE_CURVE ( 'NONE', #28677, #34483, #58250, .T. ) ;
#85185=MECHANICAL_DESIGN_GEOMETRIC_PRESENTATION_REPRESENTATION('',(#21315),#34271);
#85202=CARTESIAN_POINT ( 'NONE',  ( 14.99999999999998046, 69.99999999999998579, -6.250000000000000000 ) ) ;
#85222=UNCERTAINTY_MEASURE_WITH_UNIT (LENGTH_MEASURE( 1.000000000000000082E-05 ), #75035, 'distance_accuracy_value', 'NONE');
#85236=( LENGTH_UNIT ( ) NAMED_UNIT ( * ) SI_UNIT ( .MILLI., .METRE. ) );
#85238=ADVANCED_FACE ( 'NONE', ( #61304 ), #61795, .T. ) ;
#85240=EDGE_LOOP ( 'NONE', ( #80053, #58526, #88351, #71505 ) ) ;
#85252=CARTESIAN_POINT ( 'NONE',  ( 17.99999999995698019, 77.36262727519604709, 4.161036774752517431 ) ) ;
#85255=CARTESIAN_POINT ( 'NONE',  ( -3.889970118577499747, -8.287734203612208361, 3.750000000000403233 ) ) ;
#85261=ORIENTED_EDGE ( 'NONE', *, *, #44833, .T. ) ;
#85265=PRESENTATION_STYLE_ASSIGNMENT (( #54744 ) ) ;
#85295=( NAMED_UNIT ( * ) SI_UNIT ( $, .STERADIAN. ) SOLID_ANGLE_UNIT ( ) );
#85306=CARTESIAN_POINT ( 'NONE',  ( -8.004649405379435478, 84.50413264541207070, 3.999860480132925833 ) ) ;
#85310=( LENGTH_UNIT ( ) NAMED_UNIT ( * ) SI_UNIT ( .MILLI., .METRE. ) );
#85317=CARTESIAN_POINT ( 'NONE',  ( -19.89999999999999858, 98.99999999999998579, -7.750000000000000000 ) ) ;
#85321=AXIS2_PLACEMENT_3D ( 'NONE', #68458, #55910, #48881 ) ;
#85324=LINE ( 'NONE', #91850, #24410 ) ;
#85334=LINE ( 'NONE', #76842, #54839 ) ;
#85335=CARTESIAN_POINT ( 'NONE',  ( 9.779999999999988702, 26.99999999999999645, -2.900000000000000799 ) ) ;
#85346=( LENGTH_UNIT ( ) NAMED_UNIT ( * ) SI_UNIT ( .MILLI., .METRE. ) );
#85350=EDGE_CURVE ( 'NONE', #18642, #74685, #18384, .T. ) ;
#85369=ORIENTED_EDGE ( 'NONE', *, *, #5580, .T. ) ;
#85396=AXIS2_PLACEMENT_3D ( 'NONE', #50862, #20861, #43350 ) ;
#85398=LINE ( 'NONE', #98959, #49891 ) ;
#85413=PLANE ( 'NONE',  #73947 ) ;
#85433=CARTESIAN_POINT ( 'NONE',  ( 5.783743716948903213, -36.05632648177958544, 2.500000000000000888 ) ) ;
#85445=B_SPLINE_CURVE_WITH_KNOTS ( 'NONE', 3,
 ( #53813, #61791, #23333, #54288, #2314, #46312, #1331, #92300, #17303, #76799, #62278, #55280, #69311, #92784, #53310, #16804, #70302, #47778, #832, #31292, #78276, #30803 ),
 .UNSPECIFIED., .F., .F.,
 ( 4, 2, 2, 2, 2, 2, 2, 2, 2, 2, 4 ),
 ( -6.000000000051943759E-08, 0.002788756152630997125, 0.005577572305261994760, 0.01115520461052398916, 0.02231046922104798144, 0.03346573383157196852, 0.04462099844209594518, 0.06693152766314391933, 0.07808679227366789599, 0.08366442457892990514, 0.08924205688419188653 ),
 .UNSPECIFIED. ) ;
#85454=CARTESIAN_POINT ( 'NONE',  ( 4.395886033851783559, -0.8422402087859571784, -3.750000000000000000 ) ) ;
#85471=CARTESIAN_POINT ( 'NONE',  ( 15.55000000000000071, 99.99999999999998579, 8.000000000000000000 ) ) ;
#85496=VERTEX_POINT ( 'NONE', #11258 ) ;
#85500=AXIS2_PLACEMENT_3D ( 'NONE', #16232, #91229, #76240 ) ;
#85508=DIRECTION ( 'NONE',  ( 1.000000000000000000, 0.000000000000000000, 0.000000000000000000 ) ) ;
#85522=AXIS2_PLACEMENT_3D ( 'NONE', #36263, #95789, #12765 ) ;
#85540=VERTEX_POINT ( 'NONE', #1821 ) ;
#85541=CIRCLE ( 'NONE', #42433, 1.500000000000001332 ) ;
#85543=ORIENTED_EDGE ( 'NONE', *, *, #80540, .F. ) ;
#85546=AXIS2_PLACEMENT_3D ( 'NONE', #55463, #39485, #76485 ) ;
#85551=FILL_AREA_STYLE_COLOUR ( '', #84193 ) ;
#85560=EDGE_CURVE ( 'NONE', #38399, #59804, #77464, .T. ) ;
#85561=CARTESIAN_POINT ( 'NONE',  ( -3.750000000000000000, 36.75000000000000000, 3.750000000000000000 ) ) ;
#85567=ORIENTED_EDGE ( 'NONE', *, *, #51593, .F. ) ;
#85576=DIRECTION ( 'NONE',  ( 1.000000000000000000, 0.000000000000000000, 0.000000000000000000 ) ) ;
#85585=CARTESIAN_POINT ( 'NONE',  ( -7.750000000000003553, -0.02150918539402481983, 4.000000000000000000 ) ) ;
#85610=STYLED_ITEM ( 'NONE', ( #87867 ), #37262 ) ;
#85630=EDGE_LOOP ( 'NONE', ( #52306, #86738, #65335 ) ) ;
#85636=FACE_OUTER_BOUND ( 'NONE', #38009, .T. ) ;
#85639=EDGE_LOOP ( 'NONE', ( #42847, #90652, #6157, #23810 ) ) ;
#85650=VECTOR ( 'NONE', #41080, 1000.000000000000000 ) ;
#85651=DIRECTION ( 'NONE',  ( 0.000000000000000000, -0.000000000000000000, -1.000000000000000000 ) ) ;
#85654=CARTESIAN_POINT ( 'NONE',  ( -5.328486666255602522, -28.65465727419762487, 2.750000000000000444 ) ) ;
#85664=FACE_OUTER_BOUND ( 'NONE', #31860, .T. ) ;
#85669=SURFACE_STYLE_FILL_AREA ( #25670 ) ;
#85672=VECTOR ( 'NONE', #12637, 1000.000000000000000 ) ;
#85675=ADVANCED_FACE ( 'NONE', ( #65726 ), #59978, .T. ) ;
#85680=CARTESIAN_POINT ( 'NONE',  ( 8.879999999999991900, 76.07179676972447169, 4.000000000000000000 ) ) ;
#85688=DIRECTION ( 'NONE',  ( 1.257402221000611116E-16, -1.000000000000000000, 0.000000000000000000 ) ) ;
#85696=CARTESIAN_POINT ( 'NONE',  ( -3.750000000000000000, 37.25000000000000000, 3.750000000000000000 ) ) ;
#85707=EDGE_CURVE ( 'NONE', #65197, #96234, #26433, .T. ) ;
#85716=ORIENTED_EDGE ( 'NONE', *, *, #13123, .T. ) ;
#85717=CARTESIAN_POINT ( 'NONE',  ( 8.955816604532303771, -3.107613341149440878, -3.750000000000000000 ) ) ;
#85725=SURFACE_STYLE_USAGE ( .BOTH. , #32704 ) ;
#85732=DIRECTION ( 'NONE',  ( 0.000000000000000000, -0.000000000000000000, -1.000000000000000000 ) ) ;
#85738=FILL_AREA_STYLE_COLOUR ( '', #35858 ) ;
#85749=CARTESIAN_POINT ( 'NONE',  ( -3.889970118670757593, -8.287734203605914729, 4.000000000000807354 ) ) ;
#85750=EDGE_CURVE ( 'NONE', #21472, #31285, #21680, .T. ) ;
#85761=ORIENTED_EDGE ( 'NONE', *, *, #92324, .F. ) ;
#85763=CIRCLE ( 'NONE', #42633, 0.2500000000000000000 ) ;
#85799=LINE ( 'NONE', #54789, #39102 ) ;
#85810=SURFACE_SIDE_STYLE ('',( #69827 ) ) ;
#85820=ORIENTED_EDGE ( 'NONE', *, *, #74422, .F. ) ;
#85824=DIRECTION ( 'NONE',  ( 1.000000000000000000, -0.000000000000000000, -0.000000000000000000 ) ) ;
#85843=FILL_AREA_STYLE ('',( #25832 ) ) ;
#85856=DIRECTION ( 'NONE',  ( -1.000000000000000000, -1.927470528863119542E-16, 0.000000000000000000 ) ) ;
#85872=ORIENTED_EDGE ( 'NONE', *, *, #58377, .F. ) ;
#85892=CIRCLE ( 'NONE', #58689, 2.899999999999998579 ) ;
#85901=TOROIDAL_SURFACE ( 'NONE', #4480, 2.250000000000001332, 0.2500000000000000000 ) ;
#85909=CYLINDRICAL_SURFACE ( 'NONE', #50648, 0.2500000000000002220 ) ;
#85914=( NAMED_UNIT ( * ) SI_UNIT ( $, .STERADIAN. ) SOLID_ANGLE_UNIT ( ) );
#85917=VERTEX_POINT ( 'NONE', #81022 ) ;
#85918=STYLED_ITEM ( 'NONE', ( #37668 ), #69668 ) ;
#85934=DIRECTION ( 'NONE',  ( -0.000000000000000000, -0.000000000000000000, 1.000000000000000000 ) ) ;
#85944=DIRECTION ( 'NONE',  ( 1.000000000000000000, -0.000000000000000000, -0.000000000000000000 ) ) ;
#85948=CARTESIAN_POINT ( 'NONE',  ( 9.879999999999990123, 20.99999999999999645, 1.249999999999987121 ) ) ;
#85955=DIRECTION ( 'NONE',  ( 1.000000000000000000, 2.107602052970794797E-16, -0.000000000000000000 ) ) ;
#85970=DIRECTION ( 'NONE',  ( 1.000000000000000000, 0.000000000000000000, 0.000000000000000000 ) ) ;
#85981=DIRECTION ( 'NONE',  ( -1.257402221000611116E-16, 1.000000000000000000, 0.000000000000000000 ) ) ;
#85991=TOROIDAL_SURFACE ( 'NONE', #61989, 2.899999999999999467, 0.1000000000000000056 ) ;
#85996=ORIENTED_EDGE ( 'NONE', *, *, #45977, .F. ) ;
#86010=VERTEX_POINT ( 'NONE', #66013 ) ;
#86019=ORIENTED_EDGE ( 'NONE', *, *, #59281, .F. ) ;
#86029=CARTESIAN_POINT ( 'NONE',  ( -57.13414634146340632, 45.70731707317067816, -8.000000000000000000 ) ) ;
#86039=ORIENTED_EDGE ( 'NONE', *, *, #82686, .F. ) ;
#86047=SURFACE_STYLE_FILL_AREA ( #16567 ) ;
#86050=DIRECTION ( 'NONE',  ( 0.000000000000000000, 0.000000000000000000, -1.000000000000000000 ) ) ;
#86056=AXIS2_PLACEMENT_3D ( 'NONE', #84167, #22675, #15179 ) ;
#86079=CARTESIAN_POINT ( 'NONE',  ( -8.000000000000000000, 80.07179676972448590, -6.500000000000000888 ) ) ;
#86088=CARTESIAN_POINT ( 'NONE',  ( -4.260926550508235877, -13.83313246298655130, -3.749999999999999112 ) ) ;
#86090=ORIENTED_EDGE ( 'NONE', *, *, #4098, .F. ) ;
#86094=CARTESIAN_POINT ( 'NONE',  ( 8.979999999999991545, 27.03929484861773958, 3.000000000000000000 ) ) ;
#86107=VERTEX_POINT ( 'NONE', #82504 ) ;
#86113=DIRECTION ( 'NONE',  ( 1.000000000000000000, 0.000000000000000000, 0.000000000000000000 ) ) ;
#86118=CARTESIAN_POINT ( 'NONE',  ( 3.969999999999999751, 10.00000000000000000, -4.000000000000000000 ) ) ;
#86120=MECHANICAL_DESIGN_GEOMETRIC_PRESENTATION_REPRESENTATION('',(#94029),#98922);
#86132=LINE ( 'NONE', #62124, #7147 ) ;
#86133=ADVANCED_FACE ( 'NONE', ( #28518 ), #89515, .F. ) ;
#86147=VECTOR ( 'NONE', #64915, 1000.000000000000114 ) ;
#86156=EDGE_CURVE ( 'NONE', #20729, #66694, #5035, .T. ) ;
#86157=CARTESIAN_POINT ( 'NONE',  ( 0.4400000000000020006, 1.019547802438468986, 3.750000000000000000 ) ) ;
#86160=DIRECTION ( 'NONE',  ( -0.000000000000000000, -0.000000000000000000, 1.000000000000000000 ) ) ;
#86166=SURFACE_SIDE_STYLE ('',( #85669 ) ) ;
#86169=VECTOR ( 'NONE', #43873, 1000.000000000000114 ) ;
#86175=EDGE_LOOP ( 'NONE', ( #11598, #6685, #34209, #96709 ) ) ;
#86184=DIRECTION ( 'NONE',  ( -1.000000000000000000, 0.000000000000000000, 0.000000000000000000 ) ) ;
#86208=ORIENTED_EDGE ( 'NONE', *, *, #56040, .T. ) ;
#86220=ORIENTED_EDGE ( 'NONE', *, *, #63902, .T. ) ;
#86221=VERTEX_POINT ( 'NONE', #14521 ) ;
#86224=CARTESIAN_POINT ( 'NONE',  ( -10.77730536144846596, -98.63085534186639336, -3.750000000000000000 ) ) ;
#86230=CARTESIAN_POINT ( 'NONE',  ( -6.000000000000000000, 78.07179676972447169, -6.500000000000000888 ) ) ;
#86234=CARTESIAN_POINT ( 'NONE',  ( 17.99999999999999645, 78.53751499213471732, 3.955843470927898675 ) ) ;
#86237=CARTESIAN_POINT ( 'NONE',  ( -6.982525766850296911, -88.11956318484570261, 3.750000000000000000 ) ) ;
#86240=EDGE_LOOP ( 'NONE', ( #24562, #51813, #19701, #79795 ) ) ;
#86268=CARTESIAN_POINT ( 'NONE',  ( 4.469999999999999751, 36.75000000000000000, -3.750000000000000000 ) ) ;
#86273=CARTESIAN_POINT ( 'NONE',  ( -6.732636091893141383, -88.11213685669363826, -2.750000000000000000 ) ) ;
#86276=DIRECTION ( 'NONE',  ( 0.000000000000000000, -0.000000000000000000, -1.000000000000000000 ) ) ;
#86280=FILL_AREA_STYLE_COLOUR ( '', #98002 ) ;
#86283=AXIS2_PLACEMENT_3D ( 'NONE', #39295, #55768, #78760 ) ;
#86298=PRESENTATION_STYLE_ASSIGNMENT (( #92804 ) ) ;
#86302=AXIS2_PLACEMENT_3D ( 'NONE', #8597, #47074, #47579 ) ;
#86315=CARTESIAN_POINT ( 'NONE',  ( -8.114998381645635916, 86.24535146302233102, -4.289708087854925189 ) ) ;
#86322=ORIENTED_EDGE ( 'NONE', *, *, #6894, .T. ) ;
#86324=CARTESIAN_POINT ( 'NONE',  ( -7.750000000000000000, 0.000000000000000000, 4.000000000000000000 ) ) ;
#86332=CARTESIAN_POINT ( 'NONE',  ( 6.880000000000009663, 41.24999999999999289, -6.250000000000000000 ) ) ;
#86334=SURFACE_STYLE_FILL_AREA ( #55840 ) ;
#86354=AXIS2_PLACEMENT_3D ( 'NONE', #59517, #6517, #51027 ) ;
#86385=CIRCLE ( 'NONE', #76738, 2.000000000000000000 ) ;
#86392=EDGE_CURVE ( 'NONE', #67453, #50286, #43987, .T. ) ;
#86403=CARTESIAN_POINT ( 'NONE',  ( -10.88853822400146676, 46.97908644289115898, -2.900000000000000799 ) ) ;
#86410=( LENGTH_UNIT ( ) NAMED_UNIT ( * ) SI_UNIT ( .MILLI., .METRE. ) );
#86413=CARTESIAN_POINT ( 'NONE',  ( 4.879999999999994564, 43.00000000000000711, -6.500000000000000888 ) ) ;
#86430=CARTESIAN_POINT ( 'NONE',  ( 9.113259239972942183, -7.249774014816905421, 3.750000000000001332 ) ) ;
#86431=EDGE_CURVE ( 'NONE', #69653, #96102, #75975, .T. ) ;
#86437=ORIENTED_EDGE ( 'NONE', *, *, #66614, .F. ) ;
#86440=CARTESIAN_POINT ( 'NONE',  ( -5.068142462297546835, -24.94450071861959728, -2.500000000000806022 ) ) ;
#86446=CARTESIAN_POINT ( 'NONE',  ( 4.879999999999991900, 76.07179676972444327, -4.250000000000000000 ) ) ;
#86448=FACE_OUTER_BOUND ( 'NONE', #5588, .T. ) ;
#86463=DIRECTION ( 'NONE',  ( 0.000000000000000000, 1.000000000000000000, 0.000000000000000000 ) ) ;
#86471=CARTESIAN_POINT ( 'NONE',  ( 6.432108699068925795, -88.20011490510430008, -2.750000000000000000 ) ) ;
#86475=DIRECTION ( 'NONE',  ( -4.336808689942013792E-16, 1.000000000000000000, 0.000000000000000000 ) ) ;
#86498=ADVANCED_FACE ( 'NONE', ( #74398 ), #5921, .T. ) ;
#86500=( NAMED_UNIT ( * ) SI_UNIT ( $, .STERADIAN. ) SOLID_ANGLE_UNIT ( ) );
#86503=DIRECTION ( 'NONE',  ( -1.000000000000000000, 0.000000000000000000, 0.000000000000000000 ) ) ;
#86530=LINE ( 'NONE', #18030, #61336 ) ;
#86533=FACE_OUTER_BOUND ( 'NONE', #97974, .T. ) ;
#86539=SURFACE_SIDE_STYLE ('',( #18529 ) ) ;
#86540=ORIENTED_EDGE ( 'NONE', *, *, #73494, .T. ) ;
#86560=DIRECTION ( 'NONE',  ( 2.569960705150826877E-16, -1.000000000000000000, 0.000000000000000000 ) ) ;
#86562=CIRCLE ( 'NONE', #6763, 0.2500000000000002220 ) ;
#86571=CARTESIAN_POINT ( 'NONE',  ( -9.823916613421536326, -32.16564667764521346, 4.000000000000000888 ) ) ;
#86579=CARTESIAN_POINT ( 'NONE',  ( -6.982525766850296911, -88.11956318484570261, -3.750000000000000000 ) ) ;
#86598=VERTEX_POINT ( 'NONE', #60385 ) ;
#86617=EDGE_LOOP ( 'NONE', ( #26205, #15785, #48015, #76741 ) ) ;
#86626=ORIENTED_EDGE ( 'NONE', *, *, #73948, .F. ) ;
#86627=STYLED_ITEM ( 'NONE', ( #38097 ), #48292 ) ;
#86631=VECTOR ( 'NONE', #73374, 1000.000000000000000 ) ;
#86642=CARTESIAN_POINT ( 'NONE',  ( -3.585386599742081071, -2.690194976740612809, 2.750000000000202061 ) ) ;
#86643=ORIENTED_EDGE ( 'NONE', *, *, #93876, .F. ) ;
#86644=CARTESIAN_POINT ( 'NONE',  ( 10.72176212046095145, -40.27637155869545893, 3.750000000000000000 ) ) ;
#86649=CARTESIAN_POINT ( 'NONE',  ( -4.000000000000000000, 37.00000000000000000, 2.500000000000000000 ) ) ;
#86650=LINE ( 'NONE', #33617, #28444 ) ;
#86651=DIRECTION ( 'NONE',  ( 0.000000000000000000, 0.000000000000000000, 1.000000000000000000 ) ) ;
#86652=DIRECTION ( 'NONE',  ( -1.000000000000000000, -1.483861936729427615E-16, 0.000000000000000000 ) ) ;
#86679=LINE ( 'NONE', #11163, #85672 ) ;
#86702=CARTESIAN_POINT ( 'NONE',  ( 4.722628015970558479, -9.822377395415374579, 2.750000000000000000 ) ) ;
#86711=VERTEX_POINT ( 'NONE', #75790 ) ;
#86714=ORIENTED_EDGE ( 'NONE', *, *, #62755, .F. ) ;
#86721=SURFACE_STYLE_USAGE ( .BOTH. , #64187 ) ;
#86729=CARTESIAN_POINT ( 'NONE',  ( 9.879999999999991900, 20.99999999999999645, 0.000000000000000000 ) ) ;
#86733=CARTESIAN_POINT ( 'NONE',  ( -7.080143328635299049, -69.54337233422661768, 4.000000000001613820 ) ) ;
#86738=ORIENTED_EDGE ( 'NONE', *, *, #47800, .T. ) ;
#86761=DIRECTION ( 'NONE',  ( 0.000000000000000000, 0.000000000000000000, 1.000000000000000000 ) ) ;
#86765=AXIS2_PLACEMENT_3D ( 'NONE', #6243, #3419, #64868 ) ;
#86774=SURFACE_SIDE_STYLE ('',( #17789 ) ) ;
#86784=CARTESIAN_POINT ( 'NONE',  ( -7.754961693898215991, 84.52280956283338753, 4.000000000000000000 ) ) ;
#86800=AXIS2_PLACEMENT_3D ( 'NONE', #69224, #22744, #37261 ) ;
#86801=ADVANCED_FACE ( 'NONE', ( #46286 ), #90790, .F. ) ;
#86804=CARTESIAN_POINT ( 'NONE',  ( -3.499999999999998668, 1.019547802438465434, 2.750000000000000444 ) ) ;
#86822=CARTESIAN_POINT ( 'NONE',  ( -19.64999999999999858, 0.000000000000000000, 8.000000000000000000 ) ) ;
#86825=DIRECTION ( 'NONE',  ( 0.000000000000000000, -1.000000000000000000, 0.000000000000000000 ) ) ;
#86832=( GEOMETRIC_REPRESENTATION_CONTEXT ( 3 ) GLOBAL_UNCERTAINTY_ASSIGNED_CONTEXT ( ( #18522 ) ) GLOBAL_UNIT_ASSIGNED_CONTEXT ( ( #37169, #21669, #82148 ) ) REPRESENTATION_CONTEXT ( 'NONE', 'WORKASPACE' ) );
#86837=DIRECTION ( 'NONE',  ( 1.927470528863119542E-16, -1.000000000000000000, 0.000000000000000000 ) ) ;
#86845=VECTOR ( 'NONE', #57635, 1000.000000000000114 ) ;
#86851=LINE ( 'NONE', #95325, #82478 ) ;
#86855=PLANE ( 'NONE',  #53172 ) ;
#86865=ORIENTED_EDGE ( 'NONE', *, *, #88187, .T. ) ;
#86877=ORIENTED_EDGE ( 'NONE', *, *, #50359, .F. ) ;
#86881=CARTESIAN_POINT ( 'NONE',  ( -8.029112100182558720, -1.061264519223844571, 3.750000000000001332 ) ) ;
#86884=CARTESIAN_POINT ( 'NONE',  ( -4.000000000000000000, 37.25000000000000000, -4.000000000000000000 ) ) ;
#86889=DIRECTION ( 'NONE',  ( -0.000000000000000000, -0.000000000000000000, -1.000000000000000000 ) ) ;
#86919=DIRECTION ( 'NONE',  ( -1.927470528863119542E-16, 1.000000000000000000, 0.000000000000000000 ) ) ;
#86920=CARTESIAN_POINT ( 'NONE',  ( -6.606690058644155705, -50.93246948813188624, -2.500000000001612044 ) ) ;
#86927=CARTESIAN_POINT ( 'NONE',  ( -7.371420888394233373, -73.25401859617250011, 4.000000000000000888 ) ) ;
#86946=ORIENTED_EDGE ( 'NONE', *, *, #68204, .T. ) ;
#86955=ORIENTED_EDGE ( 'NONE', *, *, #41970, .F. ) ;
#86959=ORIENTED_EDGE ( 'NONE', *, *, #21122, .F. ) ;
#86971=CARTESIAN_POINT ( 'NONE',  ( -9.208505132027131168, -19.73424747731175088, -3.750000000000000444 ) ) ;
#86973=AXIS2_PLACEMENT_3D ( 'NONE', #56549, #63544, #9080 ) ;
#86978=EDGE_CURVE ( 'NONE', #2021, #35739, #88709, .T. ) ;
#86991=ORIENTED_EDGE ( 'NONE', *, *, #7243, .F. ) ;
#86996=EDGE_LOOP ( 'NONE', ( #7800, #5677, #3613, #47238 ) ) ;
#87010=ORIENTED_EDGE ( 'NONE', *, *, #76713, .T. ) ;
#87018=VERTEX_POINT ( 'NONE', #13207 ) ;
#87049=EDGE_CURVE ( 'NONE', #39787, #63379, #58398, .T. ) ;
#87051=DIRECTION ( 'NONE',  ( 0.000000000000000000, 1.000000000000000000, 0.000000000000000000 ) ) ;
#87056=AXIS2_PLACEMENT_3D ( 'NONE', #11495, #40536, #48012 ) ;
#87063=CARTESIAN_POINT ( 'NONE',  ( -7.116235062956296709, -80.68325857818734903, -3.749999999999999556 ) ) ;
#87064=CARTESIAN_POINT ( 'NONE',  ( 45.14529252227820422, 61.69856644711347826, -8.000000000000000000 ) ) ;
#87078=CARTESIAN_POINT ( 'NONE',  ( -5.999999999999994671, 43.00000000000000000, 6.500000000000000888 ) ) ;
#87080=ORIENTED_EDGE ( 'NONE', *, *, #51720, .F. ) ;
#87087=DIRECTION ( 'NONE',  ( -0.06975647374412567714, -0.9975640502598243087, 0.000000000000000000 ) ) ;
#87091=DIRECTION ( 'NONE',  ( 0.000000000000000000, -1.000000000000000000, 0.000000000000000000 ) ) ;
#87118=CARTESIAN_POINT ( 'NONE',  ( 11.20666413564249453, -56.81049121600103291, 3.750000000000000000 ) ) ;
#87127=ORIENTED_EDGE ( 'NONE', *, *, #84746, .T. ) ;
#87128=FACE_OUTER_BOUND ( 'NONE', #20867, .T. ) ;
#87136=EDGE_CURVE ( 'NONE', #55430, #32382, #31157, .T. ) ;
#87137=EDGE_CURVE ( 'NONE', #89183, #74673, #2566, .T. ) ;
#87151=CARTESIAN_POINT ( 'NONE',  ( -8.218815441141973821, -9.362071622911987134, -4.000000000000000000 ) ) ;
#87154=CARTESIAN_POINT ( 'NONE',  ( 18.00000000000000000, 84.07179676972448590, 3.750000000000000000 ) ) ;
#87167=FACE_OUTER_BOUND ( 'NONE', #34001, .T. ) ;
#87169=UNCERTAINTY_MEASURE_WITH_UNIT (LENGTH_MEASURE( 1.000000000000000082E-05 ), #814, 'distance_accuracy_value', 'NONE');
#87170=EDGE_CURVE ( 'NONE', #83825, #26872, #74700, .T. ) ;
#87177=CARTESIAN_POINT ( 'NONE',  ( 4.400664535130860422, -1.180071741297640253, 3.750000000000001776 ) ) ;
#87184=LINE ( 'NONE', #95172, #9679 ) ;
#87187=FACE_OUTER_BOUND ( 'NONE', #92923, .T. ) ;
#87189=VERTEX_POINT ( 'NONE', #37218 ) ;
#87208=DIRECTION ( 'NONE',  ( -1.000000000000000000, 0.000000000000000000, 0.000000000000000000 ) ) ;
#87216=( NAMED_UNIT ( * ) SI_UNIT ( $, .STERADIAN. ) SOLID_ANGLE_UNIT ( ) );
#87220=STYLED_ITEM ( 'NONE', ( #58928 ), #30569 ) ;
#87223=ORIENTED_EDGE ( 'NONE', *, *, #54030, .T. ) ;
#87248=DIRECTION ( 'NONE',  ( -1.483861936729427615E-16, 1.000000000000000000, 0.000000000000000000 ) ) ;
#87257=CIRCLE ( 'NONE', #15430, 0.2500000000000002220 ) ;
#87258=CARTESIAN_POINT ( 'NONE',  ( -11.26637474388419591, 89.93360374965293147, 6.408881440111466432 ) ) ;
#87260=AXIS2_PLACEMENT_3D ( 'NONE', #82596, #30078, #12615 ) ;
#87262=EDGE_CURVE ( 'NONE', #9146, #71617, #47268, .T. ) ;
#87263=ORIENTED_EDGE ( 'NONE', *, *, #68208, .F. ) ;
#87270=( LENGTH_UNIT ( ) NAMED_UNIT ( * ) SI_UNIT ( .MILLI., .METRE. ) );
#87274=CARTESIAN_POINT ( 'NONE',  ( 4.441314631470126173, -2.693011450497559078, 3.749999999999999556 ) ) ;
#87283=CARTESIAN_POINT ( 'NONE',  ( -8.669785729375572458, 87.01784090252159842, -4.324025984537457568 ) ) ;
#87291=ORIENTED_EDGE ( 'NONE', *, *, #59622, .F. ) ;
#87292=( NAMED_UNIT ( * ) PLANE_ANGLE_UNIT ( ) SI_UNIT ( $, .RADIAN. ) );
#87293=EDGE_CURVE ( 'NONE', #92445, #21081, #15333, .T. ) ;
#87300=LINE ( 'NONE', #86822, #9766 ) ;
#87305=CARTESIAN_POINT ( 'NONE',  ( 4.469999999999999751, 0.000000000000000000, -3.750000000000000000 ) ) ;
#87332=CIRCLE ( 'NONE', #25127, 0.2499999999999999722 ) ;
#87333=CARTESIAN_POINT ( 'NONE',  ( -4.250000000000000000, 10.25000000000000000, -3.750000000000000000 ) ) ;
#87338=MECHANICAL_DESIGN_GEOMETRIC_PRESENTATION_REPRESENTATION('',(#10692),#49007);
#87340=CARTESIAN_POINT ( 'NONE',  ( -10.44999999999999751, 99.99999999999998579, 8.000000000000000000 ) ) ;
#87371=CARTESIAN_POINT ( 'NONE',  ( -6.732636091893172470, -88.11213685669366669, -4.000000000000000000 ) ) ;
#87379=ORIENTED_EDGE ( 'NONE', *, *, #98045, .F. ) ;
#87409=CARTESIAN_POINT ( 'NONE',  ( -4.259797195126492575, -13.81744876717405468, -2.750000000000806466 ) ) ;
#87412=DIRECTION ( 'NONE',  ( -1.000000000000000000, 0.000000000000000000, 0.000000000000000000 ) ) ;
#87414=CARTESIAN_POINT ( 'NONE',  ( 5.930070213854097716, -28.64748318935870941, -4.000000000000000000 ) ) ;
#87428=DIRECTION ( 'NONE',  ( -0.000000000000000000, -0.000000000000000000, 1.000000000000000000 ) ) ;
#87437=VERTEX_POINT ( 'NONE', #17171 ) ;
#87438=CARTESIAN_POINT ( 'NONE',  ( 18.00000000000000355, 77.07179676972445748, 6.500000000000000888 ) ) ;
#87447=ORIENTED_EDGE ( 'NONE', *, *, #84512, .F. ) ;
#87452=VERTEX_POINT ( 'NONE', #69667 ) ;
#87456=CARTESIAN_POINT ( 'NONE',  ( -6.000000000000000000, 78.07179676972447169, -6.500000000000000888 ) ) ;
#87463=CARTESIAN_POINT ( 'NONE',  ( -11.48781033751606095, -88.26659283070991080, -3.750000000000000000 ) ) ;
#87468=CIRCLE ( 'NONE', #47572, 4.250000000000001776 ) ;
#87481=ORIENTED_EDGE ( 'NONE', *, *, #72341, .F. ) ;
#87488=CARTESIAN_POINT ( 'NONE',  ( -6.356754967080489926, -50.93964766207074035, 2.500000000000000000 ) ) ;
#87498=DIRECTION ( 'NONE',  ( -0.000000000000000000, -0.000000000000000000, -1.000000000000000000 ) ) ;
#87533=FACE_OUTER_BOUND ( 'NONE', #16580, .T. ) ;
#87534=EDGE_CURVE ( 'NONE', #71973, #55896, #93663, .T. ) ;
#87543=FILL_AREA_STYLE_COLOUR ( '', #38451 ) ;
#87566=( NAMED_UNIT ( * ) SI_UNIT ( $, .STERADIAN. ) SOLID_ANGLE_UNIT ( ) );
#87574=DIRECTION ( 'NONE',  ( 1.000000000000000000, 0.000000000000000000, 0.000000000000000000 ) ) ;
#87580=AXIS2_PLACEMENT_3D ( 'NONE', #95795, #74249, #20779 ) ;
#87589=EDGE_CURVE ( 'NONE', #77672, #59059, #58551, .T. ) ;
#87590=VECTOR ( 'NONE', #62363, 1000.000000000000000 ) ;
#87594=ORIENTED_EDGE ( 'NONE', *, *, #85182, .F. ) ;
#87596=ORIENTED_EDGE ( 'NONE', *, *, #18553, .F. ) ;
#87599=CIRCLE ( 'NONE', #14179, 0.2500000000000002220 ) ;
#87608=CARTESIAN_POINT ( 'NONE',  ( 11.13639359202192303, -94.02695735605159655, 4.000000000000000000 ) ) ;
#87612=EDGE_CURVE ( 'NONE', #89183, #62473, #2674, .T. ) ;
#87614=CARTESIAN_POINT ( 'NONE',  ( -47.22560975609754053, 37.78048780487799263, -8.000000000000000000 ) ) ;
#87615=CARTESIAN_POINT ( 'NONE',  ( -6.867502880612995853, -58.37510853847093983, 3.749999999999999556 ) ) ;
#87623=CARTESIAN_POINT ( 'NONE',  ( 11.61481287315787370, -90.96947208220468895, -3.750000000000001776 ) ) ;
#87627=CARTESIAN_POINT ( 'NONE',  ( 3.969999999999999751, 36.75000000000000000, 2.750000000000000000 ) ) ;
#87630=PLANE ( 'NONE',  #96808 ) ;
#87631=ORIENTED_EDGE ( 'NONE', *, *, #54030, .F. ) ;
#87664=CARTESIAN_POINT ( 'NONE',  ( 4.474002695404426966, -3.767820133606233579, 3.750000000000001776 ) ) ;
#87673=AXIS2_PLACEMENT_3D ( 'NONE', #68053, #29534, #53031 ) ;
#87674=ORIENTED_EDGE ( 'NONE', *, *, #81450, .F. ) ;
#87675=CIRCLE ( 'NONE', #1502, 0.1000000000000001166 ) ;
#87676=CARTESIAN_POINT ( 'NONE',  ( 6.660464271194117103, -84.28715080306288598, 2.499999999999999556 ) ) ;
#87692=DIRECTION ( 'NONE',  ( -0.000000000000000000, -0.000000000000000000, -1.000000000000000000 ) ) ;
#87707=EDGE_CURVE ( 'NONE', #35180, #96723, #63332, .T. ) ;
#87719=EDGE_CURVE ( 'NONE', #93614, #89322, #88096, .T. ) ;
#87720=DIRECTION ( 'NONE',  ( 1.000000000000000000, 0.000000000000000000, 0.000000000000000000 ) ) ;
#87753=PLANE ( 'NONE',  #52038 ) ;
#87758=CARTESIAN_POINT ( 'NONE',  ( 0.000000000000000000, 40.74999999999999289, -4.250000000000000000 ) ) ;
#87762=DIRECTION ( 'NONE',  ( -1.000000000000000000, -1.483861936729430326E-16, 0.000000000000000000 ) ) ;
#87767=CARTESIAN_POINT ( 'NONE',  ( -3.888677573129737830, -8.267510245829294391, 2.750000000000000444 ) ) ;
#87772=CARTESIAN_POINT ( 'NONE',  ( -11.93818897418494984, 90.30657785595315090, -6.860068911468413688 ) ) ;
#87787=CARTESIAN_POINT ( 'NONE',  ( 9.261738776912691762, -15.50721619310700028, -4.000000000000000888 ) ) ;
#87790=PRESENTATION_STYLE_ASSIGNMENT (( #33790 ) ) ;
#87810=EDGE_CURVE ( 'NONE', #24577, #9027, #79625, .T. ) ;
#87820=DIRECTION ( 'NONE',  ( 1.000000000000000000, 0.000000000000000000, 0.000000000000000000 ) ) ;
#87824=ADVANCED_FACE ( 'NONE', ( #41643 ), #35088, .T. ) ;
#87825=EDGE_CURVE ( 'NONE', #34926, #94118, #23398, .T. ) ;
#87829=AXIS2_PLACEMENT_3D ( 'NONE', #25352, #63798, #32815 ) ;
#87837=VECTOR ( 'NONE', #10756, 1000.000000000000000 ) ;
#87840=CIRCLE ( 'NONE', #89419, 2.000000000000000888 ) ;
#87848=EDGE_CURVE ( 'NONE', #82789, #981, #21819, .T. ) ;
#87849=VERTEX_POINT ( 'NONE', #19608 ) ;
#87850=CARTESIAN_POINT ( 'NONE',  ( 17.75000000000000000, 78.80384757729335377, -3.750000000000000444 ) ) ;
#87864=PRESENTATION_STYLE_ASSIGNMENT (( #88368 ) ) ;
#87867=PRESENTATION_STYLE_ASSIGNMENT (( #64858 ) ) ;
#87872=DIRECTION ( 'NONE',  ( -1.000000000000000000, 0.000000000000000000, 0.000000000000000000 ) ) ;
#87878=CARTESIAN_POINT ( 'NONE',  ( 6.935134328217578137, -80.57830137131843173, 2.750000000001609823 ) ) ;
#87881=DIRECTION ( 'NONE',  ( 0.000000000000000000, 1.000000000000000000, 0.000000000000000000 ) ) ;
#87889=SURFACE_STYLE_FILL_AREA ( #41449 ) ;
#87893=FACE_OUTER_BOUND ( 'NONE', #65815, .T. ) ;
#87898=CARTESIAN_POINT ( 'NONE',  ( 7.079515573063597245, -88.00917032380698402, -4.000000000000000000 ) ) ;
#87902=ADVANCED_FACE ( 'NONE', ( #34593 ), #65086, .F. ) ;
#87932=VECTOR ( 'NONE', #7624, 1000.000000000000000 ) ;
#87940=EDGE_CURVE ( 'NONE', #70662, #57827, #13480, .T. ) ;
#87944=PRESENTATION_STYLE_ASSIGNMENT (( #74412 ) ) ;
#87951=CARTESIAN_POINT ( 'NONE',  ( -8.029120018247418500, -1.061548449190519605, -3.750000000000000444 ) ) ;
#87968=DIRECTION ( 'NONE',  ( -0.000000000000000000, 0.000000000000000000, 1.000000000000000000 ) ) ;
#87986=ORIENTED_EDGE ( 'NONE', *, *, #51090, .F. ) ;
#87994=( NAMED_UNIT ( * ) PLANE_ANGLE_UNIT ( ) SI_UNIT ( $, .RADIAN. ) );
#87997=CARTESIAN_POINT ( 'NONE',  ( 8.629999999999991900, 70.25000000000000000, 6.500000000000000888 ) ) ;
#87998=ORIENTED_EDGE ( 'NONE', *, *, #48567, .F. ) ;
#88021=CYLINDRICAL_SURFACE ( 'NONE', #56578, 0.2500000000000002220 ) ;
#88032=CARTESIAN_POINT ( 'NONE',  ( 18.00000000000000000, 78.20644475923673156, -3.828778322547003121 ) ) ;
#88037=CARTESIAN_POINT ( 'NONE',  ( -18.89999999999999503, 92.00000000000000000, 7.750000000000000000 ) ) ;
#88038=CARTESIAN_POINT ( 'NONE',  ( -8.000000000000000000, 83.99999999999994316, -2.900000000000000799 ) ) ;
#88054=LINE ( 'NONE', #72072, #11612 ) ;
#88055=FACE_OUTER_BOUND ( 'NONE', #477, .T. ) ;
#88061=CARTESIAN_POINT ( 'NONE',  ( -13.22853281710847284, 91.00000000000000000, 7.999999999999996447 ) ) ;
#88072=SURFACE_SIDE_STYLE ('',( #58064 ) ) ;
#88073=ORIENTED_EDGE ( 'NONE', *, *, #21271, .T. ) ;
#88078=SURFACE_SIDE_STYLE ('',( #33593 ) ) ;
#88081=STYLED_ITEM ( 'NONE', ( #18328 ), #80489 ) ;
#88083=ORIENTED_EDGE ( 'NONE', *, *, #71498, .F. ) ;
#88086=ORIENTED_EDGE ( 'NONE', *, *, #27641, .F. ) ;
#88088=ORIENTED_EDGE ( 'NONE', *, *, #47195, .T. ) ;
#88092=SURFACE_STYLE_USAGE ( .BOTH. , #95099 ) ;
#88095=ADVANCED_FACE ( 'NONE', ( #24798 ), #68131, .T. ) ;
#88096=LINE ( 'NONE', #12106, #72887 ) ;
#88097=AXIS2_PLACEMENT_3D ( 'NONE', #16005, #1019, #30499 ) ;
#88101=ORIENTED_EDGE ( 'NONE', *, *, #92324, .T. ) ;
#88102=CARTESIAN_POINT ( 'NONE',  ( 11.13639359160540288, -94.02695735602790705, 3.750000000000000000 ) ) ;
#88106=CARTESIAN_POINT ( 'NONE',  ( -7.045329894599615450, -66.66420243593404393, 2.750000000000000000 ) ) ;
#88130=DIRECTION ( 'NONE',  ( 0.000000000000000000, -1.000000000000000000, 0.000000000000000000 ) ) ;
#88137=DIRECTION ( 'NONE',  ( -6.938893903907222067E-15, 1.000000000000000000, 0.000000000000000000 ) ) ;
#88142=CARTESIAN_POINT ( 'NONE',  ( 6.905582103719410725, -69.44843085160002261, -3.750000000000002220 ) ) ;
#88167=CARTESIAN_POINT ( 'NONE',  ( 6.655501998723816648, -69.44085999572126866, 2.500000000000000000 ) ) ;
#88169=ORIENTED_EDGE ( 'NONE', *, *, #80502, .T. ) ;
#88187=EDGE_CURVE ( 'NONE', #76621, #88425, #40943, .T. ) ;
#88190=ORIENTED_EDGE ( 'NONE', *, *, #63670, .T. ) ;
#88191=CYLINDRICAL_SURFACE ( 'NONE', #36362, 6.349999999999995204 ) ;
#88199=DIRECTION ( 'NONE',  ( 0.000000000000000000, 1.000000000000000000, -0.000000000000000000 ) ) ;
#88200=AXIS2_PLACEMENT_3D ( 'NONE', #94774, #970, #64261 ) ;
#88222=( BOUNDED_CURVE ( )  B_SPLINE_CURVE ( 3, ( #39082, #46088, #8092, #40558 ),
 .UNSPECIFIED., .F., .F. ) 
 B_SPLINE_CURVE_WITH_KNOTS ( ( 4, 4 ),
 ( 3.141592653589793116, 4.712388980384689674 ),
 .UNSPECIFIED. ) 
 CURVE ( )  GEOMETRIC_REPRESENTATION_ITEM ( )  RATIONAL_B_SPLINE_CURVE ( ( 1.000000000000000000, 0.8047378541243649375, 0.8047378541243649375, 1.000000000000000000 ) ) 
 REPRESENTATION_ITEM ( '' )  );
#88224=CARTESIAN_POINT ( 'NONE',  ( -6.982525766850297799, -88.11956318484570261, 3.750000000000000000 ) ) ;
#88244=TOROIDAL_SURFACE ( 'NONE', #33990, 4.190000000000001279, 0.2500000000000000000 ) ;
#88247=DIRECTION ( 'NONE',  ( 0.8070303256584299145, -0.5905099943842175847, 0.000000000000000000 ) ) ;
#88255=CARTESIAN_POINT ( 'NONE',  ( -3.750000000000000000, 10.00000000000000000, -2.500000000000000000 ) ) ;
#88256=VECTOR ( 'NONE', #2345, 1000.000000000000000 ) ;
#88259=CARTESIAN_POINT ( 'NONE',  ( 5.679672690684601122, -28.64560013356482315, 3.750000000000000000 ) ) ;
#88266=CARTESIAN_POINT ( 'NONE',  ( -6.030735014468242561, -39.80307827768279338, 2.750000000000000444 ) ) ;
#88274=UNCERTAINTY_MEASURE_WITH_UNIT (LENGTH_MEASURE( 1.000000000000000082E-05 ), #41169, 'distance_accuracy_value', 'NONE');
#88295=UNCERTAINTY_MEASURE_WITH_UNIT (LENGTH_MEASURE( 1.000000000000000082E-05 ), #32216, 'distance_accuracy_value', 'NONE');
#88296=TOROIDAL_SURFACE ( 'NONE', #11639, 1.750000000000000888, 0.2500000000000000000 ) ;
#88299=DIRECTION ( 'NONE',  ( 0.000000000000000000, 0.000000000000000000, 1.000000000000000000 ) ) ;
#88300=EDGE_CURVE ( 'NONE', #82789, #25872, #50221, .T. ) ;
#88306=DIRECTION ( 'NONE',  ( -0.000000000000000000, -0.000000000000000000, -1.000000000000000000 ) ) ;
#88310=CARTESIAN_POINT ( 'NONE',  ( 4.145753578647971338, -0.8370341202350775056, -2.500000000000000000 ) ) ;
#88335=ORIENTED_EDGE ( 'NONE', *, *, #25755, .T. ) ;
#88351=ORIENTED_EDGE ( 'NONE', *, *, #63202, .T. ) ;
#88367=VECTOR ( 'NONE', #10400, 1000.000000000000000 ) ;
#88368=SURFACE_STYLE_USAGE ( .BOTH. , #4393 ) ;
#88383=FACE_BOUND ( 'NONE', #80702, .T. ) ;
#88385=ORIENTED_EDGE ( 'NONE', *, *, #19659, .T. ) ;
#88395=EDGE_CURVE ( 'NONE', #30537, #55012, #85763, .T. ) ;
#88397=CARTESIAN_POINT ( 'NONE',  ( -3.377759596008065746, -3.629459927035739497, -2.500000000000000000 ) ) ;
#88404=ORIENTED_EDGE ( 'NONE', *, *, #38181, .F. ) ;
#88406=CARTESIAN_POINT ( 'NONE',  ( 5.680373670945877862, -28.65980262290164049, -3.999999999987121413 ) ) ;
#88410=DIRECTION ( 'NONE',  ( 0.000000000000000000, 0.000000000000000000, -1.000000000000000000 ) ) ;
#88417=CARTESIAN_POINT ( 'NONE',  ( -3.750000000000000000, 10.25000000000000000, 2.750000000000000000 ) ) ;
#88425=VERTEX_POINT ( 'NONE', #21222 ) ;
#88442=CARTESIAN_POINT ( 'NONE',  ( 4.573751236700658751, -6.413519960483383464, 3.750000000000000000 ) ) ;
#88461=COLOUR_RGB ( '', 0.66274510, 0.83137255, 0.94901961) ;
#88475=CARTESIAN_POINT ( 'NONE',  ( -4.535014064373548592, -17.52590857053363393, 2.750000000000806466 ) ) ;
#88493=CARTESIAN_POINT ( 'NONE',  ( 6.878063601867475008, -66.29791949882819324, -3.750000000000000888 ) ) ;
#88496=ADVANCED_FACE ( 'NONE', ( #27724 ), #65218, .F. ) ;
#88510=SPHERICAL_SURFACE ( 'NONE', #55581, 0.2500000000000000000 ) ;
#88519=CARTESIAN_POINT ( 'NONE',  ( -6.822555938877875370, -84.39442183841866552, -2.500000000000000000 ) ) ;
#88522=DIRECTION ( 'NONE',  ( -0.000000000000000000, 0.000000000000000000, 1.000000000000000000 ) ) ;
#88536=DIRECTION ( 'NONE',  ( 0.000000000000000000, 0.000000000000000000, 1.000000000000000000 ) ) ;
#88538=ORIENTED_EDGE ( 'NONE', *, *, #48083, .F. ) ;
#88551=( LENGTH_UNIT ( ) NAMED_UNIT ( * ) SI_UNIT ( .MILLI., .METRE. ) );
#88557=CIRCLE ( 'NONE', #7200, 1.249999999999987121 ) ;
#88562=CARTESIAN_POINT ( 'NONE',  ( -8.099999999999999645, 75.73428692542562146, 2.900000000000000355 ) ) ;
#88568=FILL_AREA_STYLE_COLOUR ( '', #70149 ) ;
#88575=COLOUR_RGB ( '', 0.66274510, 0.83137255, 0.94901961) ;
#88580=ORIENTED_EDGE ( 'NONE', *, *, #76164, .T. ) ;
#88582=EDGE_LOOP ( 'NONE', ( #24898, #33870, #24885 ) ) ;
#88588=CARTESIAN_POINT ( 'NONE',  ( -4.250000000000000000, 78.07179676972445748, 6.500000000000000888 ) ) ;
#88589=EDGE_CURVE ( 'NONE', #32382, #92377, #13882, .T. ) ;
#88590=DIRECTION ( 'NONE',  ( 1.927470528863119542E-16, -1.000000000000000000, -0.000000000000000000 ) ) ;
#88603=CARTESIAN_POINT ( 'NONE',  ( 5.129999999999995453, 43.00000000000000000, 6.250000000000000000 ) ) ;
#88630=CARTESIAN_POINT ( 'NONE',  ( -10.60841303226387033, -98.07605699796263821, -3.999999999999994671 ) ) ;
#88633=DIRECTION ( 'NONE',  ( -1.000000000000000000, 0.000000000000000000, 0.000000000000000000 ) ) ;
#88634=AXIS2_PLACEMENT_3D ( 'NONE', #35862, #66855, #66350 ) ;
#88636=SURFACE_STYLE_USAGE ( .BOTH. , #27642 ) ;
#88651=CARTESIAN_POINT ( 'NONE',  ( 4.903136312256997087, -13.39483660680936339, 2.750000000000000000 ) ) ;
#88670=PRODUCT_DEFINITION_FORMATION_WITH_SPECIFIED_SOURCE ( 'ANY', '', #36462, .NOT_KNOWN. ) ;
#88674=SURFACE_SIDE_STYLE ('',( #27678 ) ) ;
#88683=CARTESIAN_POINT ( 'NONE',  ( 8.776446609406717059, 70.10355339059326241, -6.500000000000001776 ) ) ;
#88684=ORIENTED_EDGE ( 'NONE', *, *, #5334, .F. ) ;
#88685=SURFACE_STYLE_USAGE ( .BOTH. , #11216 ) ;
#88687=VERTEX_POINT ( 'NONE', #37713 ) ;
#88693=AXIS2_PLACEMENT_3D ( 'NONE', #59609, #76956, #69465 ) ;
#88707=CIRCLE ( 'NONE', #946, 0.2500000000000002220 ) ;
#88709=LINE ( 'NONE', #89207, #26504 ) ;
#88710=ORIENTED_EDGE ( 'NONE', *, *, #34885, .F. ) ;
#88712=FILL_AREA_STYLE_COLOUR ( '', #67084 ) ;
#88714=FACE_OUTER_BOUND ( 'NONE', #35091, .T. ) ;
#88725=DIRECTION ( 'NONE',  ( -0.000000000000000000, -0.000000000000000000, -1.000000000000000000 ) ) ;
#88726=DIRECTION ( 'NONE',  ( 1.000000000000000000, 0.000000000000000000, 0.000000000000000000 ) ) ;
#88733=CIRCLE ( 'NONE', #12088, 0.5000000000000000000 ) ;
#88735=CARTESIAN_POINT ( 'NONE',  ( -9.000000000000001776, 80.99999999999994316, 0.000000000000000000 ) ) ;
#88738=ADVANCED_FACE ( 'NONE', ( #29690 ), #52210, .T. ) ;
#88740=AXIS2_PLACEMENT_3D ( 'NONE', #44190, #43702, #35711 ) ;
#88746=DIRECTION ( 'NONE',  ( 0.000000000000000000, -0.000000000000000000, 1.000000000000000000 ) ) ;
#88752=( NAMED_UNIT ( * ) PLANE_ANGLE_UNIT ( ) SI_UNIT ( $, .RADIAN. ) );
#88760=CARTESIAN_POINT ( 'NONE',  ( -7.116235074765046242, -80.68325706346374204, 2.750000000000000888 ) ) ;
#88766=CARTESIAN_POINT ( 'NONE',  ( -13.39911793698190223, 90.87255582226813999, -7.784798940734470207 ) ) ;
#88771=PRESENTATION_STYLE_ASSIGNMENT (( #41336 ) ) ;
#88784=( NAMED_UNIT ( * ) PLANE_ANGLE_UNIT ( ) SI_UNIT ( $, .RADIAN. ) );
#88791=ORIENTED_EDGE ( 'NONE', *, *, #67868, .F. ) ;
#88798=CARTESIAN_POINT ( 'NONE',  ( 8.979999999999991545, 21.00000000000000000, -2.899999999999999911 ) ) ;
#88805=DIRECTION ( 'NONE',  ( -0.000000000000000000, -1.000000000000000000, -0.000000000000000000 ) ) ;
#88814=ORIENTED_EDGE ( 'NONE', *, *, #34080, .F. ) ;
#88822=VERTEX_POINT ( 'NONE', #60199 ) ;
#88824=ORIENTED_EDGE ( 'NONE', *, *, #2294, .T. ) ;
#88833=AXIS2_PLACEMENT_3D ( 'NONE', #65460, #27468, #29924 ) ;
#88843=ORIENTED_EDGE ( 'NONE', *, *, #9359, .T. ) ;
#88880=DIRECTION ( 'NONE',  ( 1.000000000000000000, 0.000000000000000000, 0.000000000000000000 ) ) ;
#88898=DIRECTION ( 'NONE',  ( 1.049065152435176504E-16, -1.000000000000000000, 0.000000000000000000 ) ) ;
#88899=CARTESIAN_POINT ( 'NONE',  ( -10.77974636252767482, -96.52223143589499443, -4.000000000000000888 ) ) ;
#88901=CARTESIAN_POINT ( 'NONE',  ( -7.330068351210570654, -69.53589943318685584, 4.000000000000000000 ) ) ;
#88910=CARTESIAN_POINT ( 'NONE',  ( -18.89999999999999147, 99.74999999999998579, -8.000000000000000000 ) ) ;
#88920=ORIENTED_EDGE ( 'NONE', *, *, #21152, .T. ) ;
#88932=ORIENTED_EDGE ( 'NONE', *, *, #8490, .T. ) ;
#88935=CARTESIAN_POINT ( 'NONE',  ( 4.395886033851783559, -0.8422402087859571784, 3.750000000000000000 ) ) ;
#88958=AXIS2_PLACEMENT_3D ( 'NONE', #45574, #6589, #7597 ) ;
#88973=CARTESIAN_POINT ( 'NONE',  ( -7.116252256210342964, -80.68108970088772480, 2.499999999998790745 ) ) ;
#88975=CIRCLE ( 'NONE', #92194, 0.2500000000000002220 ) ;
#88980=AXIS2_PLACEMENT_3D ( 'NONE', #65295, #12309, #65792 ) ;
#88981=DIRECTION ( 'NONE',  ( 0.8070303256584298035, -0.5905099943842175847, 0.000000000000000000 ) ) ;
#88983=ADVANCED_FACE ( 'NONE', ( #85664 ), #34620, .T. ) ;
#88988=EDGE_CURVE ( 'NONE', #1670, #76760, #41015, .T. ) ;
#88991=LINE ( 'NONE', #26510, #90167 ) ;
#88994=DIRECTION ( 'NONE',  ( -1.000000000000000000, 0.000000000000000000, 0.000000000000000000 ) ) ;
#88995=ORIENTED_EDGE ( 'NONE', *, *, #87136, .F. ) ;
#89008=ORIENTED_EDGE ( 'NONE', *, *, #27556, .F. ) ;
#89016=DIRECTION ( 'NONE',  ( -1.000000000000000000, 0.000000000000000000, 0.000000000000000000 ) ) ;
#89019=PRESENTATION_STYLE_ASSIGNMENT (( #66011 ) ) ;
#89021=EDGE_LOOP ( 'NONE', ( #76073, #63401, #41476, #445 ) ) ;
#89022=COLOUR_RGB ( '', 0.72549020, 0.75294118, 0.79215686) ;
#89024=FACE_OUTER_BOUND ( 'NONE', #84299, .T. ) ;
#89054=CARTESIAN_POINT ( 'NONE',  ( 14.99999999999997868, 80.07179676972448590, 4.250000000000000000 ) ) ;
#89066=VERTEX_POINT ( 'NONE', #18644 ) ;
#89073=EDGE_CURVE ( 'NONE', #52137, #80996, #9171, .T. ) ;
#89076=VERTEX_POINT ( 'NONE', #9668 ) ;
#89089=CIRCLE ( 'NONE', #66690, 0.09999999999999939493 ) ;
#89099=( NAMED_UNIT ( * ) SI_UNIT ( $, .STERADIAN. ) SOLID_ANGLE_UNIT ( ) );
#89105=DIRECTION ( 'NONE',  ( 0.7808688094430307203, -0.6246950475544238435, 0.000000000000000000 ) ) ;
#89111=AXIS2_PLACEMENT_3D ( 'NONE', #67282, #23278, #59765 ) ;
#89122=CARTESIAN_POINT ( 'NONE',  ( 0.000000000000000000, 0.000000000000000000, -4.000000000000000000 ) ) ;
#89124=DIRECTION ( 'NONE',  ( 0.000000000000000000, 0.000000000000000000, -1.000000000000000000 ) ) ;
#89131=CARTESIAN_POINT ( 'NONE',  ( -11.48880622970674636, -88.23206844530574244, -3.750000000000000000 ) ) ;
#89135=CARTESIAN_POINT ( 'NONE',  ( -3.750000000000000000, 36.75000000000000000, -2.750000000000000000 ) ) ;
#89157=EDGE_CURVE ( 'NONE', #3713, #61040, #47410, .T. ) ;
#89160=CARTESIAN_POINT ( 'NONE',  ( 4.191187596055478082, -2.692365942001591517, 2.500000000000000000 ) ) ;
#89162=ORIENTED_EDGE ( 'NONE', *, *, #66853, .T. ) ;
#89179=COLOUR_RGB ( '', 0.09019608, 0.27058824, 0.51372549) ;
#89180=CARTESIAN_POINT ( 'NONE',  ( 8.879999999999991900, 69.99999999999998579, -6.250000000000000000 ) ) ;
#89183=VERTEX_POINT ( 'NONE', #81103 ) ;
#89188=VECTOR ( 'NONE', #25630, 1000.000000000000114 ) ;
#89189=DIRECTION ( 'NONE',  ( -0.000000000000000000, 0.000000000000000000, 1.000000000000000000 ) ) ;
#89192=EDGE_CURVE ( 'NONE', #47751, #18983, #4330, .T. ) ;
#89207=CARTESIAN_POINT ( 'NONE',  ( -19.96637108136584260, 47.61387035396268885, -3.000000000000000000 ) ) ;
#89209=LINE ( 'NONE', #36210, #66860 ) ;
#89211=DIRECTION ( 'NONE',  ( -1.000000000000000000, 0.000000000000000000, 0.000000000000000000 ) ) ;
#89216=FACE_OUTER_BOUND ( 'NONE', #11017, .T. ) ;
#89220=STYLED_ITEM ( 'NONE', ( #15147 ), #3431 ) ;
#89226=DIRECTION ( 'NONE',  ( 0.000000000000000000, -0.000000000000000000, 1.000000000000000000 ) ) ;
#89237=VERTEX_POINT ( 'NONE', #4140 ) ;
#89247=CARTESIAN_POINT ( 'NONE',  ( 12.99999999999999822, 75.00000000000000000, -8.525133428036872019 ) ) ;
#89252=( GEOMETRIC_REPRESENTATION_CONTEXT ( 3 ) GLOBAL_UNCERTAINTY_ASSIGNED_CONTEXT ( ( #12296 ) ) GLOBAL_UNIT_ASSIGNED_CONTEXT ( ( #72569, #51064, #5587 ) ) REPRESENTATION_CONTEXT ( 'NONE', 'WORKASPACE' ) );
#89257=ORIENTED_EDGE ( 'NONE', *, *, #15294, .T. ) ;
#89262=DIRECTION ( 'NONE',  ( -2.569960705150826877E-16, 1.000000000000000000, -0.000000000000000000 ) ) ;
#89301=VECTOR ( 'NONE', #61929, 1000.000000000000000 ) ;
#89302=FILL_AREA_STYLE_COLOUR ( '', #11023 ) ;
#89313=EDGE_CURVE ( 'NONE', #18983, #24454, #9762, .T. ) ;
#89316=ADVANCED_FACE ( 'NONE', ( #95113 ), #68205, .T. ) ;
#89322=VERTEX_POINT ( 'NONE', #49607 ) ;
#89340=CARTESIAN_POINT ( 'NONE',  ( -13.77612262535527954, 90.93158326518027934, -7.883772450803742338 ) ) ;
#89346=AXIS2_PLACEMENT_3D ( 'NONE', #70982, #63461, #86475 ) ;
#89351=( LENGTH_UNIT ( ) NAMED_UNIT ( * ) SI_UNIT ( .MILLI., .METRE. ) );
#89359=CARTESIAN_POINT ( 'NONE',  ( -11.80960303780298482, 90.32667112043513669, -7.004222671090198027 ) ) ;
#89363=DIRECTION ( 'NONE',  ( 0.000000000000000000, 0.000000000000000000, 1.000000000000000000 ) ) ;
#89367=ORIENTED_EDGE ( 'NONE', *, *, #47800, .F. ) ;
#89376=ORIENTED_EDGE ( 'NONE', *, *, #14001, .T. ) ;
#89379=CARTESIAN_POINT ( 'NONE',  ( -7.116252256160142231, -80.68108970088715637, -2.749999999999193978 ) ) ;
#89388=CARTESIAN_POINT ( 'NONE',  ( -11.26386101273689988, -65.37750071423508302, -4.000000000000000888 ) ) ;
#89392=DIRECTION ( 'NONE',  ( -1.000000000000000000, 0.000000000000000000, 0.000000000000000000 ) ) ;
#89406=VERTEX_POINT ( 'NONE', #76562 ) ;
#89419=AXIS2_PLACEMENT_3D ( 'NONE', #14914, #7414, #30375 ) ;
#89424=ORIENTED_EDGE ( 'NONE', *, *, #51385, .F. ) ;
#89427=PRESENTATION_STYLE_ASSIGNMENT (( #81918 ) ) ;
#89429=DIRECTION ( 'NONE',  ( 0.000000000000000000, -1.000000000000000000, 0.000000000000000000 ) ) ;
#89442=AXIS2_PLACEMENT_3D ( 'NONE', #6245, #14751, #46218 ) ;
#89451=CARTESIAN_POINT ( 'NONE',  ( 6.879999999999995453, 70.25000000000000000, 6.250000000000000000 ) ) ;
#89466=DIRECTION ( 'NONE',  ( 1.000000000000000000, 0.000000000000000000, 0.000000000000000000 ) ) ;
#89468=EDGE_LOOP ( 'NONE', ( #29774, #27362, #33451, #96453 ) ) ;
#89469=AXIS2_PLACEMENT_3D ( 'NONE', #17238, #62217, #78211 ) ;
#89471=CARTESIAN_POINT ( 'NONE',  ( 7.079515573063599021, -88.00917032380691296, 4.000000000000000000 ) ) ;
#89473=DIRECTION ( 'NONE',  ( -1.000000000000000000, 0.000000000000000000, 0.000000000000000000 ) ) ;
#89476=UNCERTAINTY_MEASURE_WITH_UNIT (LENGTH_MEASURE( 1.000000000000000082E-05 ), #86410, 'distance_accuracy_value', 'NONE');
#89485=CARTESIAN_POINT ( 'NONE',  ( 6.930493939446634499, -71.55570417525920845, -3.750000000000000888 ) ) ;
#89486=ORIENTED_EDGE ( 'NONE', *, *, #41696, .T. ) ;
#89494=( LENGTH_UNIT ( ) NAMED_UNIT ( * ) SI_UNIT ( .MILLI., .METRE. ) );
#89515=CYLINDRICAL_SURFACE ( 'NONE', #7328, 0.2500000000000002220 ) ;
#89519=EDGE_CURVE ( 'NONE', #22589, #72372, #84074, .T. ) ;
#89521=AXIS2_PLACEMENT_3D ( 'NONE', #49612, #89105, #80627 ) ;
#89528=CYLINDRICAL_SURFACE ( 'NONE', #76837, 0.2500000000000002220 ) ;
#89541=ADVANCED_FACE ( 'NONE', ( #44584 ), #15098, .F. ) ;
#89543=CARTESIAN_POINT ( 'NONE',  ( -4.262581422817185661, -13.85606188144533846, -4.000000000000000888 ) ) ;
#89550=PRESENTATION_STYLE_ASSIGNMENT (( #67047 ) ) ;
#89554=DIRECTION ( 'NONE',  ( 0.000000000000000000, 0.000000000000000000, -1.000000000000000000 ) ) ;
#89557=EDGE_CURVE ( 'NONE', #84748, #3599, #7561, .T. ) ;
#89558=CIRCLE ( 'NONE', #86354, 0.09999999999999982514 ) ;
#89561=ORIENTED_EDGE ( 'NONE', *, *, #96999, .T. ) ;
#89563=ORIENTED_EDGE ( 'NONE', *, *, #58707, .F. ) ;
#89573=ORIENTED_EDGE ( 'NONE', *, *, #85707, .T. ) ;
#89582=AXIS2_PLACEMENT_3D ( 'NONE', #32792, #18300, #79779 ) ;
#89595=CARTESIAN_POINT ( 'NONE',  ( -6.607088789283611874, -50.94270388117418946, 3.750000000000000000 ) ) ;
#89617=FACE_OUTER_BOUND ( 'NONE', #69956, .T. ) ;
#89619=CARTESIAN_POINT ( 'NONE',  ( 8.880000000000020322, 80.32179676972448590, -4.250000000000000000 ) ) ;
#89625=STYLED_ITEM ( 'NONE', ( #69133 ), #74243 ) ;
#89651=CIRCLE ( 'NONE', #89582, 0.2500000000000002220 ) ;
#89653=CARTESIAN_POINT ( 'NONE',  ( -10.44999999999999751, 99.99999999999998579, -8.000000000000000000 ) ) ;
#89655=ORIENTED_EDGE ( 'NONE', *, *, #40114, .F. ) ;
#89657=SURFACE_SIDE_STYLE ('',( #81653 ) ) ;
#89686=COLOUR_RGB ( '', 0.09019608, 0.27058824, 0.51372549) ;
#89694=AXIS2_PLACEMENT_3D ( 'NONE', #42032, #96008, #41543 ) ;
#89706=ORIENTED_EDGE ( 'NONE', *, *, #96135, .T. ) ;
#89713=DIRECTION ( 'NONE',  ( -0.000000000000000000, -0.000000000000000000, -1.000000000000000000 ) ) ;
#89720=CARTESIAN_POINT ( 'NONE',  ( -18.89999999999999503, 92.00000000000000000, 8.000000000000000000 ) ) ;
#89723=ORIENTED_EDGE ( 'NONE', *, *, #36933, .T. ) ;
#89746=CARTESIAN_POINT ( 'NONE',  ( -10.17588876012473520, 89.26462023800682744, -5.905476706514950713 ) ) ;
#89748=AXIS2_PLACEMENT_3D ( 'NONE', #55036, #15101, #45577 ) ;
#89755=CARTESIAN_POINT ( 'NONE',  ( 10.93147959982391448, -92.98161664597374454, -4.000000000000000000 ) ) ;
#89763=CYLINDRICAL_SURFACE ( 'NONE', #40201, 0.2500000000000002220 ) ;
#89765=( GEOMETRIC_REPRESENTATION_CONTEXT ( 3 ) GLOBAL_UNCERTAINTY_ASSIGNED_CONTEXT ( ( #32090 ) ) GLOBAL_UNIT_ASSIGNED_CONTEXT ( ( #71913, #55941, #79428 ) ) REPRESENTATION_CONTEXT ( 'NONE', 'WORKASPACE' ) );
#89770=VECTOR ( 'NONE', #61934, 1000.000000000000000 ) ;
#89773=SPHERICAL_SURFACE ( 'NONE', #63618, 0.2500000000000000000 ) ;
#89783=CARTESIAN_POINT ( 'NONE',  ( 4.669717816207066718, -13.81568353606978761, -2.500000000000000888 ) ) ;
#89797=VECTOR ( 'NONE', #97846, 999.9999999999998863 ) ;
#89827=CARTESIAN_POINT ( 'NONE',  ( -13.78969293960296305, 90.90480785988455636, -7.820272038271530057 ) ) ;
#89831=ADVANCED_FACE ( 'NONE', ( #25551 ), #56043, .F. ) ;
#89846=CARTESIAN_POINT ( 'NONE',  ( -13.34727560011345382, 90.86036091889430111, -7.765078796629374835 ) ) ;
#89861=MECHANICAL_DESIGN_GEOMETRIC_PRESENTATION_REPRESENTATION('',(#16438),#29192);
#89872=ADVANCED_FACE ( 'NONE', ( #32028 ), #55032, .T. ) ;
#89881=DIRECTION ( 'NONE',  ( 0.000000000000000000, -1.000000000000000000, 0.000000000000000000 ) ) ;
#89904=CIRCLE ( 'NONE', #11678, 0.2500000000000002220 ) ;
#89916=CARTESIAN_POINT ( 'NONE',  ( 4.395886034088992034, -0.8422402087801302839, 4.000000000000000000 ) ) ;
#89917=DIRECTION ( 'NONE',  ( 1.000000000000000000, 0.000000000000000000, 0.000000000000000000 ) ) ;
#89918=( NAMED_UNIT ( * ) PLANE_ANGLE_UNIT ( ) SI_UNIT ( $, .RADIAN. ) );
#89926=ORIENTED_EDGE ( 'NONE', *, *, #1499, .T. ) ;
#89954=CARTESIAN_POINT ( 'NONE',  ( 11.18664512657591459, -81.61943089668858420, 4.000000000000000000 ) ) ;
#89958=DIRECTION ( 'NONE',  ( -0.000000000000000000, -0.000000000000000000, 1.000000000000000000 ) ) ;
#89963=VECTOR ( 'NONE', #98730, 1000.000000000000114 ) ;
#89965=CIRCLE ( 'NONE', #91621, 4.000000000000001776 ) ;
#89970=CARTESIAN_POINT ( 'NONE',  ( -13.77612262535527954, 90.93158326518027934, -7.883772450803742338 ) ) ;
#89973=AXIS2_PLACEMENT_3D ( 'NONE', #4752, #66725, #59209 ) ;
#89987=ORIENTED_EDGE ( 'NONE', *, *, #81638, .F. ) ;
#90022=EDGE_CURVE ( 'NONE', #39466, #71601, #88991, .T. ) ;
#90024=( NAMED_UNIT ( * ) SI_UNIT ( $, .STERADIAN. ) SOLID_ANGLE_UNIT ( ) );
#90029=CARTESIAN_POINT ( 'NONE',  ( -7.072388532740516709, -84.40601219567591329, -3.750000000000806022 ) ) ;
#90030=ORIENTED_EDGE ( 'NONE', *, *, #17762, .F. ) ;
#90035=LINE ( 'NONE', #6058, #97049 ) ;
#90037=DIRECTION ( 'NONE',  ( 1.000000000000000000, 0.000000000000000000, 0.000000000000000000 ) ) ;
#90047=ORIENTED_EDGE ( 'NONE', *, *, #53064, .F. ) ;
#90071=ADVANCED_FACE ( 'NONE', ( #59979 ), #26290, .T. ) ;
#90082=( NAMED_UNIT ( * ) PLANE_ANGLE_UNIT ( ) SI_UNIT ( $, .RADIAN. ) );
#90104=( GEOMETRIC_REPRESENTATION_CONTEXT ( 3 ) GLOBAL_UNCERTAINTY_ASSIGNED_CONTEXT ( ( #75456 ) ) GLOBAL_UNIT_ASSIGNED_CONTEXT ( ( #47065, #55057, #18066 ) ) REPRESENTATION_CONTEXT ( 'NONE', 'WORKASPACE' ) );
#90112=DIRECTION ( 'NONE',  ( 0.000000000000000000, -1.000000000000000000, 0.000000000000000000 ) ) ;
#90146=LINE ( 'NONE', #80689, #27517 ) ;
#90152=DIRECTION ( 'NONE',  ( -1.000000000000000000, 0.000000000000000000, 0.000000000000000000 ) ) ;
#90155=ORIENTED_EDGE ( 'NONE', *, *, #81605, .T. ) ;
#90156=DIRECTION ( 'NONE',  ( -0.000000000000000000, 0.000000000000000000, 1.000000000000000000 ) ) ;
#90167=VECTOR ( 'NONE', #57985, 1000.000000000000000 ) ;
#90170=EDGE_CURVE ( 'NONE', #31275, #73541, #71441, .T. ) ;
#90179=VECTOR ( 'NONE', #96757, 1000.000000000000000 ) ;
#90180=DIRECTION ( 'NONE',  ( -1.000000000000000000, -1.049065152435176504E-16, 0.000000000000000000 ) ) ;
#90184=EDGE_CURVE ( 'NONE', #34829, #89237, #10923, .T. ) ;
#90187=AXIS2_PLACEMENT_3D ( 'NONE', #47927, #78928, #82869 ) ;
#90203=DIRECTION ( 'NONE',  ( -0.000000000000000000, -0.000000000000000000, -1.000000000000000000 ) ) ;
#90212=VERTEX_POINT ( 'NONE', #40944 ) ;
#90222=DIRECTION ( 'NONE',  ( -1.000000000000000000, 0.000000000000000000, 0.000000000000000000 ) ) ;
#90239=DIRECTION ( 'NONE',  ( 0.000000000000000000, 0.000000000000000000, 1.000000000000000000 ) ) ;
#90247=CARTESIAN_POINT ( 'NONE',  ( 11.29392812347916752, -89.88967135474473480, -4.000000000001793232 ) ) ;
#90257=ORIENTED_EDGE ( 'NONE', *, *, #42717, .T. ) ;
#90259=AXIS2_PLACEMENT_3D ( 'NONE', #3199, #54698, #33181 ) ;
#90260=LINE ( 'NONE', #69262, #63552 ) ;
#90269=DIRECTION ( 'NONE',  ( 0.000000000000000000, 0.000000000000000000, 1.000000000000000000 ) ) ;
#90276=MECHANICAL_DESIGN_GEOMETRIC_PRESENTATION_REPRESENTATION('',(#21640),#71102);
#90287=ORIENTED_EDGE ( 'NONE', *, *, #84704, .F. ) ;
#90290=EDGE_CURVE ( 'NONE', #66694, #25004, #69463, .T. ) ;
#90297=AXIS2_PLACEMENT_3D ( 'NONE', #8929, #70929, #23468 ) ;
#90301=CARTESIAN_POINT ( 'NONE',  ( -8.000000000000000000, 83.99999999999994316, 4.000000000000000000 ) ) ;
#90308=CARTESIAN_POINT ( 'NONE',  ( 4.380000000000002558, 1.019547802438462547, -3.750000000000000000 ) ) ;
#90322=CARTESIAN_POINT ( 'NONE',  ( 6.579634127946653699, -87.99828267815713900, -2.500000000000001332 ) ) ;
#90336=ORIENTED_EDGE ( 'NONE', *, *, #81160, .T. ) ;
#90338=CARTESIAN_POINT ( 'NONE',  ( 11.01793658010034704, -96.10624868222545558, 3.750000000000000444 ) ) ;
#90347=CARTESIAN_POINT ( 'NONE',  ( -7.079903288618116797, -69.52484394646381816, -2.750000000000000000 ) ) ;
#90355=FILL_AREA_STYLE ('',( #45870 ) ) ;
#90356=CARTESIAN_POINT ( 'NONE',  ( 8.629999999999991900, 70.25000000000000000, -6.500000000000000888 ) ) ;
#90372=UNCERTAINTY_MEASURE_WITH_UNIT (LENGTH_MEASURE( 1.000000000000000082E-05 ), #73522, 'distance_accuracy_value', 'NONE');
#90373=VECTOR ( 'NONE', #91153, 1000.000000000000000 ) ;
#90396=CARTESIAN_POINT ( 'NONE',  ( 0.4400000000000020006, 1.019547802438468986, -2.750000000000000000 ) ) ;
#90397=DIRECTION ( 'NONE',  ( -0.000000000000000000, -0.000000000000000000, -1.000000000000000000 ) ) ;
#90403=DIRECTION ( 'NONE',  ( 0.06975647374410356982, 0.9975640502598257520, -0.000000000000000000 ) ) ;
#90410=CYLINDRICAL_SURFACE ( 'NONE', #77053, 3.000000000000000888 ) ;
#90416=EDGE_CURVE ( 'NONE', #60398, #72885, #26405, .T. ) ;
#90428=CIRCLE ( 'NONE', #32913, 2.900000000000002576 ) ;
#90430=CARTESIAN_POINT ( 'NONE',  ( -5.809210876173504623, -36.07757871006354122, 2.500000000001614264 ) ) ;
#90434=CARTESIAN_POINT ( 'NONE',  ( 7.185089000015953964, -80.58569572050204499, -4.000000000000000000 ) ) ;
#90436=ORIENTED_EDGE ( 'NONE', *, *, #76203, .T. ) ;
#90446=CARTESIAN_POINT ( 'NONE',  ( -8.051738205446136831, 84.95449735710184314, 3.788866803286794038 ) ) ;
#90458=VECTOR ( 'NONE', #76252, 1000.000000000000000 ) ;
#90462=FACE_OUTER_BOUND ( 'NONE', #28774, .T. ) ;
#90498=CARTESIAN_POINT ( 'NONE',  ( 17.99999999999999645, 91.28723161455539525, 8.000000000000000000 ) ) ;
#90516=CARTESIAN_POINT ( 'NONE',  ( -5.811454672306065383, -36.11427488547452214, -3.750000000000000000 ) ) ;
#90522=FILL_AREA_STYLE ('',( #59045 ) ) ;
#90523=CARTESIAN_POINT ( 'NONE',  ( -10.91371419741714277, 89.69638457836573764, -6.151049038649611056 ) ) ;
#90527=AXIS2_PLACEMENT_3D ( 'NONE', #33618, #86651, #32652 ) ;
#90547=COLOUR_RGB ( '', 0.40784314, 0.44705882, 0.49803922) ;
#90556=ORIENTED_EDGE ( 'NONE', *, *, #33522, .F. ) ;
#90564=ORIENTED_EDGE ( 'NONE', *, *, #74292, .T. ) ;
#90593=CARTESIAN_POINT ( 'NONE',  ( -3.500000000000000444, -0.04521315095527938394, -3.750000000000000000 ) ) ;
#90595=CARTESIAN_POINT ( 'NONE',  ( 8.979619469809167143, 27.03494536863381015, -2.900000000000000799 ) ) ;
#90602=CARTESIAN_POINT ( 'NONE',  ( -4.000000000000000000, 36.75000000000000000, 4.000000000000000000 ) ) ;
#90607=DIRECTION ( 'NONE',  ( 0.000000000000000000, 0.000000000000000000, 1.000000000000000000 ) ) ;
#90619=CARTESIAN_POINT ( 'NONE',  ( 4.130000000000002558, 1.019547802438464545, -2.500000000000000000 ) ) ;
#90627=EDGE_CURVE ( 'NONE', #21427, #8937, #40657, .T. ) ;
#90640=CARTESIAN_POINT ( 'NONE',  ( -8.468251459920482560, -9.345277391848098247, 3.750000000000000000 ) ) ;
#90650=ORIENTED_EDGE ( 'NONE', *, *, #84161, .T. ) ;
#90652=ORIENTED_EDGE ( 'NONE', *, *, #27106, .T. ) ;
#90669=ADVANCED_FACE ( 'NONE', ( #33208 ), #53415, .F. ) ;
#90671=ORIENTED_EDGE ( 'NONE', *, *, #21031, .T. ) ;
#90677=DIRECTION ( 'NONE',  ( 1.049065152435176504E-16, -1.000000000000000000, 0.000000000000000000 ) ) ;
#90682=AXIS2_PLACEMENT_3D ( 'NONE', #7165, #29156, #90152 ) ;
#90684=EDGE_LOOP ( 'NONE', ( #19210, #51799, #29044, #26026 ) ) ;
#90700=( LENGTH_UNIT ( ) NAMED_UNIT ( * ) SI_UNIT ( .MILLI., .METRE. ) );
#90727=DIRECTION ( 'NONE',  ( -1.000000000000000000, 0.000000000000000000, 0.000000000000000000 ) ) ;
#90743=CARTESIAN_POINT ( 'NONE',  ( 8.959589291399149502, -9.312544548374205533, -4.000000000000000000 ) ) ;
#90747=AXIS2_PLACEMENT_3D ( 'NONE', #84411, #90403, #98449 ) ;
#90759=CIRCLE ( 'NONE', #14115, 0.1000000000000001166 ) ;
#90761=EDGE_LOOP ( 'NONE', ( #66615, #81722, #27059, #11860 ) ) ;
#90779=EDGE_CURVE ( 'NONE', #93614, #95526, #86562, .T. ) ;
#90786=ORIENTED_EDGE ( 'NONE', *, *, #92560, .T. ) ;
#90790=CYLINDRICAL_SURFACE ( 'NONE', #13735, 8.000000000000000000 ) ;
#90801=ORIENTED_EDGE ( 'NONE', *, *, #10850, .T. ) ;
#90810=CARTESIAN_POINT ( 'NONE',  ( 4.471356726113142166, -3.620120708367990492, -3.750000000000000888 ) ) ;
#90819=EDGE_CURVE ( 'NONE', #72372, #57586, #90146, .T. ) ;
#90822=COLOUR_RGB ( '', 0.08235294, 0.09019608, 0.10196078) ;
#90839=ORIENTED_EDGE ( 'NONE', *, *, #59271, .F. ) ;
#90840=TOROIDAL_SURFACE ( 'NONE', #19052, 0.5000000000000000000, 0.2500000000000000000 ) ;
#90848=DIRECTION ( 'NONE',  ( -1.000000000000000000, -0.000000000000000000, 0.000000000000000000 ) ) ;
#90856=DIRECTION ( 'NONE',  ( 1.000000000000000000, 0.000000000000000000, 0.000000000000000000 ) ) ;
#90871=EDGE_CURVE ( 'NONE', #26502, #37917, #73872, .T. ) ;
#90872=ADVANCED_FACE ( 'NONE', ( #20682 ), #94317, .T. ) ;
#90876=EDGE_CURVE ( 'NONE', #2021, #22085, #73763, .T. ) ;
#90893=( NAMED_UNIT ( * ) PLANE_ANGLE_UNIT ( ) SI_UNIT ( $, .RADIAN. ) );
#90898=CARTESIAN_POINT ( 'NONE',  ( 6.934035614004487869, -73.16521313705239038, 3.750000000000000000 ) ) ;
#90899=SURFACE_STYLE_USAGE ( .BOTH. , #60403 ) ;
#90900=DIRECTION ( 'NONE',  ( 0.000000000000000000, -0.000000000000000000, -1.000000000000000000 ) ) ;
#90930=CARTESIAN_POINT ( 'NONE',  ( -6.867320125584340573, -58.36821204062218982, 2.500000000000000000 ) ) ;
#90941=DIRECTION ( 'NONE',  ( 0.7808688094430307203, -0.6246950475544238435, 0.000000000000000000 ) ) ;
#90944=EDGE_CURVE ( 'NONE', #67494, #44503, #38669, .T. ) ;
#90973=DIRECTION ( 'NONE',  ( 1.224646799147353207E-16, 1.000000000000000000, 0.000000000000000000 ) ) ;
#90980=( NAMED_UNIT ( * ) SI_UNIT ( $, .STERADIAN. ) SOLID_ANGLE_UNIT ( ) );
#90981=TOROIDAL_SURFACE ( 'NONE', #47872, 10.65000000000000036, 0.2500000000000000000 ) ;
#90990=EDGE_CURVE ( 'NONE', #51712, #31750, #9986, .T. ) ;
#90993=DIRECTION ( 'NONE',  ( -0.000000000000000000, -0.000000000000000000, 1.000000000000000000 ) ) ;
#91010=CARTESIAN_POINT ( 'NONE',  ( -5.320324007939504440, -24.96642978971303961, -3.999999999999998224 ) ) ;
#91016=( NAMED_UNIT ( * ) SI_UNIT ( $, .STERADIAN. ) SOLID_ANGLE_UNIT ( ) );
#91017=CARTESIAN_POINT ( 'NONE',  ( -12.99123301834679900, 90.70871800849667466, -7.440805305833852579 ) ) ;
#91058=CARTESIAN_POINT ( 'NONE',  ( 0.000000000000000000, -97.00000000000000000, 4.000000000000000000 ) ) ;
#91062=CARTESIAN_POINT ( 'NONE',  ( -6.000000000000014211, 79.82179676972448590, 6.250000000000000000 ) ) ;
#91066=( LENGTH_UNIT ( ) NAMED_UNIT ( * ) SI_UNIT ( .MILLI., .METRE. ) );
#91069=DIRECTION ( 'NONE',  ( 0.000000000000000000, 0.000000000000000000, -1.000000000000000000 ) ) ;
#91077=EDGE_CURVE ( 'NONE', #7091, #49656, #30652, .T. ) ;
#91078=CARTESIAN_POINT ( 'NONE',  ( -13.80105244024794331, 90.89655890636515778, -7.750000000004162892 ) ) ;
#91083=ORIENTED_EDGE ( 'NONE', *, *, #45781, .T. ) ;
#91090=CARTESIAN_POINT ( 'NONE',  ( 6.879999999999995453, 43.00000000000000000, 6.250000000000000000 ) ) ;
#91092=FACE_OUTER_BOUND ( 'NONE', #23684, .T. ) ;
#91104=AXIS2_PLACEMENT_3D ( 'NONE', #67633, #31580, #83618 ) ;
#91109=UNCERTAINTY_MEASURE_WITH_UNIT (LENGTH_MEASURE( 1.000000000000000082E-05 ), #88551, 'distance_accuracy_value', 'NONE');
#91110=EDGE_CURVE ( 'NONE', #54251, #26502, #93102, .T. ) ;
#91131=ORIENTED_EDGE ( 'NONE', *, *, #96255, .T. ) ;
#91138=CARTESIAN_POINT ( 'NONE',  ( -10.91022435251843348, -52.91485255063418691, 4.000000000000000000 ) ) ;
#91147=VERTEX_POINT ( 'NONE', #55099 ) ;
#91150=DIRECTION ( 'NONE',  ( 0.000000000000000000, 0.000000000000000000, -1.000000000000000000 ) ) ;
#91151=ORIENTED_EDGE ( 'NONE', *, *, #66949, .T. ) ;
#91153=DIRECTION ( 'NONE',  ( -0.000000000000000000, -1.000000000000000000, -0.000000000000000000 ) ) ;
#91160=LINE ( 'NONE', #688, #78353 ) ;
#91173=TOROIDAL_SURFACE ( 'NONE', #48056, 0.5000000000000000000, 0.2500000000000000000 ) ;
#91175=( GEOMETRIC_REPRESENTATION_CONTEXT ( 3 ) GLOBAL_UNCERTAINTY_ASSIGNED_CONTEXT ( ( #94195 ) ) GLOBAL_UNIT_ASSIGNED_CONTEXT ( ( #43632, #31089, #62073 ) ) REPRESENTATION_CONTEXT ( 'NONE', 'WORKASPACE' ) );
#91179=SURFACE_STYLE_USAGE ( .BOTH. , #97734 ) ;
#91180=VERTEX_POINT ( 'NONE', #66051 ) ;
#91181=( LENGTH_UNIT ( ) NAMED_UNIT ( * ) SI_UNIT ( .MILLI., .METRE. ) );
#91188=DIRECTION ( 'NONE',  ( 1.000000000000000000, 0.000000000000000000, 0.000000000000000000 ) ) ;
#91192=LINE ( 'NONE', #53201, #24084 ) ;
#91205=DIRECTION ( 'NONE',  ( -0.000000000000000000, -0.000000000000000000, -1.000000000000000000 ) ) ;
#91207=( LENGTH_UNIT ( ) NAMED_UNIT ( * ) SI_UNIT ( .MILLI., .METRE. ) );
#91222=MECHANICAL_DESIGN_GEOMETRIC_PRESENTATION_REPRESENTATION('',(#78456),#54529);
#91229=DIRECTION ( 'NONE',  ( 0.000000000000000000, -1.000000000000000000, 0.000000000000000000 ) ) ;
#91238=CARTESIAN_POINT ( 'NONE',  ( 10.85665724876936089, -52.68265776531869449, -4.000000000000000000 ) ) ;
#91263=MECHANICAL_DESIGN_GEOMETRIC_PRESENTATION_REPRESENTATION('',(#11389),#33715);
#91267=FILL_AREA_STYLE ('',( #61261 ) ) ;
#91271=CIRCLE ( 'NONE', #3636, 1.249999999999987121 ) ;
#91284=CARTESIAN_POINT ( 'NONE',  ( 0.000000000000000000, 84.07179676972448590, 12.00000000000000000 ) ) ;
#91285=ORIENTED_EDGE ( 'NONE', *, *, #24332, .T. ) ;
#91289=CARTESIAN_POINT ( 'NONE',  ( -9.000000000000001776, 80.99999999999994316, 0.000000000000000000 ) ) ;
#91292=CIRCLE ( 'NONE', #40273, 10.65000000000026326 ) ;
#91314=VERTEX_POINT ( 'NONE', #5576 ) ;
#91318=CARTESIAN_POINT ( 'NONE',  ( 6.905507196098383815, -69.44000359822096868, -2.500000000000000000 ) ) ;
#91320=EDGE_CURVE ( 'NONE', #9418, #92281, #36051, .T. ) ;
#91336=SURFACE_STYLE_USAGE ( .BOTH. , #60346 ) ;
#91338=CARTESIAN_POINT ( 'NONE',  ( -10.32525428029501313, -40.46312579908686757, -4.000000000000000000 ) ) ;
#91346=DIRECTION ( 'NONE',  ( -0.000000000000000000, -1.000000000000000000, 0.000000000000000000 ) ) ;
#91347=LINE ( 'NONE', #23366, #43862 ) ;
#91362=DIRECTION ( 'NONE',  ( -1.000000000000000000, 0.000000000000000000, 0.000000000000000000 ) ) ;
#91389=SURFACE_STYLE_USAGE ( .BOTH. , #44896 ) ;
#91392=ORIENTED_EDGE ( 'NONE', *, *, #84249, .F. ) ;
#91400=CARTESIAN_POINT ( 'NONE',  ( -6.857531195348598452, -50.94829529698460391, -3.999999999999998224 ) ) ;
#91406=AXIS2_PLACEMENT_3D ( 'NONE', #9120, #26101, #86113 ) ;
#91425=ORIENTED_EDGE ( 'NONE', *, *, #24868, .T. ) ;
#91431=EDGE_CURVE ( 'NONE', #38057, #37189, #94023, .T. ) ;
#91440=ORIENTED_EDGE ( 'NONE', *, *, #4085, .F. ) ;
#91442=DIRECTION ( 'NONE',  ( 0.6246950475544238435, 0.7808688094430307203, 0.000000000000000000 ) ) ;
#91449=CARTESIAN_POINT ( 'NONE',  ( -12.99123301833645172, 90.70871800849351985, 7.440805305829000460 ) ) ;
#91455=CARTESIAN_POINT ( 'NONE',  ( 4.400664535130860422, -1.180071741297640253, -3.750000000000000888 ) ) ;
#91474=VECTOR ( 'NONE', #61659, 999.9999999999998863 ) ;
#91480=CARTESIAN_POINT ( 'NONE',  ( -3.750000000000000000, 78.07179676972445748, -4.000000000000000000 ) ) ;
#91481=FACE_OUTER_BOUND ( 'NONE', #13235, .T. ) ;
#91487=CIRCLE ( 'NONE', #49941, 0.2500000000000002220 ) ;
#91500=LINE ( 'NONE', #31472, #3267 ) ;
#91512=DIRECTION ( 'NONE',  ( -0.000000000000000000, 0.000000000000000000, 1.000000000000000000 ) ) ;
#91520=CARTESIAN_POINT ( 'NONE',  ( -7.037696229836970296, -86.26312365674226612, -4.000000000000000000 ) ) ;
#91538=ORIENTED_EDGE ( 'NONE', *, *, #12413, .T. ) ;
#91539=DIRECTION ( 'NONE',  ( 0.9975640502598243087, -0.06975647374412452528, 0.000000000000000000 ) ) ;
#91549=VERTEX_POINT ( 'NONE', #44540 ) ;
#91559=CIRCLE ( 'NONE', #69220, 1.249999999999987121 ) ;
#91561=EDGE_CURVE ( 'NONE', #55464, #80099, #57842, .T. ) ;
#91563=CARTESIAN_POINT ( 'NONE',  ( -8.000000000000000000, 80.99999999999994316, 0.000000000000000000 ) ) ;
#91588=PRESENTATION_STYLE_ASSIGNMENT (( #22112 ) ) ;
#91597=DIRECTION ( 'NONE',  ( 1.000000000000000000, 0.000000000000000000, 0.000000000000000000 ) ) ;
#91600=DIRECTION ( 'NONE',  ( -0.9961946980917453232, 0.08715574274766037244, 0.000000000000000000 ) ) ;
#91621=AXIS2_PLACEMENT_3D ( 'NONE', #65910, #20428, #64429 ) ;
#91623=FILL_AREA_STYLE_COLOUR ( '', #62093 ) ;
#91640=CARTESIAN_POINT ( 'NONE',  ( -11.48887051637748691, -88.22984412037381219, 3.750000000000000000 ) ) ;
#91655=DIRECTION ( 'NONE',  ( 0.000000000000000000, -0.000000000000000000, -1.000000000000000000 ) ) ;
#91660=DIRECTION ( 'NONE',  ( -1.000000000000000000, 0.000000000000000000, 0.000000000000000000 ) ) ;
#91674=PLANE ( 'NONE',  #72286 ) ;
#91675=CARTESIAN_POINT ( 'NONE',  ( -8.099999999999999645, 75.73428692542562146, 3.000000000000000000 ) ) ;
#91690=VERTEX_POINT ( 'NONE', #2523 ) ;
#91705=CYLINDRICAL_SURFACE ( 'NONE', #14015, 1.000000000000000888 ) ;
#91718=CARTESIAN_POINT ( 'NONE',  ( 4.629999999999991900, 76.07179676972444327, 4.250000000000000000 ) ) ;
#91722=FACE_BOUND ( 'NONE', #52662, .T. ) ;
#91723=CIRCLE ( 'NONE', #955, 0.09999999999999982514 ) ;
#91741=B_SPLINE_CURVE_WITH_KNOTS ( 'NONE', 3,
 ( #77897, #26370, #56869, #18391, #69920, #39911, #25895, #47889, #64360, #3387, #24920, #9912, #62391, #62896, #40414, #92899, #93889, #56394, #25417, #55901, #17901, #70414, #2918, #40901, #24430, #48384, #78886, #71402, #94376, #54894, #48870, #86881, #1934, #79382 ),
 .UNSPECIFIED., .F., .F.,
 ( 4, 2, 2, 2, 2, 2, 2, 2, 2, 2, 2, 2, 2, 2, 2, 2, 4 ),
 ( -5.999999999205076248E-08, 0.0003894208653645889824, 0.0007789017307291700191, 0.001557863461458290893, 0.003115786922916491657, 0.006231633845832851987, 0.01246332769166561168, 0.01869502153749837137, 0.02492671538333113279, 0.03739010307499662095, 0.04985349076666211604, 0.06231687845832762501, 0.07478026614999312705, 0.08724365384165863602, 0.09347534768749138356, 0.09659119461040775734, 0.09970704153332413111 ),
 .UNSPECIFIED. ) ;
#91742=CARTESIAN_POINT ( 'NONE',  ( 11.33987066887527284, -87.82218667483482477, -3.750000000000000000 ) ) ;
#91752=EDGE_LOOP ( 'NONE', ( #7227, #31528, #9444, #39583 ) ) ;
#91753=ORIENTED_EDGE ( 'NONE', *, *, #75787, .T. ) ;
#91762=AXIS2_PLACEMENT_3D ( 'NONE', #94707, #94205, #71229 ) ;
#91765=( LENGTH_UNIT ( ) NAMED_UNIT ( * ) SI_UNIT ( .MILLI., .METRE. ) );
#91769=DIRECTION ( 'NONE',  ( 1.000000000000000000, 0.000000000000000000, 0.000000000000000000 ) ) ;
#91779=CARTESIAN_POINT ( 'NONE',  ( 17.75000000000000000, 73.00000000000001421, 6.500000000000000888 ) ) ;
#91780=ORIENTED_EDGE ( 'NONE', *, *, #21393, .F. ) ;
#91783=ORIENTED_EDGE ( 'NONE', *, *, #92151, .F. ) ;
#91787=PRESENTATION_STYLE_ASSIGNMENT (( #61278 ) ) ;
#91795=EDGE_LOOP ( 'NONE', ( #89367, #66591, #22181 ) ) ;
#91810=VECTOR ( 'NONE', #1486, 1000.000000000000000 ) ;
#91812=CARTESIAN_POINT ( 'NONE',  ( -8.900000000000002132, 75.76920769491746910, 3.000000000000000000 ) ) ;
#91815=PRESENTATION_STYLE_ASSIGNMENT (( #15827 ) ) ;
#91821=( NAMED_UNIT ( * ) PLANE_ANGLE_UNIT ( ) SI_UNIT ( $, .RADIAN. ) );
#91827=VERTEX_POINT ( 'NONE', #55501 ) ;
#91850=CARTESIAN_POINT ( 'NONE',  ( -4.000000000000000000, 10.00000000000000000, -2.750000000000000000 ) ) ;
#91857=EDGE_LOOP ( 'NONE', ( #59554, #21892, #17937, #76157 ) ) ;
#91892=ORIENTED_EDGE ( 'NONE', *, *, #87170, .F. ) ;
#91926=DIRECTION ( 'NONE',  ( -0.000000000000000000, 0.000000000000000000, 1.000000000000000000 ) ) ;
#91927=FACE_OUTER_BOUND ( 'NONE', #52743, .T. ) ;
#91944=CARTESIAN_POINT ( 'NONE',  ( 4.903136312256997087, -13.39483660680936339, -2.750000000000000000 ) ) ;
#91945=CARTESIAN_POINT ( 'NONE',  ( 6.033511671525834785, -36.04540650298945792, 2.500000000003218315 ) ) ;
#91949=DIRECTION ( 'NONE',  ( 0.000000000000000000, 0.000000000000000000, 1.000000000000000000 ) ) ;
#91961=EDGE_LOOP ( 'NONE', ( #31885, #77648 ) ) ;
#91970=DIRECTION ( 'NONE',  ( 0.9999509640662961329, 0.009903002720634834083, 0.000000000000000000 ) ) ;
#91979=ORIENTED_EDGE ( 'NONE', *, *, #87612, .T. ) ;
#91988=EDGE_CURVE ( 'NONE', #39787, #64978, #98457, .T. ) ;
#92012=CARTESIAN_POINT ( 'NONE',  ( -8.665245649997663335, 87.00799529562949886, -4.320095926139194020 ) ) ;
#92018=TOROIDAL_SURFACE ( 'NONE', #98469, 3.690000000000000391, 0.2500000000000000000 ) ;
#92019=PRESENTATION_STYLE_ASSIGNMENT (( #61510 ) ) ;
#92023=DIRECTION ( 'NONE',  ( -1.000000000000000000, 0.000000000000000000, -0.000000000000000000 ) ) ;
#92032=AXIS2_PLACEMENT_3D ( 'NONE', #76328, #53828, #1343 ) ;
#92036=VERTEX_POINT ( 'NONE', #14945 ) ;
#92042=VERTEX_POINT ( 'NONE', #451 ) ;
#92050=CARTESIAN_POINT ( 'NONE',  ( -8.000000000000000000, 1.019547802438458550, -3.750000000000000000 ) ) ;
#92071=PRESENTATION_STYLE_ASSIGNMENT (( #8090 ) ) ;
#92076=MECHANICAL_DESIGN_GEOMETRIC_PRESENTATION_REPRESENTATION('',(#95270),#64928);
#92087=CARTESIAN_POINT ( 'NONE',  ( -5.999999999999994671, 41.24999999999999289, -6.500000000000000888 ) ) ;
#92094=CARTESIAN_POINT ( 'NONE',  ( -6.319286839011487800, -45.42958518191715456, -2.500000000000000000 ) ) ;
#92096=FACE_OUTER_BOUND ( 'NONE', #79451, .T. ) ;
#92120=AXIS2_PLACEMENT_3D ( 'NONE', #48413, #77929, #33395 ) ;
#92123=( GEOMETRIC_REPRESENTATION_CONTEXT ( 3 ) GLOBAL_UNCERTAINTY_ASSIGNED_CONTEXT ( ( #63204 ) ) GLOBAL_UNIT_ASSIGNED_CONTEXT ( ( #38628, #68635, #15648 ) ) REPRESENTATION_CONTEXT ( 'NONE', 'WORKASPACE' ) );
#92132=CARTESIAN_POINT ( 'NONE',  ( -10.57481851845687260, -40.44832046089691602, 3.750000000000000000 ) ) ;
#92137=ADVANCED_FACE ( 'NONE', ( #67442 ), #90410, .T. ) ;
#92142=ORIENTED_EDGE ( 'NONE', *, *, #11850, .T. ) ;
#92151=EDGE_CURVE ( 'NONE', #35492, #18106, #65916, .T. ) ;
#92153=CARTESIAN_POINT ( 'NONE',  ( 17.75000000000000000, 84.07179676972448590, 3.750000000000000000 ) ) ;
#92156=AXIS2_PLACEMENT_3D ( 'NONE', #65276, #86825, #95297 ) ;
#92161=ORIENTED_EDGE ( 'NONE', *, *, #15724, .F. ) ;
#92175=( GEOMETRIC_REPRESENTATION_CONTEXT ( 3 ) GLOBAL_UNCERTAINTY_ASSIGNED_CONTEXT ( ( #20492 ) ) GLOBAL_UNIT_ASSIGNED_CONTEXT ( ( #9055, #41043, #64003 ) ) REPRESENTATION_CONTEXT ( 'NONE', 'WORKASPACE' ) );
#92176=CARTESIAN_POINT ( 'NONE',  ( -8.924603092375777535, 75.06466731010172566, -2.900000000000000799 ) ) ;
#92189=VECTOR ( 'NONE', #42476, 1000.000000000000000 ) ;
#92194=AXIS2_PLACEMENT_3D ( 'NONE', #46670, #1691, #54655 ) ;
#92195=AXIS2_PLACEMENT_3D ( 'NONE', #36038, #14544, #66541 ) ;
#92196=CARTESIAN_POINT ( 'NONE',  ( 4.471352795669433888, -3.620003340312029749, -2.749999999999999556 ) ) ;
#92204=CARTESIAN_POINT ( 'NONE',  ( 0.000000000000000000, -97.00000000000000000, 3.750000000000000000 ) ) ;
#92215=( BOUNDED_SURFACE ( )  B_SPLINE_SURFACE ( 3, 2, ( 
 ( #96957, #28429, #43912 ),
 ( #66923, #97444, #95957 ),
 ( #88935, #89916, #21430 ),
 ( #27439, #35433, #51927 ),
 ( #57933, #44414, #6416 ),
 ( #88442, #61874, #22922 ),
 ( #76398, #53391, #62361 ),
 ( #82914, #75404, #77367 ),
 ( #84405, #37925, #22426 ),
 ( #75903, #60402, #92379 ),
 ( #83900, #38904, #69889 ),
 ( #30889, #83410, #6922 ),
 ( #14931, #69391, #37431 ),
 ( #23905, #8395, #913 ),
 ( #90898, #39396, #45397 ),
 ( #14432, #76881, #44901 ),
 ( #92865, #45910, #1409 ),
 ( #67920, #53898, #98937 ) ),
 .UNSPECIFIED., .F., .F., .T. ) 
 B_SPLINE_SURFACE_WITH_KNOTS ( ( 4, 2, 2, 2, 2, 2, 2, 2, 4 ),
 ( 3, 3 ),
 ( 0.000000000000000000, 0.002783952809522130881, 0.005567905619044261761, 0.01113581123808852352, 0.02227162247617704705, 0.04454324495235409409, 0.06681486742853114114, 0.07795067866661967160, 0.08908648990470818818 ),
 ( 0.000000000000000000, 1.000000000000000000 ),
 .UNSPECIFIED. ) 
 GEOMETRIC_REPRESENTATION_ITEM ( )  RATIONAL_B_SPLINE_SURFACE ( (
 ( 1.000000000000000000, 0.7071067811865475727, 1.000000000000000000),
 ( 1.000000000000000000, 0.7071067811865475727, 1.000000000000000000),
 ( 1.000000000000000000, 0.7071067811865475727, 1.000000000000000000),
 ( 1.000000000000000000, 0.7071067811865475727, 1.000000000000000000),
 ( 1.000000000000000000, 0.7071067811865475727, 1.000000000000000000),
 ( 1.000000000000000000, 0.7071067811865475727, 1.000000000000000000),
 ( 1.000000000000000000, 0.7071067811865475727, 1.000000000000000000),
 ( 1.000000000000000000, 0.7071067811865475727, 1.000000000000000000),
 ( 1.000000000000000000, 0.7071067811865475727, 1.000000000000000000),
 ( 1.000000000000000000, 0.7071067811865475727, 1.000000000000000000),
 ( 1.000000000000000000, 0.7071067811865487940, 1.000000000000000000),
 ( 1.000000000000000000, 0.7071067811865487940, 1.000000000000000000),
 ( 1.000000000000000000, 0.7071067811865487940, 1.000000000000000000),
 ( 1.000000000000000000, 0.7071067811865487940, 1.000000000000000000),
 ( 1.000000000000000000, 0.7071067811865475727, 1.000000000000000000),
 ( 1.000000000000000000, 0.7071067811865475727, 1.000000000000000000),
 ( 1.000000000000000000, 0.7071067811865479058, 1.000000000000000000),
 ( 1.000000000000000000, 0.7071067811865479058, 1.000000000000000000) ) ) 
 REPRESENTATION_ITEM ( '' )  SURFACE ( )  );
#92223=DIRECTION ( 'NONE',  ( 0.000000000000000000, -0.000000000000000000, 1.000000000000000000 ) ) ;
#92224=AXIS2_PLACEMENT_3D ( 'NONE', #80367, #18886, #3887 ) ;
#92245=ORIENTED_EDGE ( 'NONE', *, *, #39998, .T. ) ;
#92246=ORIENTED_EDGE ( 'NONE', *, *, #70402, .F. ) ;
#92247=DIRECTION ( 'NONE',  ( 1.000000000000000000, 0.000000000000000000, 0.000000000000000000 ) ) ;
#92255=ADVANCED_FACE ( 'NONE', ( #28380 ), #5400, .T. ) ;
#92261=CIRCLE ( 'NONE', #71504, 0.2500000000000002220 ) ;
#92262=DIRECTION ( 'NONE',  ( 0.000000000000000000, 0.000000000000000000, 1.000000000000000000 ) ) ;
#92263=ORIENTED_EDGE ( 'NONE', *, *, #61633, .F. ) ;
#92264=CARTESIAN_POINT ( 'NONE',  ( -4.000000000000000000, 10.25000000000000000, 3.750000000000000000 ) ) ;
#92272=SURFACE_STYLE_FILL_AREA ( #69283 ) ;
#92280=FILL_AREA_STYLE_COLOUR ( '', #12520 ) ;
#92281=VERTEX_POINT ( 'NONE', #83353 ) ;
#92290=CYLINDRICAL_SURFACE ( 'NONE', #32402, 0.1000000000000001166 ) ;
#92291=( NAMED_UNIT ( * ) SI_UNIT ( $, .STERADIAN. ) SOLID_ANGLE_UNIT ( ) );
#92300=CARTESIAN_POINT ( 'NONE',  ( -4.261098214579363663, -13.83547760778420077, -2.749999999999999556 ) ) ;
#92303=DIRECTION ( 'NONE',  ( 0.000000000000000000, 0.000000000000000000, 1.000000000000000000 ) ) ;
#92310=CARTESIAN_POINT ( 'NONE',  ( 4.655929185074548116, -8.243906417136569686, -2.749999999999999556 ) ) ;
#92312=CARTESIAN_POINT ( 'NONE',  ( 6.579634127946655475, -87.99828267815715321, -3.750000000000000000 ) ) ;
#92316=AXIS2_PLACEMENT_3D ( 'NONE', #62154, #92660, #60687 ) ;
#92318=DIRECTION ( 'NONE',  ( -0.06975647374412512203, -0.9975640502598241977, 0.000000000000000000 ) ) ;
#92322=CARTESIAN_POINT ( 'NONE',  ( 18.00000000000000000, 77.62866902037677619, -4.012032253954680883 ) ) ;
#92324=EDGE_CURVE ( 'NONE', #65307, #80133, #66868, .T. ) ;
#92326=VECTOR ( 'NONE', #27293, 1000.000000000000000 ) ;
#92329=B_SPLINE_CURVE_WITH_KNOTS ( 'NONE', 3,
 ( #16931, #70426, #71885, #47409 ),
 .UNSPECIFIED., .F., .F.,
 ( 4, 4 ),
 ( 3.469446951953613804E-18, 0.0001414015891011769215 ),
 .UNSPECIFIED. ) ;
#92332=ORIENTED_EDGE ( 'NONE', *, *, #52334, .F. ) ;
#92344=CARTESIAN_POINT ( 'NONE',  ( -8.647966315259102643, -15.58183027063508952, -3.999999999999999112 ) ) ;
#92355=( NAMED_UNIT ( * ) SI_UNIT ( $, .STERADIAN. ) SOLID_ANGLE_UNIT ( ) );
#92365=EDGE_CURVE ( 'NONE', #70878, #94114, #35383, .T. ) ;
#92371=VERTEX_POINT ( 'NONE', #66364 ) ;
#92374=ORIENTED_EDGE ( 'NONE', *, *, #36578, .T. ) ;
#92377=VERTEX_POINT ( 'NONE', #28853 ) ;
#92379=CARTESIAN_POINT ( 'NONE',  ( 5.930070213854097716, -28.64748318935870941, 4.000000000000000000 ) ) ;
#92397=EDGE_CURVE ( 'NONE', #25626, #69208, #69071, .T. ) ;
#92398=AXIS2_PLACEMENT_3D ( 'NONE', #28063, #12574, #27075 ) ;
#92401=CARTESIAN_POINT ( 'NONE',  ( -8.024359497401761132, 75.03672218798435267, 2.900000000000000355 ) ) ;
#92415=DIRECTION ( 'NONE',  ( 1.000000000000000000, 0.000000000000000000, 0.000000000000000000 ) ) ;
#92417=CARTESIAN_POINT ( 'NONE',  ( 15.00000000000000000, 77.07179676972447169, -4.250000000000000000 ) ) ;
#92420=ORIENTED_EDGE ( 'NONE', *, *, #82772, .F. ) ;
#92430=DIRECTION ( 'NONE',  ( 0.000000000000000000, 0.000000000000000000, -1.000000000000000000 ) ) ;
#92432=CARTESIAN_POINT ( 'NONE',  ( 4.145754220390653444, -0.8370734722285972929, 2.500000000000000000 ) ) ;
#92436=CARTESIAN_POINT ( 'NONE',  ( 18.00000000000001776, 4.625929269271493211E-15, -6.250000000000000000 ) ) ;
#92438=EDGE_CURVE ( 'NONE', #93321, #61288, #64258, .T. ) ;
#92445=VERTEX_POINT ( 'NONE', #81376 ) ;
#92453=LINE ( 'NONE', #23979, #64542 ) ;
#92464=VECTOR ( 'NONE', #44050, 1000.000000000000000 ) ;
#92468=MECHANICAL_DESIGN_GEOMETRIC_PRESENTATION_REPRESENTATION('',(#31790),#6254);
#92469=ADVANCED_FACE ( 'NONE', ( #60348 ), #63643, .T. ) ;
#92484=DIRECTION ( 'NONE',  ( -1.000000000000000000, 0.000000000000000000, 0.000000000000000000 ) ) ;
#92491=( BOUNDED_SURFACE ( )  B_SPLINE_SURFACE ( 3, 2, ( 
 ( #83253, #14776, #38257 ),
 ( #45248, #75744, #53243 ),
 ( #767, #60250, #68264 ),
 ( #75251, #76729, #7266 ),
 ( #84256, #82252, #38746 ),
 ( #21778, #68749, #281 ),
 ( #89755, #37277, #44748 ),
 ( #15759, #90247, #37768 ),
 ( #6764, #59751, #91742 ),
 ( #46243, #98784, #52257 ),
 ( #76249, #21272, #30728 ),
 ( #22762, #30232, #29254 ),
 ( #51768, #13768, #44255 ),
 ( #61235, #60736, #14275 ),
 ( #91238, #67766, #83748 ),
 ( #15271, #45752, #22271 ),
 ( #98286, #23262, #53737 ),
 ( #74759, #6267, #36772 ),
 ( #67264, #97792, #29740 ),
 ( #90743, #55203, #39732 ),
 ( #69732, #16731, #25714 ),
 ( #2733, #78707, #70226 ),
 ( #24240, #41216, #85717 ),
 ( #3206, #17232, #54218 ),
 ( #9221, #18206, #10702 ),
 ( #31713, #47709, #56207 ) ),
 .UNSPECIFIED., .F., .F., .F. ) 
 B_SPLINE_SURFACE_WITH_KNOTS ( ( 4, 2, 2, 2, 2, 2, 2, 2, 2, 2, 2, 2, 4 ),
 ( 3, 3 ),
 ( 0.000000000000000000, 0.001549856543994699394, 0.003099713087989398787, 0.006199426175978797575, 0.01239885235195759515, 0.02479770470391519030, 0.03719655705587278371, 0.04959540940783038060, 0.07439311411174556743, 0.08679196646370315738, 0.09299139263968195235, 0.09609110572767134983, 0.09919081881566076120 ),
 ( 0.000000000000000000, 1.000000000000000000 ),
 .UNSPECIFIED. ) 
 GEOMETRIC_REPRESENTATION_ITEM ( )  RATIONAL_B_SPLINE_SURFACE ( (
 ( 1.000000000000000000, 0.7071067811865475727, 1.000000000000000000),
 ( 1.000000000000000000, 0.7071067811865475727, 1.000000000000000000),
 ( 1.000000000000000000, 0.7071067811865475727, 1.000000000000000000),
 ( 1.000000000000000000, 0.7071067811865475727, 1.000000000000000000),
 ( 1.000000000000000000, 0.7071067811865475727, 1.000000000000000000),
 ( 1.000000000000000000, 0.7071067811865475727, 1.000000000000000000),
 ( 1.000000000000000000, 0.7071067811865475727, 1.000000000000000000),
 ( 1.000000000000000000, 0.7071067811865475727, 1.000000000000000000),
 ( 1.000000000000000000, 0.7071067811865475727, 1.000000000000000000),
 ( 1.000000000000000000, 0.7071067811865475727, 1.000000000000000000),
 ( 1.000000000000000000, 0.7071067811865475727, 1.000000000000000000),
 ( 1.000000000000000000, 0.7071067811865475727, 1.000000000000000000),
 ( 1.000000000000000000, 0.7071067811865475727, 1.000000000000000000),
 ( 1.000000000000000000, 0.7071067811865475727, 1.000000000000000000),
 ( 1.000000000000000000, 0.7071067811865496822, 1.000000000000000000),
 ( 1.000000000000000000, 0.7071067811865496822, 1.000000000000000000),
 ( 1.000000000000000000, 0.7071067811865475727, 1.000000000000000000),
 ( 1.000000000000000000, 0.7071067811865475727, 1.000000000000000000),
 ( 1.000000000000000000, 0.7071067811865475727, 1.000000000000000000),
 ( 1.000000000000000000, 0.7071067811865475727, 1.000000000000000000),
 ( 1.000000000000000000, 0.7071067811865475727, 1.000000000000000000),
 ( 1.000000000000000000, 0.7071067811865475727, 1.000000000000000000),
 ( 1.000000000000000000, 0.7071067811865475727, 1.000000000000000000),
 ( 1.000000000000000000, 0.7071067811865475727, 1.000000000000000000),
 ( 1.000000000000000000, 0.7071067811865475727, 1.000000000000000000),
 ( 1.000000000000000000, 0.7071067811865475727, 1.000000000000000000) ) ) 
 REPRESENTATION_ITEM ( '' )  SURFACE ( )  );
#92492=ORIENTED_EDGE ( 'NONE', *, *, #2301, .F. ) ;
#92502=CARTESIAN_POINT ( 'NONE',  ( 4.219999999999999751, 10.25000000000000000, 3.750000000000000000 ) ) ;
#92517=EDGE_CURVE ( 'NONE', #29532, #75564, #24475, .T. ) ;
#92524=ORIENTED_EDGE ( 'NONE', *, *, #52183, .F. ) ;
#92534=ORIENTED_EDGE ( 'NONE', *, *, #44366, .F. ) ;
#92536=CARTESIAN_POINT ( 'NONE',  ( -10.98829462902744858, 46.98606209026556968, 3.000000000000000000 ) ) ;
#92537=CARTESIAN_POINT ( 'NONE',  ( -16.94999999999999574, 99.99999999999998579, 7.750000000000000000 ) ) ;
#92550=VECTOR ( 'NONE', #98832, 1000.000000000000114 ) ;
#92560=EDGE_CURVE ( 'NONE', #15746, #63180, #89904, .T. ) ;
#92570=SURFACE_STYLE_USAGE ( .BOTH. , #94541 ) ;
#92580=CARTESIAN_POINT ( 'NONE',  ( -11.64999999999999680, 98.49999999999998579, 8.000000000000000000 ) ) ;
#92586=AXIS2_PLACEMENT_3D ( 'NONE', #47053, #46567, #31066 ) ;
#92593=ORIENTED_EDGE ( 'NONE', *, *, #26758, .F. ) ;
#92595=EDGE_CURVE ( 'NONE', #44503, #33481, #62773, .T. ) ;
#92603=FILL_AREA_STYLE_COLOUR ( '', #90547 ) ;
#92605=SURFACE_STYLE_USAGE ( .BOTH. , #62097 ) ;
#92614=CARTESIAN_POINT ( 'NONE',  ( -8.107943641493370990, -3.126452786875834722, 4.000000000000000000 ) ) ;
#92620=FACE_OUTER_BOUND ( 'NONE', #33970, .T. ) ;
#92645=DIRECTION ( 'NONE',  ( 0.000000000000000000, -1.000000000000000000, -1.734723475976805517E-15 ) ) ;
#92650=DIRECTION ( 'NONE',  ( 1.000000000000000000, 2.641710877122040890E-15, 0.000000000000000000 ) ) ;
#92652=DIRECTION ( 'NONE',  ( -0.6038238647437471629, 0.7971177707001175783, 1.387778780781426270E-14 ) ) ;
#92654=CARTESIAN_POINT ( 'NONE',  ( 8.991948000262459217, -4.139826107007521294, 3.750000000000000000 ) ) ;
#92657=PRESENTATION_STYLE_ASSIGNMENT (( #9665 ) ) ;
#92660=DIRECTION ( 'NONE',  ( 0.9975640502598243087, -0.06975647374412544122, -0.000000000000000000 ) ) ;
#92666=FILL_AREA_STYLE_COLOUR ( '', #68765 ) ;
#92675=EDGE_CURVE ( 'NONE', #63379, #61498, #96349, .T. ) ;
#92702=ORIENTED_EDGE ( 'NONE', *, *, #16628, .F. ) ;
#92714=EDGE_CURVE ( 'NONE', #67453, #11101, #45103, .T. ) ;
#92719=VECTOR ( 'NONE', #24600, 1000.000000000000000 ) ;
#92727=CARTESIAN_POINT ( 'NONE',  ( 3.969999999999999751, 37.00000000000000000, 3.750000000000000000 ) ) ;
#92732=CARTESIAN_POINT ( 'NONE',  ( -7.750000000000000000, 41.24999999999999289, -6.250000000000000000 ) ) ;
#92733=CARTESIAN_POINT ( 'NONE',  ( -8.000000000000001776, -7.313785530895824394, -3.750000000000000000 ) ) ;
#92742=DIRECTION ( 'NONE',  ( 0.000000000000000000, 1.000000000000000000, -0.000000000000000000 ) ) ;
#92743=DIRECTION ( 'NONE',  ( 0.8073289077885722476, -0.5901017155109032908, 5.601969636702199977E-15 ) ) ;
#92746=CARTESIAN_POINT ( 'NONE',  ( -7.330124059958221139, -69.53998168068582686, 4.000000000000000888 ) ) ;
#92747=ORIENTED_EDGE ( 'NONE', *, *, #17431, .F. ) ;
#92759=MECHANICAL_DESIGN_GEOMETRIC_PRESENTATION_REPRESENTATION('',(#59201),#22557);
#92761=AXIS2_PLACEMENT_3D ( 'NONE', #31389, #40400, #54880 ) ;
#92784=CARTESIAN_POINT ( 'NONE',  ( -6.607088223530021232, -50.94269062318750940, -2.749999999999999556 ) ) ;
#92786=EDGE_CURVE ( 'NONE', #98319, #24768, #37625, .T. ) ;
#92799=ADVANCED_FACE ( 'NONE', ( #67629 ), #15623, .F. ) ;
#92800=ORIENTED_EDGE ( 'NONE', *, *, #5766, .F. ) ;
#92801=FILL_AREA_STYLE_COLOUR ( '', #12153 ) ;
#92804=SURFACE_STYLE_USAGE ( .BOTH. , #79281 ) ;
#92809=MECHANICAL_DESIGN_GEOMETRIC_PRESENTATION_REPRESENTATION('',(#76821),#36944);
#92810=CARTESIAN_POINT ( 'NONE',  ( 18.00000000000000355, 78.50171742896758076, -3.769096794058098165 ) ) ;
#92811=DIRECTION ( 'NONE',  ( 0.000000000000000000, -1.000000000000000000, 0.000000000000000000 ) ) ;
#92813=CARTESIAN_POINT ( 'NONE',  ( -8.028888469223478097, -1.053269085630145208, -3.750000000000000000 ) ) ;
#92816=DIRECTION ( 'NONE',  ( -0.000000000000000000, 0.000000000000000000, 1.000000000000000000 ) ) ;
#92820=CARTESIAN_POINT ( 'NONE',  ( 0.000000000000000000, 10.25000000000000000, -2.500000000000000000 ) ) ;
#92830=CARTESIAN_POINT ( 'NONE',  ( 18.00000000000001776, 4.625929269271493211E-15, -8.000000000000000000 ) ) ;
#92831=EDGE_CURVE ( 'NONE', #9027, #74685, #51582, .T. ) ;
#92843=SURFACE_STYLE_USAGE ( .BOTH. , #62835 ) ;
#92858=B_SPLINE_CURVE_WITH_KNOTS ( 'NONE', 3,
 ( #94196, #87676, #27170, #57672, #88167, #56696, #14161, #98673, #6159, #66661, #6647, #51666, #73653, #81165, #89160, #51165, #43656, #96685 ),
 .UNSPECIFIED., .F., .F.,
 ( 4, 2, 2, 2, 2, 2, 2, 2, 4 ),
 ( 6.938893903907227145E-17, 0.01113440817397474449, 0.02226881634794941958, 0.04453763269589879059, 0.06680644904384815119, 0.07794085721782283149, 0.08350806130481017164, 0.08629166334830384866, 0.08907526539179752567 ),
 .UNSPECIFIED. ) ;
#92865=CARTESIAN_POINT ( 'NONE',  ( 6.910361961633475936, -84.29457034760254430, 3.750000000000000000 ) ) ;
#92874=ORIENTED_EDGE ( 'NONE', *, *, #21641, .F. ) ;
#92888=ORIENTED_EDGE ( 'NONE', *, *, #29040, .T. ) ;
#92899=CARTESIAN_POINT ( 'NONE',  ( -11.62814530702576477, -77.87069291667818050, 3.750000000000000888 ) ) ;
#92903=DIRECTION ( 'NONE',  ( 0.08715574274765151841, 0.9961946980917462113, 0.000000000000000000 ) ) ;
#92914=ADVANCED_FACE ( 'NONE', ( #62563 ), #70087, .F. ) ;
#92920=LINE ( 'NONE', #54917, #96264 ) ;
#92921=CARTESIAN_POINT ( 'NONE',  ( 4.380000001225145212, 0.09385850578814242118, 2.500000000000000000 ) ) ;
#92923=EDGE_LOOP ( 'NONE', ( #84767, #25516, #2563, #75579, #11821, #49819, #54235, #49215, #66598, #13409, #8258, #2457, #13861, #7199, #31474, #80320, #64822, #24296, #21489, #81094, #82298, #88932, #74087, #54656, #61391, #41534, #76288, #39066, #27245, #53270 ) ) ;
#92935=DIRECTION ( 'NONE',  ( 0.000000000000000000, 0.000000000000000000, 1.000000000000000000 ) ) ;
#92939=CARTESIAN_POINT ( 'NONE',  ( 17.88942758462985338, 78.22945624030553802, 4.041088224284109742 ) ) ;
#92941=FILL_AREA_STYLE ('',( #47448 ) ) ;
#92963=DIRECTION ( 'NONE',  ( 0.000000000000000000, 0.000000000000000000, 1.000000000000000000 ) ) ;
#92968=CARTESIAN_POINT ( 'NONE',  ( 5.129999999999991900, 76.07179676972444327, -6.250000000000000000 ) ) ;
#92969=DIRECTION ( 'NONE',  ( 0.06975647374412544122, 0.9975640502598243087, -0.000000000000000000 ) ) ;
#92977=CARTESIAN_POINT ( 'NONE',  ( 0.000000000000000000, 0.000000000000000000, 3.000000000000000000 ) ) ;
#92980=AXIS2_PLACEMENT_3D ( 'NONE', #13884, #74867, #29851 ) ;
#92984=ORIENTED_EDGE ( 'NONE', *, *, #80540, .T. ) ;
#92996=CARTESIAN_POINT ( 'NONE',  ( -6.000000000000014211, 80.32179676972448590, -4.000000000000000000 ) ) ;
#93027=EDGE_CURVE ( 'NONE', #92445, #85917, #31576, .T. ) ;
#93029=EDGE_LOOP ( 'NONE', ( #75854, #43375, #86019, #32596 ) ) ;
#93030=EDGE_LOOP ( 'NONE', ( #98317, #22023, #35016, #59691 ) ) ;
#93031=DIRECTION ( 'NONE',  ( 0.000000000000000000, 1.000000000000000000, 0.000000000000000000 ) ) ;
#93034=CIRCLE ( 'NONE', #13236, 0.2500000000000002220 ) ;
#93042=CARTESIAN_POINT ( 'NONE',  ( 15.00000000000000178, 73.00000000000000000, -6.250000000000000000 ) ) ;
#93044=COLOUR_RGB ( '', 0.40784314, 0.44705882, 0.49803922) ;
#93049=DIRECTION ( 'NONE',  ( 0.000000000000000000, 0.000000000000000000, -1.000000000000000000 ) ) ;
#93053=ORIENTED_EDGE ( 'NONE', *, *, #62783, .F. ) ;
#93059=CARTESIAN_POINT ( 'NONE',  ( 14.99999999999997868, 80.07179676972448590, -6.500000000000000888 ) ) ;
#93067=CARTESIAN_POINT ( 'NONE',  ( 12.30000000000000249, 99.99999999999998579, -8.525133428036873795 ) ) ;
#93070=ADVANCED_FACE ( 'NONE', ( #79050 ), #56372, .T. ) ;
#93094=FILL_AREA_STYLE_COLOUR ( '', #22626 ) ;
#93095=DIRECTION ( 'NONE',  ( 0.6246950475544238435, 0.7808688094430307203, 0.000000000000000000 ) ) ;
#93096=ORIENTED_EDGE ( 'NONE', *, *, #80127, .T. ) ;
#93102=LINE ( 'NONE', #70618, #43436 ) ;
#93108=COLOUR_RGB ( '', 0.31764706, 0.68627451, 0.89019608) ;
#93111=AXIS2_PLACEMENT_3D ( 'NONE', #98647, #44618, #75610 ) ;
#93116=( NAMED_UNIT ( * ) PLANE_ANGLE_UNIT ( ) SI_UNIT ( $, .RADIAN. ) );
#93123=CARTESIAN_POINT ( 'NONE',  ( 6.880000000000011440, 40.74999999999999289, -4.250000000000000000 ) ) ;
#93145=DIRECTION ( 'NONE',  ( -0.7971177707001109169, -0.6038238647437560447, -1.358445972092650111E-13 ) ) ;
#93147=DIRECTION ( 'NONE',  ( -1.000000000000000000, 0.000000000000000000, 0.000000000000000000 ) ) ;
#93149=DIRECTION ( 'NONE',  ( 0.000000000000000000, 0.000000000000000000, 1.000000000000000000 ) ) ;
#93150=EDGE_CURVE ( 'NONE', #82102, #96688, #539, .T. ) ;
#93151=CARTESIAN_POINT ( 'NONE',  ( -51.18902439024388684, 40.95121951219505974, -8.000000000000000000 ) ) ;
#93153=ORIENTED_EDGE ( 'NONE', *, *, #2661, .T. ) ;
#93154=DIRECTION ( 'NONE',  ( 0.000000000000000000, 0.000000000000000000, 1.000000000000000000 ) ) ;
#93155=CARTESIAN_POINT ( 'NONE',  ( 9.879999999999990123, 20.99999999999999645, 1.249999999999987121 ) ) ;
#93165=STYLED_ITEM ( 'NONE', ( #70841 ), #96833 ) ;
#93173=CARTESIAN_POINT ( 'NONE',  ( 3.969999999999999751, 10.25000000000000000, -2.750000000000000000 ) ) ;
#93184=ADVANCED_FACE ( 'NONE', ( #58147 ), #69009, .T. ) ;
#93189=ORIENTED_EDGE ( 'NONE', *, *, #73026, .T. ) ;
#93202=DIRECTION ( 'NONE',  ( 1.000000000000000000, 1.257402221000611116E-16, -0.000000000000000000 ) ) ;
#93212=UNCERTAINTY_MEASURE_WITH_UNIT (LENGTH_MEASURE( 1.000000000000000082E-05 ), #69301, 'distance_accuracy_value', 'NONE');
#93215=CARTESIAN_POINT ( 'NONE',  ( -3.949999999999997069, 99.99999999999998579, -8.000000000000000000 ) ) ;
#93217=CARTESIAN_POINT ( 'NONE',  ( -11.81797300553251162, -43.76346696326814367, -3.750000000000000000 ) ) ;
#93232=CARTESIAN_POINT ( 'NONE',  ( -6.857667818328269327, -50.95147662124757915, 3.999999999999999112 ) ) ;
#93235=ORIENTED_EDGE ( 'NONE', *, *, #70253, .T. ) ;
#93247=EDGE_CURVE ( 'NONE', #9027, #16419, #55973, .T. ) ;
#93253=MECHANICAL_DESIGN_GEOMETRIC_PRESENTATION_REPRESENTATION('',(#32584),#54912);
#93254=ORIENTED_EDGE ( 'NONE', *, *, #93150, .T. ) ;
#93275=CARTESIAN_POINT ( 'NONE',  ( 6.879999999999995453, 43.00000000000000000, 4.000000000000000000 ) ) ;
#93289=CARTESIAN_POINT ( 'NONE',  ( -8.048010592883702685, 84.92462609336300261, 4.034077756265262771 ) ) ;
#93296=DIRECTION ( 'NONE',  ( -1.000000000000000000, 0.000000000000000000, 0.000000000000000000 ) ) ;
#93299=FACE_OUTER_BOUND ( 'NONE', #22313, .T. ) ;
#93302=CARTESIAN_POINT ( 'NONE',  ( -16.80847703285585482, 99.89644660940670917, -8.000000000000001776 ) ) ;
#93309=AXIS2_PLACEMENT_3D ( 'NONE', #65852, #28355, #35359 ) ;
#93313=CARTESIAN_POINT ( 'NONE',  ( -10.00219152607946604, 88.91691738930978772, -5.623636179944087488 ) ) ;
#93319=CARTESIAN_POINT ( 'NONE',  ( 9.879999999999990123, 20.99999999999999645, 2.900000000000000355 ) ) ;
#93321=VERTEX_POINT ( 'NONE', #47472 ) ;
#93324=CARTESIAN_POINT ( 'NONE',  ( -8.024359497401761132, 75.03672218798435267, -2.900000000000000799 ) ) ;
#93330=CARTESIAN_POINT ( 'NONE',  ( 6.284583270191197002, -88.40194713205143273, 4.000000000000000000 ) ) ;
#93339=UNCERTAINTY_MEASURE_WITH_UNIT (LENGTH_MEASURE( 1.000000000000000082E-05 ), #54088, 'distance_accuracy_value', 'NONE');
#93356=ORIENTED_EDGE ( 'NONE', *, *, #90871, .F. ) ;
#93358=DIRECTION ( 'NONE',  ( -0.000000000000000000, -1.000000000000000000, -0.000000000000000000 ) ) ;
#93373=DIRECTION ( 'NONE',  ( 0.000000000000000000, 0.000000000000000000, 1.000000000000000000 ) ) ;
#93386=( GEOMETRIC_REPRESENTATION_CONTEXT ( 3 ) GLOBAL_UNCERTAINTY_ASSIGNED_CONTEXT ( ( #22470 ) ) GLOBAL_UNIT_ASSIGNED_CONTEXT ( ( #95002, #87994, #79523 ) ) REPRESENTATION_CONTEXT ( 'NONE', 'WORKASPACE' ) );
#93399=FACE_OUTER_BOUND ( 'NONE', #85240, .T. ) ;
#93402=SURFACE_STYLE_FILL_AREA ( #48392 ) ;
#93405=EDGE_CURVE ( 'NONE', #2183, #7152, #89965, .T. ) ;
#93422=CARTESIAN_POINT ( 'NONE',  ( 5.113979357148443761, -17.50950876261946121, 2.500000000000000000 ) ) ;
#93424=ORIENTED_EDGE ( 'NONE', *, *, #41137, .F. ) ;
#93441=CARTESIAN_POINT ( 'NONE',  ( 17.97673312326547901, 77.65179697821409377, 4.136170292160840312 ) ) ;
#93444=EDGE_CURVE ( 'NONE', #24768, #11943, #94936, .T. ) ;
#93447=CIRCLE ( 'NONE', #7238, 11.15000000000026326 ) ;
#93468=VERTEX_POINT ( 'NONE', #50420 ) ;
#93469=SURFACE_STYLE_FILL_AREA ( #53992 ) ;
#93481=CARTESIAN_POINT ( 'NONE',  ( -6.319286839011487800, -45.42958518191715456, 2.500000000000000000 ) ) ;
#93482=ORIENTED_EDGE ( 'NONE', *, *, #28919, .T. ) ;
#93500=VERTEX_POINT ( 'NONE', #81411 ) ;
#93514=EDGE_CURVE ( 'NONE', #49695, #69049, #95440, .T. ) ;
#93521=CARTESIAN_POINT ( 'NONE',  ( 4.130000000000002558, 1.019547802438462547, 2.500000000000000000 ) ) ;
#93526=ORIENTED_EDGE ( 'NONE', *, *, #95242, .T. ) ;
#93536=VERTEX_POINT ( 'NONE', #12421 ) ;
#93548=VERTEX_POINT ( 'NONE', #79935 ) ;
#93554=CARTESIAN_POINT ( 'NONE',  ( -7.984789763142470242, 85.83064272735667544, 4.183481735294424020 ) ) ;
#93563=PLANE ( 'NONE',  #67170 ) ;
#93565=CARTESIAN_POINT ( 'NONE',  ( -8.957287532561966970, -19.72663685366165254, 4.000000000000000000 ) ) ;
#93569=DIRECTION ( 'NONE',  ( -1.000000000000000000, -1.257402221000611116E-16, 0.000000000000000000 ) ) ;
#93570=PRESENTATION_STYLE_ASSIGNMENT (( #62572 ) ) ;
#93576=DIRECTION ( 'NONE',  ( 0.8070303256584298035, -0.5905099943842175847, 0.000000000000000000 ) ) ;
#93589=CARTESIAN_POINT ( 'NONE',  ( 7.079515573063599021, -88.00917032380691296, 3.750000000000000000 ) ) ;
#93597=EDGE_CURVE ( 'NONE', #55430, #64082, #11442, .T. ) ;
#93607=EDGE_CURVE ( 'NONE', #86221, #95526, #73408, .T. ) ;
#93614=VERTEX_POINT ( 'NONE', #58403 ) ;
#93640=CARTESIAN_POINT ( 'NONE',  ( -3.887834249507322593, -8.254296980867463773, 2.500000000000001776 ) ) ;
#93652=ORIENTED_EDGE ( 'NONE', *, *, #70253, .F. ) ;
#93658=AXIS2_PLACEMENT_3D ( 'NONE', #3300, #95272, #81733 ) ;
#93662=( GEOMETRIC_REPRESENTATION_CONTEXT ( 3 ) GLOBAL_UNCERTAINTY_ASSIGNED_CONTEXT ( ( #11176 ) ) GLOBAL_UNIT_ASSIGNED_CONTEXT ( ( #16772, #46281, #30765 ) ) REPRESENTATION_CONTEXT ( 'NONE', 'WORKASPACE' ) );
#93663=CIRCLE ( 'NONE', #1054, 3.940000000000000835 ) ;
#93673=CARTESIAN_POINT ( 'NONE',  ( 0.4400000000000020006, 1.019547802438468986, -2.750000000000000000 ) ) ;
#93679=DIRECTION ( 'NONE',  ( 0.000000000000000000, 0.000000000000000000, 1.000000000000000000 ) ) ;
#93687=EDGE_LOOP ( 'NONE', ( #55026, #556, #22453, #74578 ) ) ;
#93717=( NAMED_UNIT ( * ) PLANE_ANGLE_UNIT ( ) SI_UNIT ( $, .RADIAN. ) );
#93725=LINE ( 'NONE', #55231, #68364 ) ;
#93729=CARTESIAN_POINT ( 'NONE',  ( -7.287642027973244119, -86.26866148728002770, 4.000000000000000000 ) ) ;
#93744=ORIENTED_EDGE ( 'NONE', *, *, #43586, .T. ) ;
#93754=VECTOR ( 'NONE', #64953, 1000.000000000000000 ) ;
#93756=CIRCLE ( 'NONE', #28310, 0.2500000000000002220 ) ;
#93757=MECHANICAL_DESIGN_GEOMETRIC_PRESENTATION_REPRESENTATION('',(#72981),#42657);
#93762=SURFACE_SIDE_STYLE ('',( #77770 ) ) ;
#93781=CARTESIAN_POINT ( 'NONE',  ( -8.114998381645635916, 86.24535146302233102, 4.289708087854926077 ) ) ;
#93786=CARTESIAN_POINT ( 'NONE',  ( 4.395797040798986366, -0.8371465525320274104, 2.750000000000000444 ) ) ;
#93795=CARTESIAN_POINT ( 'NONE',  ( -16.94999999999999574, 99.99999999999998579, -7.750000000000000000 ) ) ;
#93807=CARTESIAN_POINT ( 'NONE',  ( -7.803778109523453743, 84.96281847254653030, -4.037836297607493741 ) ) ;
#93823=CARTESIAN_POINT ( 'NONE',  ( 11.15633344610952804, -69.21805206901655083, -4.000000000000000000 ) ) ;
#93826=( NAMED_UNIT ( * ) SI_UNIT ( $, .STERADIAN. ) SOLID_ANGLE_UNIT ( ) );
#93829=AXIS2_PLACEMENT_3D ( 'NONE', #8339, #15370, #16827 ) ;
#93838=LINE ( 'NONE', #32831, #79150 ) ;
#93849=ORIENTED_EDGE ( 'NONE', *, *, #12536, .T. ) ;
#93854=VERTEX_POINT ( 'NONE', #45965 ) ;
#93855=CARTESIAN_POINT ( 'NONE',  ( -7.750000000000000000, 43.00000000000000000, -6.500000000000000888 ) ) ;
#93857=CARTESIAN_POINT ( 'NONE',  ( -5.149999999999996803, 98.49999999999998579, 8.000000000000000000 ) ) ;
#93865=ORIENTED_EDGE ( 'NONE', *, *, #46328, .F. ) ;
#93867=ORIENTED_EDGE ( 'NONE', *, *, #30963, .T. ) ;
#93868=FACE_OUTER_BOUND ( 'NONE', #25762, .T. ) ;
#93876=EDGE_CURVE ( 'NONE', #69049, #55236, #8448, .T. ) ;
#93889=CARTESIAN_POINT ( 'NONE',  ( -11.62550287597698784, -75.79306049738043782, 3.750000000000000444 ) ) ;
#93892=DIRECTION ( 'NONE',  ( 0.9942165912674658657, -0.1073935270325955399, 0.000000000000000000 ) ) ;
#93897=DIRECTION ( 'NONE',  ( -0.000000000000000000, -0.000000000000000000, -1.000000000000000000 ) ) ;
#93901=SURFACE_STYLE_USAGE ( .BOTH. , #10899 ) ;
#93916=CARTESIAN_POINT ( 'NONE',  ( 4.191189844333585768, -2.692444605319266326, 2.500000000000000000 ) ) ;
#93919=ORIENTED_EDGE ( 'NONE', *, *, #46382, .F. ) ;
#93927=CARTESIAN_POINT ( 'NONE',  ( 6.880000000000009663, 40.99999999999999289, 4.250000000000000000 ) ) ;
#93928=ADVANCED_FACE ( 'NONE', ( #2455 ), #26568, .F. ) ;
#93934=CARTESIAN_POINT ( 'NONE',  ( -3.521809513897767641, -0.8352226969158469405, -2.749999999999595879 ) ) ;
#93937=CARTESIAN_POINT ( 'NONE',  ( -19.64999999999999858, 98.99999999999998579, -8.000000000000000000 ) ) ;
#93940=CARTESIAN_POINT ( 'NONE',  ( -15.00000000000000000, 83.99999999999998579, 3.750000000000000000 ) ) ;
#93950=ORIENTED_EDGE ( 'NONE', *, *, #16980, .F. ) ;
#93951=ADVANCED_FACE ( 'NONE', ( #88383, #36746 ), #48899, .F. ) ;
#93955=AXIS2_PLACEMENT_3D ( 'NONE', #31494, #46996, #17012 ) ;
#93971=ORIENTED_EDGE ( 'NONE', *, *, #28646, .T. ) ;
#93973=MECHANICAL_DESIGN_GEOMETRIC_PRESENTATION_REPRESENTATION('',(#66781),#79557);
#93979=ORIENTED_EDGE ( 'NONE', *, *, #52861, .T. ) ;
#93989=CARTESIAN_POINT ( 'NONE',  ( -11.16114668437453084, -52.93485207676555149, -3.749999999999999556 ) ) ;
#93993=ORIENTED_EDGE ( 'NONE', *, *, #18074, .F. ) ;
#94012=DIRECTION ( 'NONE',  ( 0.000000000000000000, 0.000000000000000000, -1.000000000000000000 ) ) ;
#94023=B_SPLINE_CURVE_WITH_KNOTS ( 'NONE', 3,
 ( #98568, #37052, #61017, #91017, #21560, #7048, #52532, #83040, #90523, #31495, #37552, #69519, #15548, #67551, #92012, #60527, #54014, #68537, #22058, #38532 ),
 .UNSPECIFIED., .F., .F.,
 ( 4, 2, 2, 2, 2, 2, 2, 2, 2, 4 ),
 ( 0.001219073179698296813, 0.001886422127363689919, 0.002553771075029083026, 0.003888468970359869239, 0.005223166865690655886, 0.006557864761021442099, 0.007892562656352228312, 0.009227260551683014525, 0.01056195844701380074, 0.01189665634234458695 ),
 .UNSPECIFIED. ) ;
#94029=STYLED_ITEM ( 'NONE', ( #6793 ), #14479 ) ;
#94033=CARTESIAN_POINT ( 'NONE',  ( 3.969999999999999751, 9.750000000000000000, 3.750000000000000000 ) ) ;
#94034=ORIENTED_EDGE ( 'NONE', *, *, #14952, .F. ) ;
#94041=CARTESIAN_POINT ( 'NONE',  ( -3.750000000000000000, 10.00000000000000000, 4.000000000000000000 ) ) ;
#94045=ORIENTED_EDGE ( 'NONE', *, *, #32680, .F. ) ;
#94052=CARTESIAN_POINT ( 'NONE',  ( -9.098828036256710661, 88.10682954397124433, 5.081100641017341601 ) ) ;
#94058=DIRECTION ( 'NONE',  ( 0.000000000000000000, -1.000000000000000000, 0.000000000000000000 ) ) ;
#94060=CARTESIAN_POINT ( 'NONE',  ( 0.000000000000000000, 69.99999999999998579, -6.250000000000000000 ) ) ;
#94061=MECHANICAL_DESIGN_GEOMETRIC_PRESENTATION_REPRESENTATION('',(#38198),#4645);
#94062=CARTESIAN_POINT ( 'NONE',  ( 18.00000000000000000, 84.07179676972448590, 12.00000000000000000 ) ) ;
#94072=CARTESIAN_POINT ( 'NONE',  ( -5.069238243371155583, -24.95996232635749834, -3.750000000000000888 ) ) ;
#94073=FACE_OUTER_BOUND ( 'NONE', #11719, .T. ) ;
#94090=EDGE_LOOP ( 'NONE', ( #34990, #37307, #66043 ) ) ;
#94102=EDGE_LOOP ( 'NONE', ( #15001, #57606, #57695, #61178 ) ) ;
#94110=FILL_AREA_STYLE ('',( #78627 ) ) ;
#94112=B_SPLINE_CURVE_WITH_KNOTS ( 'NONE', 3,
 ( #94822, #27303, #88310, #81782, #18839, #45779, #14804, #89783, #74786, #6295, #82279, #98811, #75279, #36296, #30260, #60274, #43783, #66793 ),
 .UNSPECIFIED., .F., .F.,
 ( 4, 2, 2, 2, 2, 2, 2, 2, 4 ),
 ( 0.000000000000000000, 0.002783400404998704388, 0.005566800809997408776, 0.01113360161999481755, 0.02226720323998963511, 0.04453440647997927021, 0.06680160971996890185, 0.07793521133996370032, 0.08906881295995849879 ),
 .UNSPECIFIED. ) ;
#94114=VERTEX_POINT ( 'NONE', #74730 ) ;
#94118=VERTEX_POINT ( 'NONE', #67237 ) ;
#94130=CARTESIAN_POINT ( 'NONE',  ( 10.72176212051081734, -40.27637155869391705, 4.000000000000000888 ) ) ;
#94135=VECTOR ( 'NONE', #68354, 1000.000000000000000 ) ;
#94144=SURFACE_STYLE_USAGE ( .BOTH. , #63637 ) ;
#94173=EDGE_LOOP ( 'NONE', ( #76259, #39063, #80983, #25313 ) ) ;
#94179=DIRECTION ( 'NONE',  ( -1.257402221000611116E-16, 1.000000000000000000, -0.000000000000000000 ) ) ;
#94185=CARTESIAN_POINT ( 'NONE',  ( 6.004190426492125532, -34.81345361117713111, 3.750000000000001776 ) ) ;
#94194=ADVANCED_FACE ( 'NONE', ( #60223 ), #2287, .T. ) ;
#94195=UNCERTAINTY_MEASURE_WITH_UNIT (LENGTH_MEASURE( 1.000000000000000082E-05 ), #43632, 'distance_accuracy_value', 'NONE');
#94196=CARTESIAN_POINT ( 'NONE',  ( 6.579634127946608402, -87.99828267815712479, 2.500000000000000000 ) ) ;
#94199=DIRECTION ( 'NONE',  ( -0.000000000000000000, -0.000000000000000000, 1.000000000000000000 ) ) ;
#94205=DIRECTION ( 'NONE',  ( -0.000000000000000000, 0.000000000000000000, 1.000000000000000000 ) ) ;
#94211=DIRECTION ( 'NONE',  ( -1.000000000000000000, 0.000000000000000000, 0.000000000000000000 ) ) ;
#94212=CARTESIAN_POINT ( 'NONE',  ( 17.97400638239465565, 77.67876782659364210, 4.131022355321460893 ) ) ;
#94215=VECTOR ( 'NONE', #84227, 1000.000000000000000 ) ;
#94216=CARTESIAN_POINT ( 'NONE',  ( -7.116171662378945051, -80.69120418497870162, 3.749999999999193534 ) ) ;
#94221=EDGE_LOOP ( 'NONE', ( #82585, #90564, #42007, #97317 ) ) ;
#94228=EDGE_LOOP ( 'NONE', ( #60648, #82250, #22561, #86626 ) ) ;
#94237=LINE ( 'NONE', #25768, #87837 ) ;
#94239=EDGE_CURVE ( 'NONE', #96487, #79084, #83720, .T. ) ;
#94242=( LENGTH_UNIT ( ) NAMED_UNIT ( * ) SI_UNIT ( .MILLI., .METRE. ) );
#94244=DIRECTION ( 'NONE',  ( -1.000000000000000000, 0.000000000000000000, -0.000000000000000000 ) ) ;
#94245=FILL_AREA_STYLE ('',( #32758 ) ) ;
#94250=CIRCLE ( 'NONE', #54281, 10.90000000000026326 ) ;
#94259=AXIS2_PLACEMENT_3D ( 'NONE', #26243, #64708, #94738 ) ;
#94287=AXIS2_PLACEMENT_3D ( 'NONE', #88603, #4145, #49138 ) ;
#94299=EDGE_LOOP ( 'NONE', ( #71411, #93189, #37734, #67253 ) ) ;
#94307=CARTESIAN_POINT ( 'NONE',  ( 8.650319761586390044, -1.048872767157960961, -3.999999999999999112 ) ) ;
#94316=UNCERTAINTY_MEASURE_WITH_UNIT (LENGTH_MEASURE( 1.000000000000000082E-05 ), #69164, 'distance_accuracy_value', 'NONE');
#94317=( BOUNDED_SURFACE ( )  B_SPLINE_SURFACE ( 3, 2, ( 
 ( #97197, #19692, #73170 ),
 ( #65672, #44655, #50179 ),
 ( #14171, #58669, #96696 ),
 ( #13169, #36674, #96193 ),
 ( #58163, #82155, #51176 ),
 ( #50685, #81177, #36172 ),
 ( #66672, #59157, #21174 ),
 ( #13667, #44151, #74659 ),
 ( #61130, #30131, #91640 ),
 ( #46142, #68162, #69141 ),
 ( #68645, #669, #38159 ),
 ( #60637, #31119, #175 ),
 ( #14675, #84632, #23158 ),
 ( #15659, #6660, #8147 ),
 ( #53140, #61614, #16134 ),
 ( #76628, #38640, #54119 ),
 ( #91138, #29635, #83649 ),
 ( #22664, #77118, #54605 ),
 ( #15164, #45141, #92132 ),
 ( #75647, #23657, #46620 ),
 ( #30623, #85121, #31613 ),
 ( #53633, #8630, #39139 ),
 ( #45645, #7668, #76142 ),
 ( #1153, #7159, #90640 ),
 ( #67669, #37176, #84153 ),
 ( #69629, #62104, #37662 ),
 ( #16632, #92614, #75150 ),
 ( #98179, #52647, #24138 ),
 ( #60143, #98682, #22165 ),
 ( #83150, #49090, #48094 ) ),
 .UNSPECIFIED., .F., .F., .F. ) 
 B_SPLINE_SURFACE_WITH_KNOTS ( ( 4, 2, 2, 2, 2, 2, 2, 2, 2, 2, 2, 2, 2, 2, 4 ),
 ( 3, 3 ),
 ( 0.000000000000000000, 0.001557317058375510058, 0.003114634116751020115, 0.006229268233502040231, 0.01245853646700408046, 0.01868780470050612069, 0.02491707293400816092, 0.03737560940101224138, 0.04983414586801632185, 0.06229268233502040231, 0.07475121880202448277, 0.08720975526902856323, 0.09343902350253061040, 0.09655365761928162704, 0.09966829173603264369 ),
 ( 0.000000000000000000, 1.000000000000000000 ),
 .UNSPECIFIED. ) 
 GEOMETRIC_REPRESENTATION_ITEM ( )  RATIONAL_B_SPLINE_SURFACE ( (
 ( 1.000000000000000000, 0.7071067811865445751, 1.000000000000000000),
 ( 1.000000000000000000, 0.7071067811865445751, 1.000000000000000000),
 ( 1.000000000000000000, 0.7071067811865475727, 1.000000000000000000),
 ( 1.000000000000000000, 0.7071067811865475727, 1.000000000000000000),
 ( 1.000000000000000000, 0.7071067811865451302, 1.000000000000000000),
 ( 1.000000000000000000, 0.7071067811865451302, 1.000000000000000000),
 ( 1.000000000000000000, 0.7071067811865500152, 1.000000000000000000),
 ( 1.000000000000000000, 0.7071067811865500152, 1.000000000000000000),
 ( 1.000000000000000000, 0.7071067811865475727, 1.000000000000000000),
 ( 1.000000000000000000, 0.7071067811865475727, 1.000000000000000000),
 ( 1.000000000000000000, 0.7071067811865450192, 1.000000000000000000),
 ( 1.000000000000000000, 0.7071067811865450192, 1.000000000000000000),
 ( 1.000000000000000000, 0.7071067811865475727, 1.000000000000000000),
 ( 1.000000000000000000, 0.7071067811865475727, 1.000000000000000000),
 ( 1.000000000000000000, 0.7071067811865473507, 1.000000000000000000),
 ( 1.000000000000000000, 0.7071067811865473507, 1.000000000000000000),
 ( 1.000000000000000000, 0.7071067811865451302, 1.000000000000000000),
 ( 1.000000000000000000, 0.7071067811865451302, 1.000000000000000000),
 ( 1.000000000000000000, 0.7071067811865475727, 1.000000000000000000),
 ( 1.000000000000000000, 0.7071067811865475727, 1.000000000000000000),
 ( 1.000000000000000000, 0.7071067811865475727, 1.000000000000000000),
 ( 1.000000000000000000, 0.7071067811865475727, 1.000000000000000000),
 ( 1.000000000000000000, 0.7071067811865475727, 1.000000000000000000),
 ( 1.000000000000000000, 0.7071067811865475727, 1.000000000000000000),
 ( 1.000000000000000000, 0.7071067811865475727, 1.000000000000000000),
 ( 1.000000000000000000, 0.7071067811865475727, 1.000000000000000000),
 ( 1.000000000000000000, 0.7071067811865475727, 1.000000000000000000),
 ( 1.000000000000000000, 0.7071067811865475727, 1.000000000000000000),
 ( 1.000000000000000000, 0.7071067811865475727, 1.000000000000000000),
 ( 1.000000000000000000, 0.7071067811865475727, 1.000000000000000000) ) ) 
 REPRESENTATION_ITEM ( '' )  SURFACE ( )  );
#94318=AXIS2_PLACEMENT_3D ( 'NONE', #32569, #71574, #77574 ) ;
#94324=DIRECTION ( 'NONE',  ( 0.000000000000000000, 0.000000000000000000, 1.000000000000000000 ) ) ;
#94331=VECTOR ( 'NONE', #7768, 1000.000000000000000 ) ;
#94334=AXIS2_PLACEMENT_3D ( 'NONE', #16497, #77968, #69494 ) ;
#94376=CARTESIAN_POINT ( 'NONE',  ( -8.332083457818344030, -7.290751590027323203, 3.750000000000000888 ) ) ;
#94379=DIRECTION ( 'NONE',  ( 1.000000000000000000, 0.000000000000000000, 1.214306433183763862E-14 ) ) ;
#94384=ORIENTED_EDGE ( 'NONE', *, *, #30368, .F. ) ;
#94416=CARTESIAN_POINT ( 'NONE',  ( -6.606690058690507961, -50.93246948815529151, -2.750000000000000000 ) ) ;
#94434=TOROIDAL_SURFACE ( 'NONE', #51327, 4.190000000000001279, 0.2500000000000000000 ) ;
#94439=CIRCLE ( 'NONE', #268, 0.2500000000000002220 ) ;
#94445=ORIENTED_EDGE ( 'NONE', *, *, #18998, .T. ) ;
#94446=CARTESIAN_POINT ( 'NONE',  ( -4.000000000000000000, 10.00000000000000000, 3.750000000000000000 ) ) ;
#94447=( NAMED_UNIT ( * ) SI_UNIT ( $, .STERADIAN. ) SOLID_ANGLE_UNIT ( ) );
#94456=DIRECTION ( 'NONE',  ( -1.000000000000000000, 0.000000000000000000, 0.000000000000000000 ) ) ;
#94463=LINE ( 'NONE', #34439, #63300 ) ;
#94470=DIRECTION ( 'NONE',  ( 0.000000000000000000, 0.000000000000000000, -1.000000000000000000 ) ) ;
#94484=LINE ( 'NONE', #94974, #92189 ) ;
#94487=EDGE_CURVE ( 'NONE', #7185, #20454, #24614, .T. ) ;
#94502=ORIENTED_EDGE ( 'NONE', *, *, #14029, .F. ) ;
#94506=ORIENTED_EDGE ( 'NONE', *, *, #25455, .F. ) ;
#94507=ORIENTED_EDGE ( 'NONE', *, *, #70442, .T. ) ;
#94508=FACE_OUTER_BOUND ( 'NONE', #58884, .T. ) ;
#94510=UNCERTAINTY_MEASURE_WITH_UNIT (LENGTH_MEASURE( 1.000000000000000082E-05 ), #13087, 'distance_accuracy_value', 'NONE');
#94529=VECTOR ( 'NONE', #26247, 1000.000000000000000 ) ;
#94537=AXIS2_PLACEMENT_3D ( 'NONE', #23593, #30068, #54057 ) ;
#94541=SURFACE_SIDE_STYLE ('',( #70574 ) ) ;
#94546=CIRCLE ( 'NONE', #37107, 2.899999999999999911 ) ;
#94548=CARTESIAN_POINT ( 'NONE',  ( -8.000000000000000000, 75.73428692542562146, 2.900000000000000355 ) ) ;
#94555=DIRECTION ( 'NONE',  ( 0.08715574274765151841, 0.9961946980917462113, 0.000000000000000000 ) ) ;
#94560=CARTESIAN_POINT ( 'NONE',  ( -7.037775641161837292, -86.26045154785950331, -3.750000000000000444 ) ) ;
#94561=DIRECTION ( 'NONE',  ( -0.000000000000000000, 0.000000000000000000, 1.000000000000000000 ) ) ;
#94574=ADVANCED_FACE ( 'NONE', ( #71667 ), #33642, .F. ) ;
#94576=LINE ( 'NONE', #40108, #66319 ) ;
#94578=ORIENTED_EDGE ( 'NONE', *, *, #1966, .F. ) ;
#94590=( NAMED_UNIT ( * ) PLANE_ANGLE_UNIT ( ) SI_UNIT ( $, .RADIAN. ) );
#94593=ORIENTED_EDGE ( 'NONE', *, *, #98248, .T. ) ;
#94608=ORIENTED_EDGE ( 'NONE', *, *, #84928, .T. ) ;
#94609=STYLED_ITEM ( 'NONE', ( #95229 ), #24342 ) ;
#94614=ORIENTED_EDGE ( 'NONE', *, *, #94239, .F. ) ;
#94618=MECHANICAL_DESIGN_GEOMETRIC_PRESENTATION_REPRESENTATION('',(#2081),#32371);
#94624=CARTESIAN_POINT ( 'NONE',  ( -3.521047174887395048, -6.414748048906915301, 2.500000000000000888 ) ) ;
#94626=CARTESIAN_POINT ( 'NONE',  ( 10.34946471139303092, -32.01331896743604233, 4.000000000000000000 ) ) ;
#94629=EDGE_CURVE ( 'NONE', #91827, #80133, #34628, .T. ) ;
#94632=ORIENTED_EDGE ( 'NONE', *, *, #98665, .F. ) ;
#94637=DIRECTION ( 'NONE',  ( -0.5150380749100542666, 1.049727191138618572E-16, -0.8571673007021122226 ) ) ;
#94644=DIRECTION ( 'NONE',  ( 0.000000000000000000, -1.000000000000000000, 0.000000000000000000 ) ) ;
#94648=ORIENTED_EDGE ( 'NONE', *, *, #65647, .F. ) ;
#94662=CARTESIAN_POINT ( 'NONE',  ( -8.000000000000000000, 1.019547802438466100, -4.000000000000000000 ) ) ;
#94669=MECHANICAL_DESIGN_GEOMETRIC_PRESENTATION_REPRESENTATION('',(#24461),#80328);
#94684=STYLED_ITEM ( 'NONE', ( #7633 ), #92799 ) ;
#94690=EDGE_CURVE ( 'NONE', #27652, #97731, #98069, .T. ) ;
#94699=DIRECTION ( 'NONE',  ( -0.000000000000000000, 0.000000000000000000, 1.000000000000000000 ) ) ;
#94707=CARTESIAN_POINT ( 'NONE',  ( -6.000000000000000000, 78.07179676972447169, -4.250000000000000000 ) ) ;
#94717=DIRECTION ( 'NONE',  ( -1.000000000000000000, 0.000000000000000000, 0.000000000000000000 ) ) ;
#94718=VERTEX_POINT ( 'NONE', #50135 ) ;
#94730=ORIENTED_EDGE ( 'NONE', *, *, #68637, .F. ) ;
#94738=DIRECTION ( 'NONE',  ( 1.000000000000000000, 0.000000000000000000, 0.000000000000000000 ) ) ;
#94749=( NAMED_UNIT ( * ) SI_UNIT ( $, .STERADIAN. ) SOLID_ANGLE_UNIT ( ) );
#94765=CARTESIAN_POINT ( 'NONE',  ( -9.343156623282764528, 88.41679554545861208, 5.273290232418111678 ) ) ;
#94774=CARTESIAN_POINT ( 'NONE',  ( 8.879999999999991900, 76.07179676972447169, -6.500000000000000888 ) ) ;
#94777=CARTESIAN_POINT ( 'NONE',  ( 6.757757868617466634, -58.31753767725378879, 3.750000000000000888 ) ) ;
#94779=COLOUR_RGB ( '', 0.72549020, 0.75294118, 0.79215686) ;
#94780=DIRECTION ( 'NONE',  ( 1.000000000000000000, 0.000000000000000000, 0.000000000000000000 ) ) ;
#94782=CARTESIAN_POINT ( 'NONE',  ( -6.982525766850298687, -88.11956318484570261, 2.750000000000000444 ) ) ;
#94787=CARTESIAN_POINT ( 'NONE',  ( -8.004790597918161055, 84.51838969325523010, -3.750000002001242283 ) ) ;
#94796=DIRECTION ( 'NONE',  ( -0.000000000000000000, -1.000000000000000000, -0.000000000000000000 ) ) ;
#94804=DIRECTION ( 'NONE',  ( -1.000000000000000000, -1.257402221000611116E-16, 0.000000000000000000 ) ) ;
#94806=CARTESIAN_POINT ( 'NONE',  ( 6.579634127946655475, -87.99828267815715321, -3.750000000000000000 ) ) ;
#94812=( GEOMETRIC_REPRESENTATION_CONTEXT ( 3 ) GLOBAL_UNCERTAINTY_ASSIGNED_CONTEXT ( ( #43473 ) ) GLOBAL_UNIT_ASSIGNED_CONTEXT ( ( #33300, #87292, #95287 ) ) REPRESENTATION_CONTEXT ( 'NONE', 'WORKASPACE' ) );
#94817=DIRECTION ( 'NONE',  ( 0.000000000000000000, 1.000000000000000000, 0.000000000000000000 ) ) ;
#94822=CARTESIAN_POINT ( 'NONE',  ( 4.130000000000002558, 1.019547802438464545, -2.500000000000000000 ) ) ;
#94824=AXIS2_PLACEMENT_3D ( 'NONE', #13621, #22123, #76584 ) ;
#94827=EDGE_LOOP ( 'NONE', ( #75064, #84188, #53460, #79400 ) ) ;
#94830=ORIENTED_EDGE ( 'NONE', *, *, #71236, .T. ) ;
#94832=DIRECTION ( 'NONE',  ( 0.000000000000000000, 0.000000000000000000, -1.000000000000000000 ) ) ;
#94843=ADVANCED_FACE ( 'NONE', ( #35123 ), #13124, .T. ) ;
#94848=ORIENTED_EDGE ( 'NONE', *, *, #13478, .T. ) ;
#94864=EDGE_CURVE ( 'NONE', #73802, #67464, #5640, .T. ) ;
#94872=DIRECTION ( 'NONE',  ( -0.000000000000000000, -0.000000000000000000, -1.000000000000000000 ) ) ;
#94879=( NAMED_UNIT ( * ) PLANE_ANGLE_UNIT ( ) SI_UNIT ( $, .RADIAN. ) );
#94887=CIRCLE ( 'NONE', #51794, 3.000000000000002665 ) ;
#94898=CARTESIAN_POINT ( 'NONE',  ( 11.44532481276809577, -77.50732122612269848, 3.750000000000000444 ) ) ;
#94900=CARTESIAN_POINT ( 'NONE',  ( 1.379999999999981908, 20.99999999999999645, 1.249999999999987121 ) ) ;
#94907=CARTESIAN_POINT ( 'NONE',  ( -3.627483523208788530, -3.617667194775422423, -2.499999999999798383 ) ) ;
#94913=CARTESIAN_POINT ( 'NONE',  ( 4.573751236700658751, -6.413519960483383464, -3.750000000000000000 ) ) ;
#94915=FACE_OUTER_BOUND ( 'NONE', #26587, .T. ) ;
#94923=DIRECTION ( 'NONE',  ( 0.000000000000000000, 0.000000000000000000, -1.000000000000000000 ) ) ;
#94934=DIRECTION ( 'NONE',  ( -0.08715574274765129636, -0.9961946980917462113, 0.000000000000000000 ) ) ;
#94936=LINE ( 'NONE', #94446, #96414 ) ;
#94952=EDGE_CURVE ( 'NONE', #64082, #15746, #38948, .T. ) ;
#94961=EDGE_CURVE ( 'NONE', #39745, #95826, #61576, .T. ) ;
#94962=( GEOMETRIC_REPRESENTATION_CONTEXT ( 3 ) GLOBAL_UNCERTAINTY_ASSIGNED_CONTEXT ( ( #52459 ) ) GLOBAL_UNIT_ASSIGNED_CONTEXT ( ( #25346, #76360, #23374 ) ) REPRESENTATION_CONTEXT ( 'NONE', 'WORKASPACE' ) );
#94965=ORIENTED_EDGE ( 'NONE', *, *, #58588, .T. ) ;
#94974=CARTESIAN_POINT ( 'NONE',  ( 0.000000000000000000, 69.99999999999998579, 6.250000000000000000 ) ) ;
#94987=AXIS2_PLACEMENT_3D ( 'NONE', #85144, #4110, #35576 ) ;
#94992=VERTEX_POINT ( 'NONE', #38600 ) ;
#94994=CARTESIAN_POINT ( 'NONE',  ( -5.999999999999994671, 43.00000000000000000, 6.250000000000000000 ) ) ;
#95002=( LENGTH_UNIT ( ) NAMED_UNIT ( * ) SI_UNIT ( .MILLI., .METRE. ) );
#95005=ORIENTED_EDGE ( 'NONE', *, *, #69909, .F. ) ;
#95017=ORIENTED_EDGE ( 'NONE', *, *, #86978, .T. ) ;
#95018=COLOUR_RGB ( '', 0.72549020, 0.75294118, 0.79215686) ;
#95025=CARTESIAN_POINT ( 'NONE',  ( -12.16982443903230759, 90.48687232357862342, 7.214476785723132224 ) ) ;
#95038=CARTESIAN_POINT ( 'NONE',  ( 17.99999999999999645, 78.80384757729335377, -3.999999999999996891 ) ) ;
#95045=CARTESIAN_POINT ( 'NONE',  ( -4.536162299966319367, -17.54167381550513838, -3.750000000000000000 ) ) ;
#95046=FACE_OUTER_BOUND ( 'NONE', #29347, .T. ) ;
#95060=FACE_OUTER_BOUND ( 'NONE', #38021, .T. ) ;
#95061=CARTESIAN_POINT ( 'NONE',  ( -10.88853822400146854, 46.97908644289115898, -3.000000000000000000 ) ) ;
#95068=AXIS2_PLACEMENT_3D ( 'NONE', #70861, #85856, #86837 ) ;
#95076=EDGE_CURVE ( 'NONE', #40011, #74673, #45598, .T. ) ;
#95078=ORIENTED_EDGE ( 'NONE', *, *, #69598, .T. ) ;
#95089=( GEOMETRIC_REPRESENTATION_CONTEXT ( 3 ) GLOBAL_UNCERTAINTY_ASSIGNED_CONTEXT ( ( #33501 ) ) GLOBAL_UNIT_ASSIGNED_CONTEXT ( ( #22022, #66516, #90980 ) ) REPRESENTATION_CONTEXT ( 'NONE', 'WORKASPACE' ) );
#95095=ORIENTED_EDGE ( 'NONE', *, *, #74804, .F. ) ;
#95099=SURFACE_SIDE_STYLE ('',( #73084 ) ) ;
#95106=CARTESIAN_POINT ( 'NONE',  ( 11.43665280317779676, -81.62088987012548102, 3.750000000000000000 ) ) ;
#95108=DIRECTION ( 'NONE',  ( 0.000000000000000000, -0.000000000000000000, -1.000000000000000000 ) ) ;
#95113=FACE_OUTER_BOUND ( 'NONE', #5465, .T. ) ;
#95114=FACE_OUTER_BOUND ( 'NONE', #16955, .T. ) ;
#95124=CARTESIAN_POINT ( 'NONE',  ( -6.000000000000000000, 78.07179676972447169, -6.250000000000000000 ) ) ;
#95148=COLOUR_RGB ( '', 0.09019608, 0.27058824, 0.51372549) ;
#95150=ADVANCED_FACE ( 'NONE', ( #91092 ), #69098, .T. ) ;
#95165=CARTESIAN_POINT ( 'NONE',  ( -9.000000000000003553, 80.99999999999994316, 0.000000000000000000 ) ) ;
#95166=CARTESIAN_POINT ( 'NONE',  ( 6.452519493965914954, -47.68837976023561964, 3.750000000000001776 ) ) ;
#95172=CARTESIAN_POINT ( 'NONE',  ( -6.982525766850298687, -88.11956318484570261, 3.750000000000000000 ) ) ;
#95174=ADVANCED_FACE ( 'NONE', ( #97641 ), #15123, .F. ) ;
#95177=ORIENTED_EDGE ( 'NONE', *, *, #51630, .F. ) ;
#95222=MECHANICAL_DESIGN_GEOMETRIC_PRESENTATION_REPRESENTATION('',(#31353),#93662);
#95223=DIRECTION ( 'NONE',  ( 0.000000000000000000, -1.000000000000000000, 0.000000000000000000 ) ) ;
#95229=PRESENTATION_STYLE_ASSIGNMENT (( #3769 ) ) ;
#95230=ADVANCED_FACE ( 'NONE', ( #78068 ), #74179, .T. ) ;
#95240=AXIS2_PLACEMENT_3D ( 'NONE', #63776, #39823, #94780 ) ;
#95242=EDGE_CURVE ( 'NONE', #25004, #38304, #10072, .T. ) ;
#95250=CARTESIAN_POINT ( 'NONE',  ( -12.24686443627862964, 90.44926614966664147, 7.163467944141830301 ) ) ;
#95270=STYLED_ITEM ( 'NONE', ( #58583 ), #41174 ) ;
#95272=DIRECTION ( 'NONE',  ( -1.000000000000000000, -0.000000000000000000, -0.000000000000000000 ) ) ;
#95273=ORIENTED_EDGE ( 'NONE', *, *, #22580, .T. ) ;
#95276=CARTESIAN_POINT ( 'NONE',  ( -6.732636091893172470, -88.11213685669366669, -3.250000000000000000 ) ) ;
#95277=CARTESIAN_POINT ( 'NONE',  ( -8.352412229647901754, 86.23350694210130030, -4.048761466749791538 ) ) ;
#95280=EDGE_CURVE ( 'NONE', #875, #95488, #17090, .T. ) ;
#95281=CIRCLE ( 'NONE', #15522, 0.5000000000000004441 ) ;
#95287=( NAMED_UNIT ( * ) SI_UNIT ( $, .STERADIAN. ) SOLID_ANGLE_UNIT ( ) );
#95288=( NAMED_UNIT ( * ) PLANE_ANGLE_UNIT ( ) SI_UNIT ( $, .RADIAN. ) );
#95294=FILL_AREA_STYLE ('',( #18820 ) ) ;
#95297=DIRECTION ( 'NONE',  ( 0.000000000000000000, 0.000000000000000000, -1.000000000000000000 ) ) ;
#95302=UNCERTAINTY_MEASURE_WITH_UNIT (LENGTH_MEASURE( 1.000000000000000082E-05 ), #16146, 'distance_accuracy_value', 'NONE');
#95309=EDGE_CURVE ( 'NONE', #80996, #42048, #31078, .T. ) ;
#95311=AXIS2_PLACEMENT_3D ( 'NONE', #4634, #81589, #43105 ) ;
#95318=EDGE_CURVE ( 'NONE', #57591, #9146, #2594, .T. ) ;
#95325=CARTESIAN_POINT ( 'NONE',  ( 1.379999999999981908, 20.99999999999999645, -1.249999999999987121 ) ) ;
#95329=STYLED_ITEM ( 'NONE', ( #63087 ), #67519 ) ;
#95332=CARTESIAN_POINT ( 'NONE',  ( -9.000000000000001776, 80.99999999999994316, 1.249999999999987121 ) ) ;
#95339=ORIENTED_EDGE ( 'NONE', *, *, #60871, .T. ) ;
#95368=EDGE_CURVE ( 'NONE', #76544, #87452, #24096, .T. ) ;
#95381=LINE ( 'NONE', #3411, #4111 ) ;
#95395=CARTESIAN_POINT ( 'NONE',  ( 11.13571380284232326, -94.04086316623734376, 3.750000000000001332 ) ) ;
#95406=CARTESIAN_POINT ( 'NONE',  ( -3.638343494402133782, -8.270261767329072811, -2.500000000000000888 ) ) ;
#95414=ORIENTED_EDGE ( 'NONE', *, *, #12112, .F. ) ;
#95415=CARTESIAN_POINT ( 'NONE',  ( 7.185087194272973932, -80.58596676771932721, -4.000000000000000000 ) ) ;
#95416=CARTESIAN_POINT ( 'NONE',  ( -19.00000000000000000, 75.76920769491739804, 2.900000000000000355 ) ) ;
#95420=DIRECTION ( 'NONE',  ( 0.000000000000000000, 0.000000000000000000, 1.000000000000000000 ) ) ;
#95427=DIRECTION ( 'NONE',  ( 0.000000000000000000, 0.000000000000000000, -1.000000000000000000 ) ) ;
#95430=UNCERTAINTY_MEASURE_WITH_UNIT (LENGTH_MEASURE( 1.000000000000000082E-05 ), #37427, 'distance_accuracy_value', 'NONE');
#95438=ORIENTED_EDGE ( 'NONE', *, *, #84161, .F. ) ;
#95440=LINE ( 'NONE', #95940, #53287 ) ;
#95449=VERTEX_POINT ( 'NONE', #39096 ) ;
#95460=SURFACE_STYLE_FILL_AREA ( #13428 ) ;
#95471=ADVANCED_BREP_SHAPE_REPRESENTATION ( '', ( #9364, #74641, #40953, #27931 ), #34259 ) ;
#95488=VERTEX_POINT ( 'NONE', #55572 ) ;
#95496=DIRECTION ( 'NONE',  ( 0.000000000000000000, 1.000000000000000000, 0.000000000000000000 ) ) ;
#95526=VERTEX_POINT ( 'NONE', #20021 ) ;
#95528=( NAMED_UNIT ( * ) PLANE_ANGLE_UNIT ( ) SI_UNIT ( $, .RADIAN. ) );
#95537=CARTESIAN_POINT ( 'NONE',  ( -6.787878914541004782, -86.25326249609902618, -2.499999999999999556 ) ) ;
#95542=CIRCLE ( 'NONE', #18891, 2.899999999999999023 ) ;
#95544=DIRECTION ( 'NONE',  ( -0.000000000000000000, 1.000000000000000000, -0.000000000000000000 ) ) ;
#95548=CARTESIAN_POINT ( 'NONE',  ( 18.00000000000000000, 78.80384757729335377, -3.750000000000000444 ) ) ;
#95553=CARTESIAN_POINT ( 'NONE',  ( -6.607077646681807082, -50.94230861868440741, -3.750000000000000444 ) ) ;
#95568=EDGE_CURVE ( 'NONE', #44437, #90212, #57575, .T. ) ;
#95569=DIRECTION ( 'NONE',  ( -1.000000000000000000, 0.000000000000000000, 0.000000000000000000 ) ) ;
#95572=ORIENTED_EDGE ( 'NONE', *, *, #68637, .T. ) ;
#95579=DIRECTION ( 'NONE',  ( 4.683753385137374737E-14, -1.000000000000000000, 0.000000000000000000 ) ) ;
#95596=SURFACE_STYLE_USAGE ( .BOTH. , #88078 ) ;
#95602=ORIENTED_EDGE ( 'NONE', *, *, #45830, .F. ) ;
#95612=EDGE_LOOP ( 'NONE', ( #13357, #32232, #45360, #95177 ) ) ;
#95615=CARTESIAN_POINT ( 'NONE',  ( 10.79852199278004754, -95.56374241347876364, 4.000000000000000000 ) ) ;
#95619=VERTEX_POINT ( 'NONE', #5029 ) ;
#95626=ORIENTED_EDGE ( 'NONE', *, *, #22946, .T. ) ;
#95629=ADVANCED_FACE ( 'NONE', ( #87533 ), #88021, .T. ) ;
#95630=CARTESIAN_POINT ( 'NONE',  ( 11.57153612472183646, -43.60599867514397943, 3.750000000000000000 ) ) ;
#95646=ADVANCED_FACE ( 'NONE', ( #96033 ), #65511, .T. ) ;
#95648=SURFACE_STYLE_FILL_AREA ( #42643 ) ;
#95654=CARTESIAN_POINT ( 'NONE',  ( -11.26382985214544696, -93.42670896122723434, -3.999999999999098943 ) ) ;
#95656=DIRECTION ( 'NONE',  ( -0.000000000000000000, 1.000000000000000000, -0.000000000000000000 ) ) ;
#95672=CARTESIAN_POINT ( 'NONE',  ( 6.878063601867475008, -66.29791949882819324, 2.750000000000000000 ) ) ;
#95680=DIRECTION ( 'NONE',  ( 0.000000000000000000, 0.000000000000000000, 1.000000000000000000 ) ) ;
#95681=CARTESIAN_POINT ( 'NONE',  ( 2.550000000000003819, 99.99999999999998579, -8.525133428036873795 ) ) ;
#95688=ORIENTED_EDGE ( 'NONE', *, *, #39123, .T. ) ;
#95700=B_SPLINE_CURVE_WITH_KNOTS ( 'NONE', 3,
 ( #28393, #50894, #11056, #88899, #56074, #79052, #10564, #65887, #13390, #20408, #41576, #36391, #89388, #72044, #20902, #51391, #74369, #97403, #7388, #37886, #92344, #61349, #400, #7876, #22883, #14392, #30350, #23870 ),
 .UNSPECIFIED., .F., .F.,
 ( 4, 2, 2, 2, 2, 2, 2, 2, 2, 2, 2, 2, 2, 4 ),
 ( 0.000000000000000000, 0.001557342785199824619, 0.003114685570399649238, 0.006229371140799340109, 0.01245874228159868022, 0.02491748456319740554, 0.03737622684479612045, 0.04983496912639484577, 0.06229371140799356416, 0.07475245368959228254, 0.08721119597119100786, 0.09344056711199036358, 0.09655525268239005532, 0.09966993825278973318 ),
 .UNSPECIFIED. ) ;
#95707=( NAMED_UNIT ( * ) PLANE_ANGLE_UNIT ( ) SI_UNIT ( $, .RADIAN. ) );
#95714=AXIS2_PLACEMENT_3D ( 'NONE', #5919, #97425, #26934 ) ;
#95728=PLANE ( 'NONE',  #73485 ) ;
#95736=LINE ( 'NONE', #19728, #49842 ) ;
#95737=DIRECTION ( 'NONE',  ( 0.000000000000000000, 0.000000000000000000, 1.000000000000000000 ) ) ;
#95743=SPHERICAL_SURFACE ( 'NONE', #77051, 0.2500000000000000000 ) ;
#95766=EDGE_CURVE ( 'NONE', #71601, #79717, #71008, .T. ) ;
#95778=( GEOMETRIC_REPRESENTATION_CONTEXT ( 3 ) GLOBAL_UNCERTAINTY_ASSIGNED_CONTEXT ( ( #76114 ) ) GLOBAL_UNIT_ASSIGNED_CONTEXT ( ( #94242, #18263, #56741 ) ) REPRESENTATION_CONTEXT ( 'NONE', 'WORKASPACE' ) );
#95782=CARTESIAN_POINT ( 'NONE',  ( 11.10000000000000142, 98.49999999999998579, -8.000000000000000000 ) ) ;
#95783=ORIENTED_EDGE ( 'NONE', *, *, #23470, .F. ) ;
#95789=DIRECTION ( 'NONE',  ( -0.000000000000000000, -0.000000000000000000, -1.000000000000000000 ) ) ;
#95794=CYLINDRICAL_SURFACE ( 'NONE', #3831, 0.2500000000000002220 ) ;
#95795=CARTESIAN_POINT ( 'NONE',  ( -9.000000000000001776, 83.99999999999994316, 3.000000000000000000 ) ) ;
#95807=FILL_AREA_STYLE ('',( #80300 ) ) ;
#95813=PRESENTATION_STYLE_ASSIGNMENT (( #11315 ) ) ;
#95825=FACE_OUTER_BOUND ( 'NONE', #63610, .T. ) ;
#95826=VERTEX_POINT ( 'NONE', #91480 ) ;
#95873=( NAMED_UNIT ( * ) PLANE_ANGLE_UNIT ( ) SI_UNIT ( $, .RADIAN. ) );
#95876=DIRECTION ( 'NONE',  ( -0.000000000000000000, -0.000000000000000000, 1.000000000000000000 ) ) ;
#95881=ORIENTED_EDGE ( 'NONE', *, *, #42334, .F. ) ;
#95883=FILL_AREA_STYLE ('',( #44333 ) ) ;
#95884=CIRCLE ( 'NONE', #32042, 7.250000000000002665 ) ;
#95898=FACE_OUTER_BOUND ( 'NONE', #53058, .T. ) ;
#95905=CARTESIAN_POINT ( 'NONE',  ( -18.89999999999999147, 91.25000000000000000, 7.750000000000000000 ) ) ;
#95912=CARTESIAN_POINT ( 'NONE',  ( -3.250000001579299802, 0.08818787376460503202, -2.500000000000000000 ) ) ;
#95922=CARTESIAN_POINT ( 'NONE',  ( -7.366188783701793419, -80.69039970148938323, 3.999999999999999112 ) ) ;
#95924=DIRECTION ( 'NONE',  ( 0.000000000000000000, 0.000000000000000000, -1.000000000000000000 ) ) ;
#95932=CARTESIAN_POINT ( 'NONE',  ( 8.879999999999999005, 20.99999999999999645, -1.249999999999987121 ) ) ;
#95940=CARTESIAN_POINT ( 'NONE',  ( -8.000000000000000000, 80.07179676972448590, 4.250000000000000000 ) ) ;
#95947=EDGE_LOOP ( 'NONE', ( #5109, #15329 ) ) ;
#95954=ORIENTED_EDGE ( 'NONE', *, *, #87719, .F. ) ;
#95957=CARTESIAN_POINT ( 'NONE',  ( 4.630000001262032150, 0.09071174558778491437, 4.000000000000000000 ) ) ;
#95958=DIRECTION ( 'NONE',  ( 0.000000000000000000, 0.000000000000000000, -1.000000000000000000 ) ) ;
#95967=PLANE ( 'NONE',  #70237 ) ;
#95972=STYLED_ITEM ( 'NONE', ( #13723 ), #33401 ) ;
#96008=DIRECTION ( 'NONE',  ( -0.000000000000000000, 0.000000000000000000, 1.000000000000000000 ) ) ;
#96010=DIRECTION ( 'NONE',  ( 1.000000000000000000, 0.000000000000000000, 0.000000000000000000 ) ) ;
#96019=FILL_AREA_STYLE_COLOUR ( '', #37826 ) ;
#96033=FACE_OUTER_BOUND ( 'NONE', #94173, .T. ) ;
#96039=AXIS2_PLACEMENT_3D ( 'NONE', #71179, #33156, #63650 ) ;
#96046=CARTESIAN_POINT ( 'NONE',  ( 18.00000000000000000, 78.53751499213353782, -3.955843470927832950 ) ) ;
#96051=CARTESIAN_POINT ( 'NONE',  ( -7.124966299160218952, -78.82422258446059971, -3.750000000000000000 ) ) ;
#96070=( NAMED_UNIT ( * ) PLANE_ANGLE_UNIT ( ) SI_UNIT ( $, .RADIAN. ) );
#96087=ORIENTED_EDGE ( 'NONE', *, *, #76771, .F. ) ;
#96088=EDGE_LOOP ( 'NONE', ( #8871, #55007, #72074, #51079 ) ) ;
#96096=AXIS2_PLACEMENT_3D ( 'NONE', #55335, #56806, #54830 ) ;
#96097=EDGE_CURVE ( 'NONE', #96723, #18240, #94887, .T. ) ;
#96102=VERTEX_POINT ( 'NONE', #86446 ) ;
#96108=CYLINDRICAL_SURFACE ( 'NONE', #40990, 10.00000000000000178 ) ;
#96112=DIRECTION ( 'NONE',  ( 0.000000000000000000, 1.000000000000000000, 0.000000000000000000 ) ) ;
#96113=AXIS2_PLACEMENT_3D ( 'NONE', #24104, #45609, #1117 ) ;
#96121=CARTESIAN_POINT ( 'NONE',  ( -5.812563760649267941, -35.09659463721938977, 3.750000000000000444 ) ) ;
#96135=EDGE_CURVE ( 'NONE', #86711, #21427, #92453, .T. ) ;
#96139=ORIENTED_EDGE ( 'NONE', *, *, #57620, .T. ) ;
#96146=PLANE ( 'NONE',  #37628 ) ;
#96158=SURFACE_STYLE_FILL_AREA ( #73630 ) ;
#96169=ORIENTED_EDGE ( 'NONE', *, *, #42353, .T. ) ;
#96171=CARTESIAN_POINT ( 'NONE',  ( 18.00000000000000000, 91.21610151837452918, -8.000000000000000000 ) ) ;
#96172=CARTESIAN_POINT ( 'NONE',  ( 6.452519493965914954, -47.68837976023561964, 2.750000000000000000 ) ) ;
#96181=ORIENTED_EDGE ( 'NONE', *, *, #43235, .T. ) ;
#96187=LINE ( 'NONE', #40721, #24606 ) ;
#96193=CARTESIAN_POINT ( 'NONE',  ( -11.02874191836853512, -96.54482102863701698, 3.750000000000000000 ) ) ;
#96203=MECHANICAL_DESIGN_GEOMETRIC_PRESENTATION_REPRESENTATION('',(#56237),#81755);
#96205=ORIENTED_EDGE ( 'NONE', *, *, #59826, .T. ) ;
#96206=CARTESIAN_POINT ( 'NONE',  ( 10.83696084481538691, -98.17058944465519232, 3.750000000000000000 ) ) ;
#96207=CIRCLE ( 'NONE', #97802, 11.15000000000026326 ) ;
#96209=ORIENTED_EDGE ( 'NONE', *, *, #3440, .T. ) ;
#96216=ADVANCED_FACE ( 'NONE', ( #24476 ), #82935, .T. ) ;
#96222=EDGE_CURVE ( 'NONE', #7152, #55464, #4914, .T. ) ;
#96234=VERTEX_POINT ( 'NONE', #72897 ) ;
#96241=LINE ( 'NONE', #5243, #6824 ) ;
#96248=CYLINDRICAL_SURFACE ( 'NONE', #59178, 2.000000000000000000 ) ;
#96252=DIRECTION ( 'NONE',  ( -0.000000000000000000, -1.000000000000000000, -0.000000000000000000 ) ) ;
#96255=EDGE_CURVE ( 'NONE', #40043, #6847, #81388, .T. ) ;
#96259=CARTESIAN_POINT ( 'NONE',  ( -12.29167862326001348, 90.46743899975659531, 7.079701151216531763 ) ) ;
#96263=ORIENTED_EDGE ( 'NONE', *, *, #79818, .T. ) ;
#96264=VECTOR ( 'NONE', #31426, 1000.000000000000000 ) ;
#96275=VECTOR ( 'NONE', #74240, 1000.000000000000000 ) ;
#96285=CARTESIAN_POINT ( 'NONE',  ( -10.89045396206015504, 89.68015320059716089, -6.284968870999087187 ) ) ;
#96295=LINE ( 'NONE', #57774, #76388 ) ;
#96303=DIRECTION ( 'NONE',  ( -1.000000000000000000, 0.000000000000000000, 0.000000000000000000 ) ) ;
#96309=AXIS2_PLACEMENT_3D ( 'NONE', #79167, #41196, #40193 ) ;
#96329=FACE_OUTER_BOUND ( 'NONE', #15095, .T. ) ;
#96339=( NAMED_UNIT ( * ) PLANE_ANGLE_UNIT ( ) SI_UNIT ( $, .RADIAN. ) );
#96342=EDGE_CURVE ( 'NONE', #76829, #44664, #14975, .T. ) ;
#96344=CIRCLE ( 'NONE', #42027, 2.000000000000000888 ) ;
#96348=ADVANCED_FACE ( 'NONE', ( #75365 ), #28870, .F. ) ;
#96349=CIRCLE ( 'NONE', #93111, 2.999999999999997335 ) ;
#96352=COLOUR_RGB ( '', 0.09019608, 0.27058824, 0.51372549) ;
#96359=ORIENTED_EDGE ( 'NONE', *, *, #41929, .F. ) ;
#96362=DIRECTION ( 'NONE',  ( 0.000000000000000000, 0.000000000000000000, 1.000000000000000000 ) ) ;
#96366=ORIENTED_EDGE ( 'NONE', *, *, #82692, .T. ) ;
#96369=CARTESIAN_POINT ( 'NONE',  ( -13.80022967267210987, 90.89648642031431791, -7.755896862406649106 ) ) ;
#96386=ORIENTED_EDGE ( 'NONE', *, *, #24734, .F. ) ;
#96400=CARTESIAN_POINT ( 'NONE',  ( 8.879999999999991900, 76.07179676972447169, -6.500000000000000888 ) ) ;
#96401=DIRECTION ( 'NONE',  ( 0.000000000000000000, 0.000000000000000000, 1.000000000000000000 ) ) ;
#96403=STYLED_ITEM ( 'NONE', ( #88771 ), #96915 ) ;
#96406=DIRECTION ( 'NONE',  ( 0.000000000000000000, 0.000000000000000000, -1.000000000000000000 ) ) ;
#96414=VECTOR ( 'NONE', #49431, 1000.000000000000000 ) ;
#96415=CARTESIAN_POINT ( 'NONE',  ( 5.365144748710862110, -17.52568678401977920, -4.000000000000000000 ) ) ;
#96422=DIRECTION ( 'NONE',  ( 0.000000000000000000, -1.000000000000000000, 0.000000000000000000 ) ) ;
#96430=SURFACE_STYLE_FILL_AREA ( #35407 ) ;
#96435=ADVANCED_FACE ( 'NONE', ( #74875 ), #20901, .T. ) ;
#96448=ORIENTED_EDGE ( 'NONE', *, *, #13324, .T. ) ;
#96453=ORIENTED_EDGE ( 'NONE', *, *, #16828, .F. ) ;
#96456=SURFACE_SIDE_STYLE ('',( #36431 ) ) ;
#96457=PLANE ( 'NONE',  #32982 ) ;
#96479=AXIS2_PLACEMENT_3D ( 'NONE', #94994, #87498, #19013 ) ;
#96487=VERTEX_POINT ( 'NONE', #44861 ) ;
#96498=ORIENTED_EDGE ( 'NONE', *, *, #10801, .T. ) ;
#96504=UNCERTAINTY_MEASURE_WITH_UNIT (LENGTH_MEASURE( 1.000000000000000082E-05 ), #80794, 'distance_accuracy_value', 'NONE');
#96509=SURFACE_STYLE_USAGE ( .BOTH. , #72990 ) ;
#96511=DIRECTION ( 'NONE',  ( 1.000000000000000000, 0.000000000000000000, 0.000000000000000000 ) ) ;
#96513=SPHERICAL_SURFACE ( 'NONE', #40388, 0.2500000000000000000 ) ;
#96521=VECTOR ( 'NONE', #61255, 1000.000000000000000 ) ;
#96522=EDGE_CURVE ( 'NONE', #49230, #30576, #68378, .T. ) ;
#96535=CARTESIAN_POINT ( 'NONE',  ( -4.285591316845103194, -17.54293119412274038, -2.500000000000001776 ) ) ;
#96546=ADVANCED_FACE ( 'NONE', ( #51390 ), #81876, .T. ) ;
#96550=EDGE_CURVE ( 'NONE', #91827, #59823, #58051, .T. ) ;
#96554=DIRECTION ( 'NONE',  ( 0.000000000000000000, 1.000000000000000000, -0.000000000000000000 ) ) ;
#96576=LINE ( 'NONE', #53019, #1273 ) ;
#96580=EDGE_CURVE ( 'NONE', #87437, #50168, #85334, .T. ) ;
#96586=ORIENTED_EDGE ( 'NONE', *, *, #75964, .T. ) ;
#96587=( BOUNDED_CURVE ( )  B_SPLINE_CURVE ( 3, ( #12087, #34088, #26593, #35070 ),
 .UNSPECIFIED., .F., .F. ) 
 B_SPLINE_CURVE_WITH_KNOTS ( ( 4, 4 ),
 ( 4.712388980384680792, 6.283185307179586232 ),
 .UNSPECIFIED. ) 
 CURVE ( )  GEOMETRIC_REPRESENTATION_ITEM ( )  RATIONAL_B_SPLINE_CURVE ( ( 1.000000000000000000, 0.8047378541243628280, 0.8047378541243628280, 1.000000000000000000 ) ) 
 REPRESENTATION_ITEM ( '' )  );
#96589=PRESENTATION_STYLE_ASSIGNMENT (( #66061 ) ) ;
#96611=CARTESIAN_POINT ( 'NONE',  ( -8.900000000000002132, 80.99999999999994316, 0.000000000000000000 ) ) ;
#96612=ORIENTED_EDGE ( 'NONE', *, *, #57903, .T. ) ;
#96620=( NAMED_UNIT ( * ) PLANE_ANGLE_UNIT ( ) SI_UNIT ( $, .RADIAN. ) );
#96644=PLANE ( 'NONE',  #20855 ) ;
#96647=CARTESIAN_POINT ( 'NONE',  ( -6.000000000000014211, 80.07179676972448590, 6.250000000000000000 ) ) ;
#96655=CARTESIAN_POINT ( 'NONE',  ( -6.599999999999995204, -97.00000000000000000, 3.750000000000000000 ) ) ;
#96663=AXIS2_PLACEMENT_3D ( 'NONE', #29734, #92223, #53237 ) ;
#96670=VERTEX_POINT ( 'NONE', #69355 ) ;
#96685=CARTESIAN_POINT ( 'NONE',  ( 4.130000000000002558, 1.019547802438462547, 2.500000000000000000 ) ) ;
#96688=VERTEX_POINT ( 'NONE', #16847 ) ;
#96696=CARTESIAN_POINT ( 'NONE',  ( -10.91898769996044827, -97.58648078763678768, 3.750000000000000000 ) ) ;
#96701=AXIS2_PLACEMENT_3D ( 'NONE', #59710, #96252, #97747 ) ;
#96704=CARTESIAN_POINT ( 'NONE',  ( 3.969999999999999751, 37.00000000000000000, -2.750000000000000000 ) ) ;
#96709=ORIENTED_EDGE ( 'NONE', *, *, #73587, .F. ) ;
#96717=AXIS2_PLACEMENT_3D ( 'NONE', #69960, #1479, #70452 ) ;
#96723=VERTEX_POINT ( 'NONE', #38864 ) ;
#96729=PLANE ( 'NONE',  #36825 ) ;
#96731=CIRCLE ( 'NONE', #26476, 0.2500000000000002220 ) ;
#96733=ORIENTED_EDGE ( 'NONE', *, *, #17431, .T. ) ;
#96734=AXIS2_PLACEMENT_3D ( 'NONE', #43291, #65291, #35294 ) ;
#96737=DIRECTION ( 'NONE',  ( 1.000000000000000000, 0.000000000000000000, 0.000000000000000000 ) ) ;
#96741=FILL_AREA_STYLE_COLOUR ( '', #13174 ) ;
#96747=DIRECTION ( 'NONE',  ( 0.000000000000000000, -1.000000000000000000, 0.000000000000000000 ) ) ;
#96750=DIRECTION ( 'NONE',  ( 1.000000000000000000, 1.273191542001295551E-15, 0.000000000000000000 ) ) ;
#96755=COLOUR_RGB ( '', 0.40784314, 0.44705882, 0.49803922) ;
#96757=DIRECTION ( 'NONE',  ( -0.000000000000000000, -0.000000000000000000, 1.000000000000000000 ) ) ;
#96762=ORIENTED_EDGE ( 'NONE', *, *, #39416, .F. ) ;
#96763=FACE_OUTER_BOUND ( 'NONE', #56122, .T. ) ;
#96772=FACE_OUTER_BOUND ( 'NONE', #9269, .T. ) ;
#96776=PRESENTATION_STYLE_ASSIGNMENT (( #73252 ) ) ;
#96777=CYLINDRICAL_SURFACE ( 'NONE', #35406, 0.2499999999999997780 ) ;
#96782=EDGE_CURVE ( 'NONE', #95488, #13782, #54332, .T. ) ;
#96786=CARTESIAN_POINT ( 'NONE',  ( -8.000000000000000000, 80.99999999999994316, 0.000000000000000000 ) ) ;
#96787=SURFACE_STYLE_FILL_AREA ( #20773 ) ;
#96808=AXIS2_PLACEMENT_3D ( 'NONE', #73110, #73607, #35112 ) ;
#96812=( NAMED_UNIT ( * ) PLANE_ANGLE_UNIT ( ) SI_UNIT ( $, .RADIAN. ) );
#96830=ORIENTED_EDGE ( 'NONE', *, *, #15869, .F. ) ;
#96833=ADVANCED_FACE ( 'NONE', ( #54822 ), #51855, .T. ) ;
#96837=VECTOR ( 'NONE', #34816, 1000.000000000000114 ) ;
#96841=AXIS2_PLACEMENT_3D ( 'NONE', #93275, #86276, #10279 ) ;
#96842=ORIENTED_EDGE ( 'NONE', *, *, #2891, .F. ) ;
#96845=ORIENTED_EDGE ( 'NONE', *, *, #6639, .F. ) ;
#96855=MECHANICAL_DESIGN_GEOMETRIC_PRESENTATION_REPRESENTATION('',(#80921),#42594);
#96859=CARTESIAN_POINT ( 'NONE',  ( 17.75000000000000000, 84.07179676972448590, -3.750000000000000000 ) ) ;
#96867=CARTESIAN_POINT ( 'NONE',  ( -13.78553237914111129, 90.91070185254878311, -7.842545424067505877 ) ) ;
#96872=AXIS2_PLACEMENT_3D ( 'NONE', #26976, #87968, #34466 ) ;
#96897=DIRECTION ( 'NONE',  ( 1.000000000000000000, 1.257402221000611116E-16, -0.000000000000000000 ) ) ;
#96903=CARTESIAN_POINT ( 'NONE',  ( -9.347645168806021587, 88.42200471242378512, 5.276767730577756055 ) ) ;
#96905=B_SPLINE_SURFACE_WITH_KNOTS ( 'NONE', 3, 1, ( 
 ( #5139, #13122 ),
 ( #43618, #90593 ),
 ( #59606, #28620 ),
 ( #82607, #35630 ),
 ( #67620, #98128 ),
 ( #60091, #22120 ),
 ( #52600, #14631 ),
 ( #20129, #50633 ),
 ( #38598, #133 ),
 ( #78066, #68605 ),
 ( #69096, #62555 ),
 ( #60595, #47063 ),
 ( #31568, #54562 ),
 ( #62064, #76094 ),
 ( #76582, #61574 ),
 ( #53585, #32052 ),
 ( #38116, #39590 ),
 ( #46098, #8102 ) ),
 .UNSPECIFIED., .F., .F., .F.,
 ( 4, 2, 2, 2, 2, 2, 2, 2, 4 ),
 ( 2, 2 ),
 ( 0.000000000000000000, 0.06249999999999988898, 0.1249999999999998890, 0.2499999999999997780, 0.4999999999999994449, 0.5624999999999994449, 0.6249999999999994449, 0.7499999999999995559, 0.8570805329376184334 ),
 ( 0.000000000000000000, 1.000000000000000000 ),
 .UNSPECIFIED. ) ;
#96915=ADVANCED_FACE ( 'NONE', ( #56797 ), #95794, .F. ) ;
#96916=DIRECTION ( 'NONE',  ( -2.569960705150826877E-16, 1.000000000000000000, 0.000000000000000000 ) ) ;
#96921=CARTESIAN_POINT ( 'NONE',  ( -7.750000000000000000, 1.019547802438466100, 3.750000000000000000 ) ) ;
#96932=CIRCLE ( 'NONE', #71374, 6.349999999999995204 ) ;
#96957=CARTESIAN_POINT ( 'NONE',  ( 4.380000000000000782, 1.019547802438464545, 3.750000000000000000 ) ) ;
#96958=CARTESIAN_POINT ( 'NONE',  ( 3.969999999999999751, 10.00000000000000000, 3.750000000000000000 ) ) ;
#96960=CARTESIAN_POINT ( 'NONE',  ( 14.99999999999997868, 80.07179676972448590, -6.250000000000000000 ) ) ;
#96993=CARTESIAN_POINT ( 'NONE',  ( -5.780406540405962801, -39.80436905996668884, 2.500000000000000000 ) ) ;
#96995=AXIS2_PLACEMENT_3D ( 'NONE', #33370, #3391, #33854 ) ;
#96998=CIRCLE ( 'NONE', #84217, 0.2500000000000002220 ) ;
#96999=EDGE_CURVE ( 'NONE', #96102, #97731, #46916, .T. ) ;
#97000=CARTESIAN_POINT ( 'NONE',  ( 6.825220758711185276, -50.90060425938852973, 3.999999999999999112 ) ) ;
#97011=CARTESIAN_POINT ( 'NONE',  ( 6.903457398626329677, -84.61157762779829739, -3.750000000000000888 ) ) ;
#97020=CARTESIAN_POINT ( 'NONE',  ( 18.00000000000000355, 77.62863619046393637, 4.012044713968255572 ) ) ;
#97036=ADVANCED_FACE ( 'NONE', ( #47722 ), #8738, .F. ) ;
#97045=MECHANICAL_DESIGN_GEOMETRIC_PRESENTATION_REPRESENTATION('',(#71482),#63471);
#97049=VECTOR ( 'NONE', #60526, 1000.000000000000000 ) ;
#97073=CARTESIAN_POINT ( 'NONE',  ( 10.88969086829045452, -97.65447219785596644, -3.750000000000000000 ) ) ;
#97074=CARTESIAN_POINT ( 'NONE',  ( -4.262581423003710235, -13.85606188143285600, -3.750000000000000444 ) ) ;
#97081=CYLINDRICAL_SURFACE ( 'NONE', #33197, 0.2500000000000002220 ) ;
#97086=DIRECTION ( 'NONE',  ( -0.06975647374410356982, -0.9975640502598257520, -0.000000000000000000 ) ) ;
#97089=DIRECTION ( 'NONE',  ( 1.000000000000000000, 0.000000000000000000, 0.000000000000000000 ) ) ;
#97092=ORIENTED_EDGE ( 'NONE', *, *, #98665, .T. ) ;
#97104=ORIENTED_EDGE ( 'NONE', *, *, #78101, .T. ) ;
#97118=EDGE_CURVE ( 'NONE', #50286, #56730, #84749, .T. ) ;
#97123=EDGE_CURVE ( 'NONE', #55759, #76829, #70738, .T. ) ;
#97128=CARTESIAN_POINT ( 'NONE',  ( -3.585811805803780672, -2.700665136322976334, 3.750000000000000000 ) ) ;
#97129=CARTESIAN_POINT ( 'NONE',  ( -3.750000000000000000, 37.25000000000000000, 4.000000000000000000 ) ) ;
#97154=PRODUCT_DEFINITION_SHAPE ( 'NONE', 'NONE',  #56260 ) ;
#97160=CARTESIAN_POINT ( 'NONE',  ( -11.20030343312800980, -94.46585862447406612, -4.000000000000451195 ) ) ;
#97169=UNCERTAINTY_MEASURE_WITH_UNIT (LENGTH_MEASURE( 1.000000000000000082E-05 ), #12114, 'distance_accuracy_value', 'NONE');
#97188=ORIENTED_EDGE ( 'NONE', *, *, #45616, .F. ) ;
#97197=CARTESIAN_POINT ( 'NONE',  ( -10.53011945866295029, -98.59345040283277228, 4.000000000000000000 ) ) ;
#97214=EDGE_CURVE ( 'NONE', #74673, #89322, #54906, .T. ) ;
#97217=MECHANICAL_DESIGN_GEOMETRIC_PRESENTATION_REPRESENTATION('',(#4624),#30153);
#97223=B_SPLINE_CURVE_WITH_KNOTS ( 'NONE', 3,
 ( #72868, #50870, #82343, #81847, #20870, #81362, #12861, #73857, #5387, #44343, #28365, #28841, #58853, #89359, #74849, #59344, #89846, #6350 ),
 .UNSPECIFIED., .F., .F.,
 ( 4, 2, 2, 2, 2, 2, 2, 2, 4 ),
 ( 0.000000000000000000, 0.001337396791554949218, 0.002674793583109898436, 0.004012190374664847438, 0.005349587166219796873, 0.006686983957774746308, 0.008024380749329694876, 0.009361777540884644311, 0.01069917433243959375 ),
 .UNSPECIFIED. ) ;
#97225=VERTEX_POINT ( 'NONE', #93215 ) ;
#97235=CARTESIAN_POINT ( 'NONE',  ( 8.629999999999995453, 40.74999999999999289, -4.000000000000000000 ) ) ;
#97242=CARTESIAN_POINT ( 'NONE',  ( 4.629999999999990123, 76.07179676972444327, 4.250000000000000000 ) ) ;
#97243=ORIENTED_EDGE ( 'NONE', *, *, #79727, .T. ) ;
#97259=ORIENTED_EDGE ( 'NONE', *, *, #36318, .F. ) ;
#97265=AXIS2_PLACEMENT_3D ( 'NONE', #61743, #92262, #22302 ) ;
#97275=COLOUR_RGB ( '', 0.40784314, 0.44705882, 0.49803922) ;
#97281=DIRECTION ( 'NONE',  ( -2.569960705150826877E-16, 1.000000000000000000, -0.000000000000000000 ) ) ;
#97295=FILL_AREA_STYLE_COLOUR ( '', #84886 ) ;
#97304=SURFACE_STYLE_FILL_AREA ( #19312 ) ;
#97317=ORIENTED_EDGE ( 'NONE', *, *, #69112, .T. ) ;
#97322=ORIENTED_EDGE ( 'NONE', *, *, #14142, .T. ) ;
#97340=LINE ( 'NONE', #6814, #92550 ) ;
#97343=ORIENTED_EDGE ( 'NONE', *, *, #15169, .T. ) ;
#97363=VERTEX_POINT ( 'NONE', #64181 ) ;
#97364=DIRECTION ( 'NONE',  ( 1.000000000000000000, 0.000000000000000000, 0.000000000000000000 ) ) ;
#97365=( NAMED_UNIT ( * ) SI_UNIT ( $, .STERADIAN. ) SOLID_ANGLE_UNIT ( ) );
#97371=CYLINDRICAL_SURFACE ( 'NONE', #39230, 0.2500000000000002220 ) ;
#97379=EDGE_CURVE ( 'NONE', #55236, #5883, #80180, .T. ) ;
#97386=DIRECTION ( 'NONE',  ( 1.000000000000000000, 0.000000000000000000, 0.000000000000000000 ) ) ;
#97390=DIRECTION ( 'NONE',  ( 0.000000000000000000, -0.000000000000000000, -1.000000000000000000 ) ) ;
#97393=CARTESIAN_POINT ( 'NONE',  ( -7.037799269744632547, -86.25965645050756336, -2.499999999999194422 ) ) ;
#97400=ORIENTED_EDGE ( 'NONE', *, *, #58025, .T. ) ;
#97403=CARTESIAN_POINT ( 'NONE',  ( -9.823941624389807004, -32.16601312911085842, -3.999999999999999112 ) ) ;
#97417=UNCERTAINTY_MEASURE_WITH_UNIT (LENGTH_MEASURE( 1.000000000000000082E-05 ), #23265, 'distance_accuracy_value', 'NONE');
#97425=DIRECTION ( 'NONE',  ( -1.000000000000000000, 0.000000000000000000, 0.000000000000000000 ) ) ;
#97430=VECTOR ( 'NONE', #66265, 1000.000000000000000 ) ;
#97444=CARTESIAN_POINT ( 'NONE',  ( 4.380000001274070520, 0.08775168531748565870, 4.000000000000000000 ) ) ;
#97445=FILL_AREA_STYLE ('',( #4384 ) ) ;
#97468=ORIENTED_EDGE ( 'NONE', *, *, #68437, .F. ) ;
#97473=EDGE_CURVE ( 'NONE', #93536, #56519, #96187, .T. ) ;
#97474=ORIENTED_EDGE ( 'NONE', *, *, #53534, .T. ) ;
#97483=LINE ( 'NONE', #58969, #30754 ) ;
#97484=CARTESIAN_POINT ( 'NONE',  ( 11.35644480889443386, -65.08008077083093212, 3.750000000000000000 ) ) ;
#97486=ORIENTED_EDGE ( 'NONE', *, *, #5168, .F. ) ;
#97489=PLANE ( 'NONE',  #39023 ) ;
#97493=TOROIDAL_SURFACE ( 'NONE', #9684, 10.09999999999999787, 0.1000000000000000056 ) ;
#97503=CARTESIAN_POINT ( 'NONE',  ( 6.829574850499570360, -88.00372650123708240, -2.750000000000000000 ) ) ;
#97511=CARTESIAN_POINT ( 'NONE',  ( 18.00000000000000355, 77.07179676972445748, 4.250000000000000000 ) ) ;
#97536=( GEOMETRIC_REPRESENTATION_CONTEXT ( 3 ) GLOBAL_UNCERTAINTY_ASSIGNED_CONTEXT ( ( #78455 ) ) GLOBAL_UNIT_ASSIGNED_CONTEXT ( ( #74105, #12625, #82108 ) ) REPRESENTATION_CONTEXT ( 'NONE', 'WORKASPACE' ) );
#97549=EDGE_LOOP ( 'NONE', ( #88073, #62118, #62223 ) ) ;
#97564=ORIENTED_EDGE ( 'NONE', *, *, #72137, .F. ) ;
#97577=CARTESIAN_POINT ( 'NONE',  ( -15.00000000000000000, 83.99999999999998579, 7.750000000000000000 ) ) ;
#97608=TOROIDAL_SURFACE ( 'NONE', #33678, 7.250000000000002665, 0.2500000000000000000 ) ;
#97609=CIRCLE ( 'NONE', #41775, 0.09999999999999982514 ) ;
#97612=CARTESIAN_POINT ( 'NONE',  ( 10.09974179616572521, -32.02510747888860010, 4.000000000000000000 ) ) ;
#97619=DIRECTION ( 'NONE',  ( 0.000000000000000000, 0.000000000000000000, -1.000000000000000000 ) ) ;
#97631=CYLINDRICAL_SURFACE ( 'NONE', #70715, 1.249999999999987121 ) ;
#97641=FACE_OUTER_BOUND ( 'NONE', #33335, .T. ) ;
#97661=ORIENTED_EDGE ( 'NONE', *, *, #4652, .T. ) ;
#97675=CARTESIAN_POINT ( 'NONE',  ( -6.349999999999995204, -97.00000000000000000, 4.000000000000000000 ) ) ;
#97679=ORIENTED_EDGE ( 'NONE', *, *, #56725, .T. ) ;
#97680=FILL_AREA_STYLE_COLOUR ( '', #15053 ) ;
#97693=DIRECTION ( 'NONE',  ( -0.000000000000000000, -0.000000000000000000, -1.000000000000000000 ) ) ;
#97698=CARTESIAN_POINT ( 'NONE',  ( -3.750000000000000888, 1.019547802438453887, -3.750000000000000000 ) ) ;
#97700=EDGE_LOOP ( 'NONE', ( #33200, #81785 ) ) ;
#97701=CARTESIAN_POINT ( 'NONE',  ( -7.232415441807423129, -88.12698951299773853, 4.000000000000000000 ) ) ;
#97706=CARTESIAN_POINT ( 'NONE',  ( 8.879999999999991900, 20.99999999999999645, 1.249999999999987121 ) ) ;
#97708=AXIS2_PLACEMENT_3D ( 'NONE', #86079, #55582, #10081 ) ;
#97716=ADVANCED_FACE ( 'NONE', ( #20675 ), #18248, .T. ) ;
#97731=VERTEX_POINT ( 'NONE', #28168 ) ;
#97734=SURFACE_SIDE_STYLE ('',( #60680 ) ) ;
#97737=DIRECTION ( 'NONE',  ( -1.000000000000000000, 0.000000000000000000, 0.000000000000000000 ) ) ;
#97745=SURFACE_STYLE_USAGE ( .BOTH. , #66217 ) ;
#97747=DIRECTION ( 'NONE',  ( 0.000000000000000000, 0.000000000000000000, 1.000000000000000000 ) ) ;
#97753=ORIENTED_EDGE ( 'NONE', *, *, #26485, .T. ) ;
#97766=CARTESIAN_POINT ( 'NONE',  ( -7.750000000000000000, 40.74999999999999289, 4.250000000000000000 ) ) ;
#97772=EDGE_CURVE ( 'NONE', #16059, #33129, #86530, .T. ) ;
#97777=ORIENTED_EDGE ( 'NONE', *, *, #87049, .F. ) ;
#97782=CARTESIAN_POINT ( 'NONE',  ( -10.28286150160603363, 89.18763609516977908, -5.839555419999089558 ) ) ;
#97785=VECTOR ( 'NONE', #94637, 1000.000000000000000 ) ;
#97792=CARTESIAN_POINT ( 'NONE',  ( 9.511402282428090160, -15.49422404099892248, -4.000000000000000000 ) ) ;
#97802=AXIS2_PLACEMENT_3D ( 'NONE', #67000, #22997, #60964 ) ;
#97821=CARTESIAN_POINT ( 'NONE',  ( -3.772435416983038525, -6.430908609849964819, 4.000000000001613820 ) ) ;
#97835=EDGE_CURVE ( 'NONE', #76829, #70343, #42229, .T. ) ;
#97846=DIRECTION ( 'NONE',  ( 0.6246950475544238435, 0.7808688094430307203, 0.000000000000000000 ) ) ;
#97849=COLOUR_RGB ( '', 0.31764706, 0.68627451, 0.89019608) ;
#97853=AXIS2_PLACEMENT_3D ( 'NONE', #14884, #9326, #98889 ) ;
#97871=CARTESIAN_POINT ( 'NONE',  ( 6.910443788319881264, -84.29081344359276784, -2.499999999992758681 ) ) ;
#97887=CARTESIAN_POINT ( 'NONE',  ( -18.89999999999999503, 92.00000000000000000, -7.750000000000000000 ) ) ;
#97899=CARTESIAN_POINT ( 'NONE',  ( -7.121341127193570486, -73.24353698637885657, -2.750000000000000000 ) ) ;
#97906=EDGE_LOOP ( 'NONE', ( #51189, #68640, #2172, #67931, #41059, #62047, #51030, #17067, #17276, #10950, #63112, #69461, #84369, #93865, #24256, #36689, #53891, #56620, #89008, #59301, #66805, #60855, #65663, #46392, #63854, #19714, #1894, #38073, #83085, #2467 ) ) ;
#97917=DIRECTION ( 'NONE',  ( 1.000000000000000000, 0.000000000000000000, 0.000000000000000000 ) ) ;
#97943=EDGE_LOOP ( 'NONE', ( #52073, #71135, #55675, #57517 ) ) ;
#97966=EDGE_CURVE ( 'NONE', #6107, #40043, #48559, .T. ) ;
#97974=EDGE_LOOP ( 'NONE', ( #76064, #7279, #82330, #47642 ) ) ;
#97979=DIRECTION ( 'NONE',  ( 1.000000000000000000, 0.000000000000000000, 0.000000000000000000 ) ) ;
#97989=AXIS2_PLACEMENT_3D ( 'NONE', #17347, #2354, #8842 ) ;
#97991=AXIS2_PLACEMENT_3D ( 'NONE', #15212, #68209, #62148 ) ;
#97993=COLOUR_RGB ( '', 0.31764706, 0.68627451, 0.89019608) ;
#98002=COLOUR_RGB ( '', 0.08235294, 0.09019608, 0.10196078) ;
#98040=CARTESIAN_POINT ( 'NONE',  ( 8.630000000000000782, 1.019547802438459216, 3.750000000000000000 ) ) ;
#98043=ORIENTED_EDGE ( 'NONE', *, *, #31392, .F. ) ;
#98045=EDGE_CURVE ( 'NONE', #57827, #96234, #57490, .T. ) ;
#98049=CARTESIAN_POINT ( 'NONE',  ( -6.000000000000000000, 78.07179676972447169, -4.000000000000000000 ) ) ;
#98055=CARTESIAN_POINT ( 'NONE',  ( 10.72255383998327005, -40.29605683832149765, -3.750000000000002220 ) ) ;
#98056=CARTESIAN_POINT ( 'NONE',  ( -6.060988839905886216, -36.09899559454662210, -4.000000000000000000 ) ) ;
#98069=CIRCLE ( 'NONE', #27802, 0.2500000000000002220 ) ;
#98105=CARTESIAN_POINT ( 'NONE',  ( -7.750000000000000000, 41.24999999999999289, -6.500000000000000888 ) ) ;
#98128=CARTESIAN_POINT ( 'NONE',  ( -3.711005778769052021, -5.293034685380286319, -3.750000000000000000 ) ) ;
#98130=AXIS2_PLACEMENT_3D ( 'NONE', #29106, #21631, #52117 ) ;
#98138=( NAMED_UNIT ( * ) PLANE_ANGLE_UNIT ( ) SI_UNIT ( $, .RADIAN. ) );
#98142=CARTESIAN_POINT ( 'NONE',  ( 11.34661744925197624, 54.08985607419764818, -3.000000000000000000 ) ) ;
#98167=ORIENTED_EDGE ( 'NONE', *, *, #20667, .T. ) ;
#98179=CARTESIAN_POINT ( 'NONE',  ( -7.778993154286912848, -1.060766117536017017, 4.000000000000000000 ) ) ;
#98185=SURFACE_SIDE_STYLE ('',( #13178 ) ) ;
#98192=DIRECTION ( 'NONE',  ( 0.000000000000000000, -1.000000000000000000, 0.000000000000000000 ) ) ;
#98216=DIRECTION ( 'NONE',  ( 0.000000000000000000, 0.000000000000000000, -1.000000000000000000 ) ) ;
#98226=CARTESIAN_POINT ( 'NONE',  ( 8.629999999999995453, 41.24999999999999289, -4.250000000000000000 ) ) ;
#98234=DIRECTION ( 'NONE',  ( 0.000000000000000000, -1.000000000000000000, 0.000000000000000000 ) ) ;
#98235=( NAMED_UNIT ( * ) SI_UNIT ( $, .STERADIAN. ) SOLID_ANGLE_UNIT ( ) );
#98237=ADVANCED_FACE ( 'NONE', ( #19984 ), #97489, .F. ) ;
#98245=EDGE_CURVE ( 'NONE', #5309, #14873, #34710, .T. ) ;
#98248=EDGE_CURVE ( 'NONE', #10214, #48471, #43955, .T. ) ;
#98264=CARTESIAN_POINT ( 'NONE',  ( -8.000000000000000000, 1.019547802438458550, 3.750000000000000000 ) ) ;
#98277=PRESENTATION_STYLE_ASSIGNMENT (( #21772 ) ) ;
#98278=CARTESIAN_POINT ( 'NONE',  ( -8.099999999999999645, 75.73428692542562146, -2.900000000000000355 ) ) ;
#98286=CARTESIAN_POINT ( 'NONE',  ( 10.09973302567988362, -32.02492402194155119, -4.000000000000000000 ) ) ;
#98290=CARTESIAN_POINT ( 'NONE',  ( 4.219999999999999751, 10.25000000000000000, -3.750000000000000000 ) ) ;
#98298=UNCERTAINTY_MEASURE_WITH_UNIT (LENGTH_MEASURE( 1.000000000000000082E-05 ), #1384, 'distance_accuracy_value', 'NONE');
#98301=CIRCLE ( 'NONE', #61502, 0.2500000000000002220 ) ;
#98317=ORIENTED_EDGE ( 'NONE', *, *, #69290, .T. ) ;
#98319=VERTEX_POINT ( 'NONE', #76927 ) ;
#98324=ORIENTED_EDGE ( 'NONE', *, *, #11977, .F. ) ;
#98330=VERTEX_POINT ( 'NONE', #46433 ) ;
#98334=SURFACE_SIDE_STYLE ('',( #31268 ) ) ;
#98336=DIRECTION ( 'NONE',  ( -1.000000000000000000, -2.107602052970794797E-16, 0.000000000000000000 ) ) ;
#98355=DIRECTION ( 'NONE',  ( -1.000000000000000000, -1.257402221000612102E-16, 0.000000000000000000 ) ) ;
#98365=EDGE_CURVE ( 'NONE', #95619, #31275, #35789, .T. ) ;
#98367=CARTESIAN_POINT ( 'NONE',  ( 4.572805491839753600, -6.390838093316509649, -2.500000000000000000 ) ) ;
#98378=DIRECTION ( 'NONE',  ( 0.9975640502598243087, -0.06975647374412544122, -0.000000000000000000 ) ) ;
#98390=DIRECTION ( 'NONE',  ( -0.000000000000000000, 0.000000000000000000, 1.000000000000000000 ) ) ;
#98416=VECTOR ( 'NONE', #17914, 1000.000000000000000 ) ;
#98417=UNCERTAINTY_MEASURE_WITH_UNIT (LENGTH_MEASURE( 1.000000000000000082E-05 ), #12541, 'distance_accuracy_value', 'NONE');
#98437=DIRECTION ( 'NONE',  ( 1.000000000000000000, 0.000000000000000000, 0.000000000000000000 ) ) ;
#98442=SURFACE_STYLE_FILL_AREA ( #28430 ) ;
#98449=DIRECTION ( 'NONE',  ( -0.9975640502598257520, 0.06975647374410356982, 0.000000000000000000 ) ) ;
#98457=LINE ( 'NONE', #29913, #5202 ) ;
#98469=AXIS2_PLACEMENT_3D ( 'NONE', #90396, #21935, #52415 ) ;
#98471=ORIENTED_EDGE ( 'NONE', *, *, #89157, .T. ) ;
#98477=CARTESIAN_POINT ( 'NONE',  ( -7.037799270021981357, -86.25965645051654462, 2.749999999998387956 ) ) ;
#98481=CARTESIAN_POINT ( 'NONE',  ( 7.160365893312771846, -84.29711206764778808, -4.000000000000000000 ) ) ;
#98485=DIRECTION ( 'NONE',  ( 1.000000000000000000, -0.000000000000000000, -0.000000000000000000 ) ) ;
#98490=( BOUNDED_CURVE ( )  B_SPLINE_CURVE ( 3, ( #41545, #72009, #80006, #87997 ),
 .UNSPECIFIED., .F., .F. ) 
 B_SPLINE_CURVE_WITH_KNOTS ( ( 4, 4 ),
 ( 0.000000000000000000, 1.570796326794896558 ),
 .UNSPECIFIED. ) 
 CURVE ( )  GEOMETRIC_REPRESENTATION_ITEM ( )  RATIONAL_B_SPLINE_CURVE ( ( 1.000000000000000000, 0.8047378541243649375, 0.8047378541243649375, 1.000000000000000000 ) ) 
 REPRESENTATION_ITEM ( '' )  );
#98511=AXIS2_PLACEMENT_3D ( 'NONE', #78652, #710, #47657 ) ;
#98524=CARTESIAN_POINT ( 'NONE',  ( 8.629999999999995453, 41.24999999999999289, -6.250000000000000000 ) ) ;
#98539=AXIS2_PLACEMENT_3D ( 'NONE', #49119, #19111, #49591 ) ;
#98568=CARTESIAN_POINT ( 'NONE',  ( -13.80105244024794331, 90.89655890636515778, -7.750000000004162892 ) ) ;
#98581=ORIENTED_EDGE ( 'NONE', *, *, #84783, .F. ) ;
#98607=ORIENTED_EDGE ( 'NONE', *, *, #36807, .F. ) ;
#98608=EDGE_CURVE ( 'NONE', #17079, #75926, #22465, .T. ) ;
#98612=( NAMED_UNIT ( * ) PLANE_ANGLE_UNIT ( ) SI_UNIT ( $, .RADIAN. ) );
#98613=COLOUR_RGB ( '', 0.40784314, 0.44705882, 0.49803922) ;
#98614=ADVANCED_FACE ( 'NONE', ( #52941 ), #53341, .T. ) ;
#98630=EDGE_LOOP ( 'NONE', ( #2746, #28530, #21422, #81010 ) ) ;
#98647=CARTESIAN_POINT ( 'NONE',  ( 11.34661744925197624, 54.08985607419764818, 0.000000000000000000 ) ) ;
#98652=AXIS2_PLACEMENT_3D ( 'NONE', #34356, #57361, #19375 ) ;
#98665=EDGE_CURVE ( 'NONE', #87189, #61498, #29423, .T. ) ;
#98673=CARTESIAN_POINT ( 'NONE',  ( 5.783708210301603536, -36.05554043948455245, 2.500000000000000000 ) ) ;
#98682=CARTESIAN_POINT ( 'NONE',  ( -8.000000002517667852, -0.01653120533954156174, 4.000000000000000000 ) ) ;
#98694=CARTESIAN_POINT ( 'NONE',  ( 3.969999999999999751, 10.00000000000000000, -2.750000000000000000 ) ) ;
#98701=CYLINDRICAL_SURFACE ( 'NONE', #69453, 0.2500000000000002220 ) ;
#98705=EDGE_CURVE ( 'NONE', #21472, #81788, #77909, .T. ) ;
#98717=PLANE ( 'NONE',  #44733 ) ;
#98720=AXIS2_PLACEMENT_3D ( 'NONE', #71579, #11063, #3090 ) ;
#98723=EDGE_LOOP ( 'NONE', ( #38432, #73846, #73417, #55240 ) ) ;
#98724=ADVANCED_FACE ( 'NONE', ( #18399 ), #78897, .T. ) ;
#98726=DIRECTION ( 'NONE',  ( 1.000000000000000000, 0.000000000000000000, 0.000000000000000000 ) ) ;
#98730=DIRECTION ( 'NONE',  ( 0.8070303256584299145, -0.5905099943842175847, 0.000000000000000000 ) ) ;
#98735=DIRECTION ( 'NONE',  ( -0.000000000000000000, -0.000000000000000000, 1.000000000000000000 ) ) ;
#98751=CARTESIAN_POINT ( 'NONE',  ( 5.129999999999995453, 43.00000000000000711, 6.250000000000000000 ) ) ;
#98770=AXIS2_PLACEMENT_3D ( 'NONE', #23541, #77008, #8033 ) ;
#98779=DIRECTION ( 'NONE',  ( 0.000000000000000000, 0.000000000000000000, 1.000000000000000000 ) ) ;
#98784=CARTESIAN_POINT ( 'NONE',  ( 11.43665875895689332, -81.61983315981103715, -4.000000000003584688 ) ) ;
#98785=CARTESIAN_POINT ( 'NONE',  ( 3.969999999999999751, 37.00000000000000000, 2.750000000000000000 ) ) ;
#98790=SURFACE_STYLE_FILL_AREA ( #3097 ) ;
#98811=CARTESIAN_POINT ( 'NONE',  ( 6.324651560460970323, -50.88858560564519706, -2.500000000000001776 ) ) ;
#98817=EDGE_LOOP ( 'NONE', ( #79614, #16729, #40740, #15802, #9680 ) ) ;
#98822=ORIENTED_EDGE ( 'NONE', *, *, #78485, .T. ) ;
#98824=ADVANCED_FACE ( 'NONE', ( #34364 ), #64532, .T. ) ;
#98832=DIRECTION ( 'NONE',  ( 0.9961946980917458783, -0.08715574274765407192, 0.000000000000000000 ) ) ;
#98835=EDGE_LOOP ( 'NONE', ( #56136, #14309, #93867, #44161, #68052 ) ) ;
#98844=AXIS2_PLACEMENT_3D ( 'NONE', #12905, #43401, #64419 ) ;
#98854=CARTESIAN_POINT ( 'NONE',  ( 3.969999999999999751, 36.75000000000000000, 4.000000000000000000 ) ) ;
#98863=CARTESIAN_POINT ( 'NONE',  ( 4.380000000000000782, 1.019547802438464545, -2.750000000000000000 ) ) ;
#98866=EDGE_LOOP ( 'NONE', ( #59643, #93950, #49816, #5567 ) ) ;
#98878=DIRECTION ( 'NONE',  ( -0.000000000000000000, 0.000000000000000000, 1.000000000000000000 ) ) ;
#98882=CARTESIAN_POINT ( 'NONE',  ( -11.16008302860135259, -52.90628376244837483, -3.749999999998196998 ) ) ;
#98889=DIRECTION ( 'NONE',  ( 0.5901017155109145040, 0.8073289077885640319, 0.000000000000000000 ) ) ;
#98904=( LENGTH_UNIT ( ) NAMED_UNIT ( * ) SI_UNIT ( .MILLI., .METRE. ) );
#98922=( GEOMETRIC_REPRESENTATION_CONTEXT ( 3 ) GLOBAL_UNCERTAINTY_ASSIGNED_CONTEXT ( ( #77214 ) ) GLOBAL_UNIT_ASSIGNED_CONTEXT ( ( #52287, #75775, #37795 ) ) REPRESENTATION_CONTEXT ( 'NONE', 'WORKASPACE' ) );
#98927=B_SPLINE_CURVE_WITH_KNOTS ( 'NONE', 3,
 ( #29903, #22929, #53397, #77373, #38909, #62367, #83906, #45914, #31381, #15435, #69396, #918, #16895, #91400, #70389, #54871, #76403, #53903, #7918, #68419, #15909, #77870 ),
 .UNSPECIFIED., .F., .F.,
 ( 4, 2, 2, 2, 2, 2, 2, 2, 2, 2, 4 ),
 ( 0.000000000000000000, 0.002789117597787886711, 0.005578235195575773422, 0.01115647039115154684, 0.02231294078230309369, 0.03346941117345463707, 0.04462588156460618738, 0.06693882234690927413, 0.07809529273806081751, 0.08367352793363661001, 0.08925176312921238864 ),
 .UNSPECIFIED. ) ;
#98937=CARTESIAN_POINT ( 'NONE',  ( 7.079515573063597245, -88.00917032380698402, 4.000000000000000000 ) ) ;
#98941=ADVANCED_FACE ( 'NONE', ( #74838 ), #3973, .T. ) ;
#98946=EDGE_LOOP ( 'NONE', ( #84788, #43588, #78150, #48565 ) ) ;
#98957=B_SPLINE_CURVE_WITH_KNOTS ( 'NONE', 3,
 ( #86579, #94560, #56085, #87063, #96051, #25593, #79570, #56572, #95553, #10092, #3096, #80049, #94072, #95045, #86088, #42073, #4068, #50046, #18087, #64047, #12046, #63564 ),
 .UNSPECIFIED., .F., .F.,
 ( 4, 2, 2, 2, 2, 2, 2, 2, 2, 2, 4 ),
 ( 0.000000000000000000, 0.005577058014692720320, 0.01115411602938544064, 0.02230823205877083618, 0.04461646411754159602, 0.05577058014692697074, 0.06692469617631234546, 0.07807881220569773406, 0.08365587022039042142, 0.08644439922773676510, 0.08923292823508310878 ),
 .UNSPECIFIED. ) ;
#98959=CARTESIAN_POINT ( 'NONE',  ( 6.880000000000009663, 40.99999999999999289, 4.250000000000000000 ) ) ;
#98964=CARTESIAN_POINT ( 'NONE',  ( 9.879999999999984794, 27.00000000000000711, 2.958578643762690419 ) ) ;
#98979=ORIENTED_EDGE ( 'NONE', *, *, #599, .T. ) ;
#98981=CARTESIAN_POINT ( 'NONE',  ( 1.379999999999981908, 20.99999999999999645, 0.000000000000000000 ) ) ;
ENDSEC;
END-ISO-10303-21;
